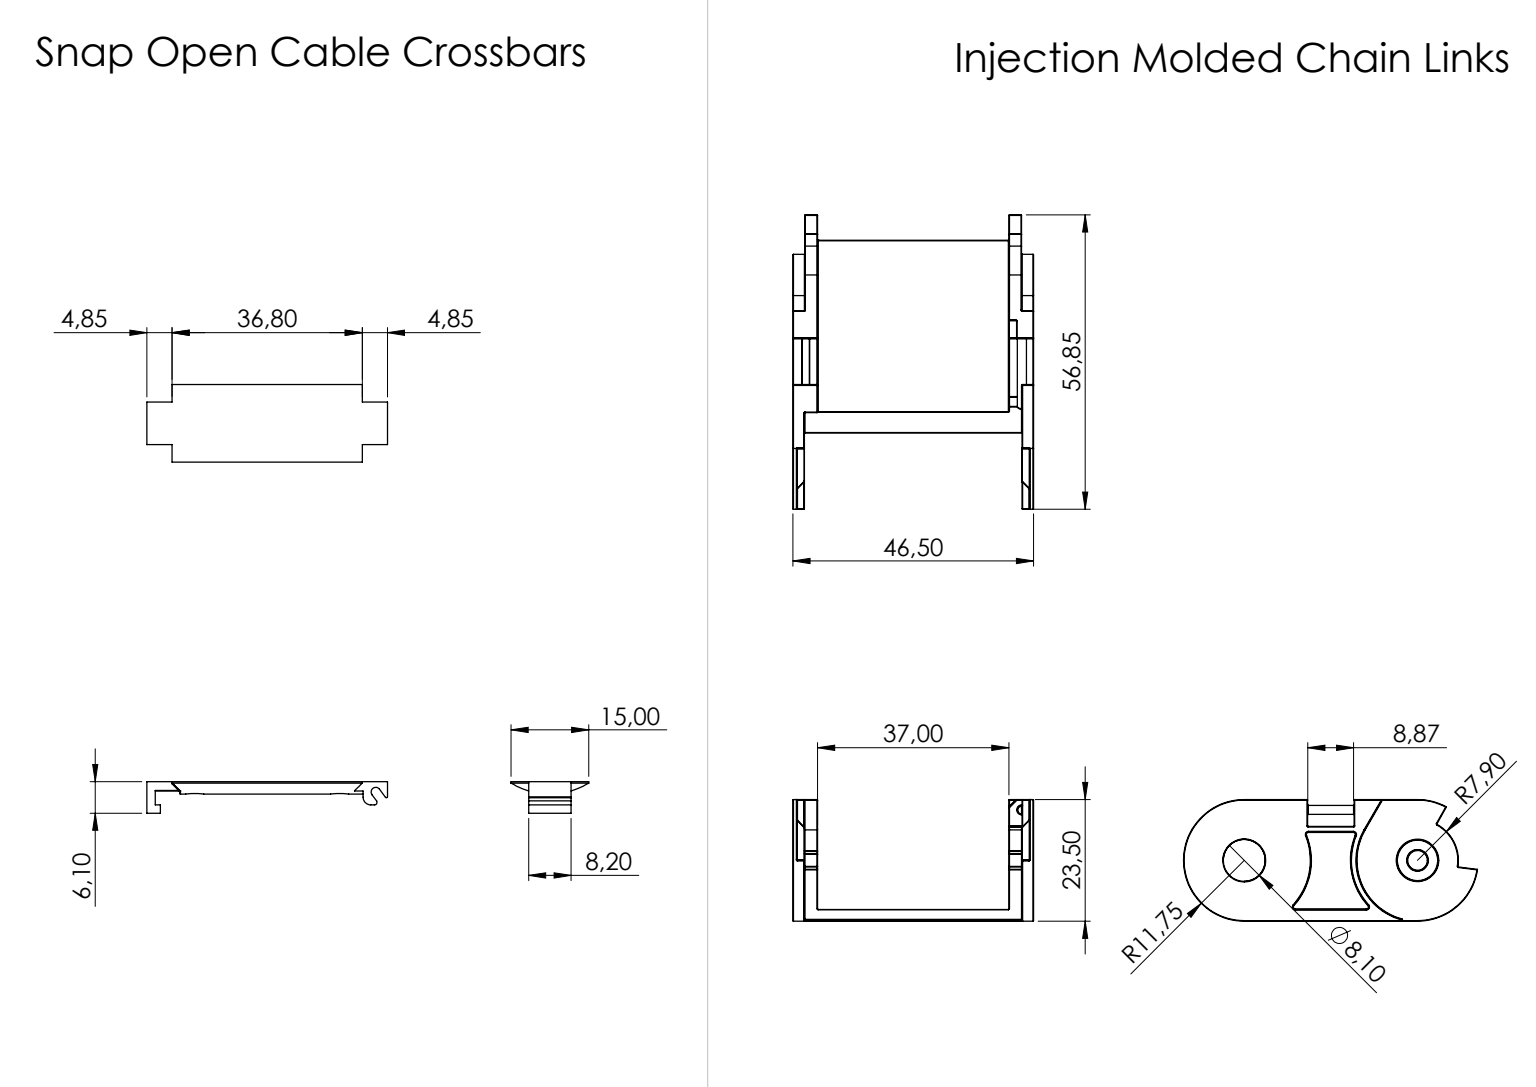
ISO-10303-21;
HEADER;
FILE_DESCRIPTION (('STEP AP214'),
    '1' );
FILE_NAME ('Injection Molded Chain Links.step',
    '2026-10-08T22:59:04',
    ( '' ),
    ( '' ),
    'SwSTEP 2.0',
    'SolidWorks 2020',
    '' );
FILE_SCHEMA (( 'AUTOMOTIVE_DESIGN' ));
ENDSEC;

DATA;
#14=ORIENTED_EDGE ( 'NONE', *, *, #107088, .T. ) ;
#39=LINE ( 'NONE', #62597, #48246 ) ;
#42=CARTESIAN_POINT ( 'NONE',  ( -20.94999999999999929, 0.000000000000000000, -7.900000000000000355 ) ) ;
#67=CARTESIAN_POINT ( 'NONE',  ( -23.15000000000000213, 0.000000000000000000, -4.149999999999999467 ) ) ;
#104=VECTOR ( 'NONE', #151138, 1000.000000000000000 ) ;
#105=ORIENTED_EDGE ( 'NONE', *, *, #252643, .T. ) ;
#109=VERTEX_POINT ( 'NONE', #88531 ) ;
#166=DIRECTION ( 'NONE',  ( -2.952720810173289112E-16, 1.000000000000000000, 0.000000000000000000 ) ) ;
#216=FACE_OUTER_BOUND ( 'NONE', #240838, .T. ) ;
#242=DIRECTION ( 'NONE',  ( 0.000000000000000000, 0.1568667991644863147, -0.9876197685951252359 ) ) ;
#257=CARTESIAN_POINT ( 'NONE',  ( -21.05000000000000071, 0.000000000000000000, -33.50000000000000000 ) ) ;
#265=DIRECTION ( 'NONE',  ( 1.000000000000000000, 1.836970198721029934E-16, 0.000000000000000000 ) ) ;
#269=TOROIDAL_SURFACE ( 'NONE', #212681, 0.2000000000000000111, 0.1000000000000000056 ) ;
#310=CARTESIAN_POINT ( 'NONE',  ( -18.50000000000000000, 9.350000000000001421, -21.35000000000000142 ) ) ;
#321=ORIENTED_EDGE ( 'NONE', *, *, #151126, .F. ) ;
#334=ORIENTED_EDGE ( 'NONE', *, *, #211457, .T. ) ;
#336=CARTESIAN_POINT ( 'NONE',  ( -20.94999027547553894, 10.29326151434211489, -38.95928225104149334 ) ) ;
#345=ORIENTED_EDGE ( 'NONE', *, *, #216352, .F. ) ;
#347=DIRECTION ( 'NONE',  ( 0.000000000000000000, -1.000000000000000000, 0.000000000000000000 ) ) ;
#349=CIRCLE ( 'NONE', #121198, 0.1000000000000000472 ) ;
#354=CIRCLE ( 'NONE', #158793, 0.09999999999999939493 ) ;
#359=AXIS2_PLACEMENT_3D ( 'NONE', #100272, #179854, #1176 ) ;
#378=FACE_OUTER_BOUND ( 'NONE', #36021, .T. ) ;
#380=ORIENTED_EDGE ( 'NONE', *, *, #23400, .F. ) ;
#389=EDGE_LOOP ( 'NONE', ( #34523, #210444, #11516, #231770, #22823, #35860, #120111, #57918, #85074, #11479, #66670, #27843 ) ) ;
#407=VECTOR ( 'NONE', #248788, 1000.000000000000000 ) ;
#409=AXIS2_PLACEMENT_3D ( 'NONE', #159903, #62072, #196433 ) ;
#440=CARTESIAN_POINT ( 'NONE',  ( -23.15000000000000213, 11.75000000000000355, -26.65839931010294350 ) ) ;
#454=DIRECTION ( 'NONE',  ( 0.000000000000000000, 0.000000000000000000, -1.000000000000000000 ) ) ;
#456=SPHERICAL_SURFACE ( 'NONE', #94402, 0.1000000000000000056 ) ;
#465=ORIENTED_EDGE ( 'NONE', *, *, #48822, .T. ) ;
#565=EDGE_CURVE ( 'NONE', #186188, #257228, #38296, .T. ) ;
#572=DIRECTION ( 'NONE',  ( 0.000000000000000000, -1.000000000000000000, 0.000000000000000000 ) ) ;
#581=LINE ( 'NONE', #39765, #75360 ) ;
#585=DIRECTION ( 'NONE',  ( 0.000000000000000000, 0.000000000000000000, -1.000000000000000000 ) ) ;
#587=ORIENTED_EDGE ( 'NONE', *, *, #178313, .F. ) ;
#626=ORIENTED_EDGE ( 'NONE', *, *, #237164, .T. ) ;
#649=DIRECTION ( 'NONE',  ( 0.000000000000000000, -0.6728971962616965286, 0.7397360091702632756 ) ) ;
#664=AXIS2_PLACEMENT_3D ( 'NONE', #248100, #70784, #68187 ) ;
#669=AXIS2_PLACEMENT_3D ( 'NONE', #62579, #85950, #142101 ) ;
#683=ORIENTED_EDGE ( 'NONE', *, *, #92102, .F. ) ;
#694=TOROIDAL_SURFACE ( 'NONE', #134002, 0.2000000000000000111, 0.1000000000000000056 ) ;
#747=CYLINDRICAL_SURFACE ( 'NONE', #257067, 0.5000000000000004441 ) ;
#757=EDGE_CURVE ( 'NONE', #213598, #47066, #138218, .T. ) ;
#764=CIRCLE ( 'NONE', #146531, 0.09999999999999949207 ) ;
#776=ADVANCED_FACE ( 'NONE', ( #218436 ), #241868, .T. ) ;
#836=ORIENTED_EDGE ( 'NONE', *, *, #101044, .T. ) ;
#847=TOROIDAL_SURFACE ( 'NONE', #100785, 4.099999999999999645, 0.1000000000000000056 ) ;
#873=CARTESIAN_POINT ( 'NONE',  ( -18.59999999999999787, 7.021664781900089913, -37.13356540189729316 ) ) ;
#878=DIRECTION ( 'NONE',  ( 0.000000000000000000, 0.000000000000000000, -1.000000000000000000 ) ) ;
#910=DIRECTION ( 'NONE',  ( 0.000000000000000000, 0.000000000000000000, -1.000000000000000000 ) ) ;
#939=CARTESIAN_POINT ( 'NONE',  ( 21.05000000000000071, -0.08559286336224566916, 6.413662734869540749 ) ) ;
#953=CARTESIAN_POINT ( 'NONE',  ( 22.40000000000010516, -9.465541304798784944E-13, 11.75043289245892808 ) ) ;
#960=CARTESIAN_POINT ( 'NONE',  ( -20.85000000000000142, 7.021664781900089913, -37.33356540189728889 ) ) ;
#977=ADVANCED_FACE ( 'NONE', ( #13240 ), #152767, .T. ) ;
#1009=EDGE_CURVE ( 'NONE', #228001, #178016, #16977, .T. ) ;
#1021=AXIS2_PLACEMENT_3D ( 'NONE', #24358, #201685, #107719 ) ;
#1027=DIRECTION ( 'NONE',  ( 0.000000000000000000, 0.9654727137038715545, 0.2605042016806676242 ) ) ;
#1041=ORIENTED_EDGE ( 'NONE', *, *, #205494, .F. ) ;
#1047=ORIENTED_EDGE ( 'NONE', *, *, #175147, .T. ) ;
#1094=FACE_OUTER_BOUND ( 'NONE', #108621, .T. ) ;
#1123=ORIENTED_EDGE ( 'NONE', *, *, #146803, .T. ) ;
#1147=CARTESIAN_POINT ( 'NONE',  ( 20.96937028524355640, 10.62446937162667737, -7.491426101169610163 ) ) ;
#1157=CARTESIAN_POINT ( 'NONE',  ( 23.14999999999999858, 0.000000000000000000, -33.50000000000000000 ) ) ;
#1160=CARTESIAN_POINT ( 'NONE',  ( 20.94999999999999929, 0.000000000000000000, -12.87500000000000000 ) ) ;
#1175=CARTESIAN_POINT ( 'NONE',  ( -23.25000000000000000, -11.75000000000000000, 3.469446951953614189E-15 ) ) ;
#1176=DIRECTION ( 'NONE',  ( -3.265361837132813093E-16, 1.000000000000000000, 0.000000000000000000 ) ) ;
#1186=CARTESIAN_POINT ( 'NONE',  ( -23.15000000000000213, 0.000000000000000000, 0.000000000000000000 ) ) ;
#1240=DIRECTION ( 'NONE',  ( 1.000000000000000000, 0.000000000000000000, 0.000000000000000000 ) ) ;
#1291=DIRECTION ( 'NONE',  ( 0.000000000000000000, 0.000000000000000000, -1.000000000000000000 ) ) ;
#1349=ADVANCED_FACE ( 'NONE', ( #250241 ), #148585, .T. ) ;
#1357=DIRECTION ( 'NONE',  ( 1.000000000000000000, -7.304098846218135653E-16, -2.111765289898286048E-31 ) ) ;
#1367=ORIENTED_EDGE ( 'NONE', *, *, #19245, .F. ) ;
#1370=DIRECTION ( 'NONE',  ( -1.000000000000000000, 7.304098846218135653E-16, 0.000000000000000000 ) ) ;
#1386=ORIENTED_EDGE ( 'NONE', *, *, #239545, .T. ) ;
#1410=ORIENTED_EDGE ( 'NONE', *, *, #124135, .T. ) ;
#1416=EDGE_CURVE ( 'NONE', #106998, #147671, #205037, .T. ) ;
#1470=DIRECTION ( 'NONE',  ( 0.000000000000000000, 0.000000000000000000, -1.000000000000000000 ) ) ;
#1477=EDGE_CURVE ( 'NONE', #5738, #125216, #26199, .T. ) ;
#1493=DIRECTION ( 'NONE',  ( -1.000000000000000000, 7.304098846218134667E-16, 2.111765289898285610E-31 ) ) ;
#1514=AXIS2_PLACEMENT_3D ( 'NONE', #216703, #117607, #38090 ) ;
#1562=EDGE_LOOP ( 'NONE', ( #208368, #145962, #52787, #187592 ) ) ;
#1576=ORIENTED_EDGE ( 'NONE', *, *, #142962, .T. ) ;
#1578=CIRCLE ( 'NONE', #80675, 0.1999999999999987899 ) ;
#1619=CARTESIAN_POINT ( 'NONE',  ( 23.14999999999999858, 11.65000000000000746, -26.48519422934606027 ) ) ;
#1674=VERTEX_POINT ( 'NONE', #171707 ) ;
#1764=AXIS2_PLACEMENT_3D ( 'NONE', #228855, #129746, #163748 ) ;
#1770=DIRECTION ( 'NONE',  ( 0.000000000000000000, 0.000000000000000000, -1.000000000000000000 ) ) ;
#1789=CARTESIAN_POINT ( 'NONE',  ( -18.51697539158856998, 10.31565961586830227, -39.03641941191784070 ) ) ;
#1800=DIRECTION ( 'NONE',  ( 1.000000000000000000, 0.000000000000000000, 0.000000000000000000 ) ) ;
#1812=DIRECTION ( 'NONE',  ( 0.000000000000000000, -0.9654727137038715545, 0.2605042016806676242 ) ) ;
#1823=CARTESIAN_POINT ( 'NONE',  ( 21.05000000000000071, 11.60000000000000675, -26.57179676972450011 ) ) ;
#1903=AXIS2_PLACEMENT_3D ( 'NONE', #254078, #75484, #96279 ) ;
#1923=ORIENTED_EDGE ( 'NONE', *, *, #127687, .F. ) ;
#1932=CARTESIAN_POINT ( 'NONE',  ( 18.50000972452444969, 10.29326151434227121, -38.95928225104144360 ) ) ;
#1934=CARTESIAN_POINT ( 'NONE',  ( 18.59999999999999787, -1.835859311443637010, -45.00443916879852679 ) ) ;
#1941=DIRECTION ( 'NONE',  ( -1.000000000000000000, -2.952720810173289112E-16, 0.000000000000000000 ) ) ;
#1958=DIRECTION ( 'NONE',  ( -3.469446951953614189E-14, 0.000000000000000000, 1.000000000000000000 ) ) ;
#2001=CYLINDRICAL_SURFACE ( 'NONE', #44834, 0.1000000000000000611 ) ;
#2013=AXIS2_PLACEMENT_3D ( 'NONE', #234226, #54301, #34786 ) ;
#2053=ORIENTED_EDGE ( 'NONE', *, *, #23400, .T. ) ;
#2055=AXIS2_PLACEMENT_3D ( 'NONE', #151383, #191803, #135636 ) ;
#2079=LINE ( 'NONE', #161180, #97613 ) ;
#2106=ORIENTED_EDGE ( 'NONE', *, *, #177693, .F. ) ;
#2112=CIRCLE ( 'NONE', #185298, 0.09999999999999892308 ) ;
#2119=ORIENTED_EDGE ( 'NONE', *, *, #28206, .T. ) ;
#2143=AXIS2_PLACEMENT_3D ( 'NONE', #50735, #208578, #170767 ) ;
#2157=DIRECTION ( 'NONE',  ( 0.000000000000000000, -0.4930308989875248349, -0.8700118002898312719 ) ) ;
#2178=AXIS2_PLACEMENT_3D ( 'NONE', #78745, #134856, #20087 ) ;
#2185=CIRCLE ( 'NONE', #147950, 0.5000000000000022204 ) ;
#2200=ORIENTED_EDGE ( 'NONE', *, *, #62626, .F. ) ;
#2208=DIRECTION ( 'NONE',  ( -1.000000000000000000, 0.000000000000000000, 0.000000000000000000 ) ) ;
#2227=CARTESIAN_POINT ( 'NONE',  ( 21.05000000000000071, -11.64999999999999147, -30.50000000000000000 ) ) ;
#2270=FACE_OUTER_BOUND ( 'NONE', #139592, .T. ) ;
#2308=ADVANCED_FACE ( 'NONE', ( #245479 ), #47239, .T. ) ;
#2323=FACE_OUTER_BOUND ( 'NONE', #221063, .T. ) ;
#2327=DIRECTION ( 'NONE',  ( 0.000000000000000000, 0.2605042016806672911, -0.9654727137038716656 ) ) ;
#2356=CARTESIAN_POINT ( 'NONE',  ( 18.59999999999999076, 11.75000000000000355, -8.099999999999999645 ) ) ;
#2373=ORIENTED_EDGE ( 'NONE', *, *, #116759, .T. ) ;
#2401=AXIS2_PLACEMENT_3D ( 'NONE', #20596, #4830, #81791 ) ;
#2406=ORIENTED_EDGE ( 'NONE', *, *, #176143, .F. ) ;
#2425=AXIS2_PLACEMENT_3D ( 'NONE', #153513, #135160, #16531 ) ;
#2438=CARTESIAN_POINT ( 'NONE',  ( 20.41140022480491467, 10.41043084240188854, -7.615001303634437058 ) ) ;
#2449=DIRECTION ( 'NONE',  ( 0.000000000000000000, -1.000000000000000000, 0.000000000000000000 ) ) ;
#2462=VECTOR ( 'NONE', #109339, 999.9999999999998863 ) ;
#2464=CIRCLE ( 'NONE', #48263, 0.1000000000000006578 ) ;
#2468=DIRECTION ( 'NONE',  ( 1.000000000000000000, 0.000000000000000000, -0.000000000000000000 ) ) ;
#2471=CARTESIAN_POINT ( 'NONE',  ( 23.14999999999999858, 5.599999999999996980, -21.09473398108690390 ) ) ;
#2481=CARTESIAN_POINT ( 'NONE',  ( -23.25000000000000000, 6.933893972126341509, -37.28564583437357527 ) ) ;
#2507=CARTESIAN_POINT ( 'NONE',  ( -20.85000000000000142, -1.835859311443637010, -45.00443916879852679 ) ) ;
#2524=CARTESIAN_POINT ( 'NONE',  ( 22.00356870141732912, 7.254242362486300166, -3.773983934443023074E-12 ) ) ;
#2532=AXIS2_PLACEMENT_3D ( 'NONE', #196465, #218584, #174399 ) ;
#2536=CARTESIAN_POINT ( 'NONE',  ( -18.59999999999999787, 9.350000000000001421, -21.25000000000000000 ) ) ;
#2539=ADVANCED_FACE ( 'NONE', ( #24724 ), #47377, .T. ) ;
#2543=DIRECTION ( 'NONE',  ( -1.000000000000000000, -0.000000000000000000, -0.000000000000000000 ) ) ;
#2622=CARTESIAN_POINT ( 'NONE',  ( -18.59999999999999787, -1.164121893241208960, -41.41484808557160591 ) ) ;
#2656=ORIENTED_EDGE ( 'NONE', *, *, #25519, .F. ) ;
#2661=LINE ( 'NONE', #164332, #59484 ) ;
#2686=AXIS2_PLACEMENT_3D ( 'NONE', #214499, #68931, #227984 ) ;
#2687=CARTESIAN_POINT ( 'NONE',  ( -20.85000000000000142, -1.835859311443637010, -45.00443916879852679 ) ) ;
#2688=CIRCLE ( 'NONE', #231670, 0.1999999999999987899 ) ;
#2693=ORIENTED_EDGE ( 'NONE', *, *, #252232, .F. ) ;
#2720=ORIENTED_EDGE ( 'NONE', *, *, #35424, .T. ) ;
#2730=DIRECTION ( 'NONE',  ( -0.7071067811865475727, -0.7071067811865475727, 0.000000000000000000 ) ) ;
#2734=CIRCLE ( 'NONE', #31990, 11.75000000000000000 ) ;
#2746=DIRECTION ( 'NONE',  ( 0.000000000000000000, 0.1575844902526727098, 0.9875055080513754913 ) ) ;
#2776=CARTESIAN_POINT ( 'NONE',  ( -21.05000000000000071, 1.261786168565025568, -8.086498963545480478 ) ) ;
#2804=EDGE_CURVE ( 'NONE', #58858, #117566, #146462, .T. ) ;
#2815=AXIS2_PLACEMENT_3D ( 'NONE', #94429, #119149, #18750 ) ;
#2824=DIRECTION ( 'NONE',  ( 1.000000000000000000, 0.000000000000000000, -0.000000000000000000 ) ) ;
#2856=DIRECTION ( 'NONE',  ( 0.000000000000000000, 0.9908441862701596881, 0.1350103645451904977 ) ) ;
#2868=AXIS2_PLACEMENT_3D ( 'NONE', #237182, #175947, #32601 ) ;
#2894=EDGE_CURVE ( 'NONE', #117327, #96622, #2079, .T. ) ;
#2897=ORIENTED_EDGE ( 'NONE', *, *, #128023, .F. ) ;
#2900=AXIS2_PLACEMENT_3D ( 'NONE', #201147, #143739, #240291 ) ;
#2913=VECTOR ( 'NONE', #172553, 1000.000000000000000 ) ;
#2958=DIRECTION ( 'NONE',  ( 0.000000000000000000, -0.1298341882520022694, -0.9915357197604853789 ) ) ;
#2977=AXIS2_PLACEMENT_3D ( 'NONE', #253000, #74412, #122498 ) ;
#2980=CIRCLE ( 'NONE', #252784, 0.09999999999999949207 ) ;
#3000=ORIENTED_EDGE ( 'NONE', *, *, #195095, .F. ) ;
#3012=ORIENTED_EDGE ( 'NONE', *, *, #238285, .F. ) ;
#3023=EDGE_CURVE ( 'NONE', #205304, #197965, #251765, .T. ) ;
#3040=CARTESIAN_POINT ( 'NONE',  ( -22.39999999999999858, 7.790779598373403836, 0.09999999999999939493 ) ) ;
#3043=CARTESIAN_POINT ( 'NONE',  ( 23.14999999999998437, 0.000000000000000000, 0.000000000000000000 ) ) ;
#3044=VERTEX_POINT ( 'NONE', #124619 ) ;
#3045=( LENGTH_UNIT ( ) NAMED_UNIT ( * ) SI_UNIT ( .MILLI., .METRE. ) );
#3067=CARTESIAN_POINT ( 'NONE',  ( 23.15000000000000213, -11.48912529307605546, -30.39999999999999503 ) ) ;
#3079=ORIENTED_EDGE ( 'NONE', *, *, #16516, .T. ) ;
#3101=DIRECTION ( 'NONE',  ( 1.000000000000000000, 0.000000000000000000, 0.000000000000000000 ) ) ;
#3137=CARTESIAN_POINT ( 'NONE',  ( -21.05000000000000071, -11.65000000000000036, 3.469446951953614189E-15 ) ) ;
#3147=FACE_OUTER_BOUND ( 'NONE', #106294, .T. ) ;
#3157=AXIS2_PLACEMENT_3D ( 'NONE', #39913, #180686, #43735 ) ;
#3158=VERTEX_POINT ( 'NONE', #133592 ) ;
#3194=AXIS2_PLACEMENT_3D ( 'NONE', #216657, #253210, #96674 ) ;
#3211=AXIS2_PLACEMENT_3D ( 'NONE', #225352, #131399, #89696 ) ;
#3226=DIRECTION ( 'NONE',  ( 0.000000000000000000, 0.000000000000000000, -1.000000000000000000 ) ) ;
#3228=FACE_OUTER_BOUND ( 'NONE', #214729, .T. ) ;
#3249=DIRECTION ( 'NONE',  ( 0.000000000000000000, -0.4999999999999799605, 0.8660254037844502539 ) ) ;
#3275=AXIS2_PLACEMENT_3D ( 'NONE', #31311, #49554, #73002 ) ;
#3287=CARTESIAN_POINT ( 'NONE',  ( -23.25000000000000000, -11.75000000000000000, 11.75000000000000000 ) ) ;
#3290=CARTESIAN_POINT ( 'NONE',  ( -23.25000000000000000, 0.000000000000000000, 0.000000000000000000 ) ) ;
#3294=ORIENTED_EDGE ( 'NONE', *, *, #79730, .F. ) ;
#3301=FACE_OUTER_BOUND ( 'NONE', #12226, .T. ) ;
#3327=CARTESIAN_POINT ( 'NONE',  ( -23.25000000000000000, 4.250000000000000000, -12.15000000000000391 ) ) ;
#3345=EDGE_LOOP ( 'NONE', ( #239006, #182794, #63827, #133263 ) ) ;
#3364=FACE_OUTER_BOUND ( 'NONE', #36710, .T. ) ;
#3402=EDGE_CURVE ( 'NONE', #83068, #179010, #22840, .T. ) ;
#3423=ORIENTED_EDGE ( 'NONE', *, *, #134881, .T. ) ;
#3447=DIRECTION ( 'NONE',  ( -0.000000000000000000, -0.000000000000000000, -1.000000000000000000 ) ) ;
#3477=CYLINDRICAL_SURFACE ( 'NONE', #1021, 0.09999999999999939493 ) ;
#3478=CARTESIAN_POINT ( 'NONE',  ( 22.49999999999999645, 11.64976291803192154, 0.08880997638692984808 ) ) ;
#3488=ORIENTED_EDGE ( 'NONE', *, *, #212736, .T. ) ;
#3504=CARTESIAN_POINT ( 'NONE',  ( 18.44444291854881968, -9.490101180943229409, -40.12890396489097355 ) ) ;
#3514=EDGE_CURVE ( 'NONE', #51281, #78587, #255988, .T. ) ;
#3557=CARTESIAN_POINT ( 'NONE',  ( -20.94999999999999929, 0.000000000000000000, -29.50000000000000355 ) ) ;
#3561=AXIS2_PLACEMENT_3D ( 'NONE', #138729, #236573, #1812 ) ;
#3582=CARTESIAN_POINT ( 'NONE',  ( -21.05439746398122836, 11.74999999999999645, -6.989916487484737928 ) ) ;
#3591=FACE_OUTER_BOUND ( 'NONE', #215374, .T. ) ;
#3594=ORIENTED_EDGE ( 'NONE', *, *, #227408, .F. ) ;
#3602=DIRECTION ( 'NONE',  ( 0.000000000000000000, 0.9915357197604882655, -0.1298341882519791490 ) ) ;
#3628=AXIS2_PLACEMENT_3D ( 'NONE', #8302, #107375, #206488 ) ;
#3631=VERTEX_POINT ( 'NONE', #104098 ) ;
#3645=EDGE_CURVE ( 'NONE', #255042, #137088, #210458, .T. ) ;
#3650=DIRECTION ( 'NONE',  ( -3.469446951953605354E-14, 1.000000000000000000, 0.000000000000000000 ) ) ;
#3661=ORIENTED_EDGE ( 'NONE', *, *, #115872, .F. ) ;
#3664=( BOUNDED_SURFACE ( )  B_SPLINE_SURFACE ( 3, 2, ( 
 ( #19306, #57123, #238346 ),
 ( #222611, #68705, #205626 ),
 ( #204345, #146932, #4840 ),
 ( #225181, #84353, #3582 ),
 ( #43998, #23180, #166547 ),
 ( #148232, #63553, #246062 ) ),
 .UNSPECIFIED., .F., .F., .F. ) 
 B_SPLINE_SURFACE_WITH_KNOTS ( ( 4, 2, 4 ),
 ( 3, 3 ),
 ( 1.570796326794895448, 2.356194490192343505, 3.141592653589791784 ),
 ( 0.000000000000000000, 1.000000000000000000 ),
 .UNSPECIFIED. ) 
 GEOMETRIC_REPRESENTATION_ITEM ( )  RATIONAL_B_SPLINE_SURFACE ( (
 ( 1.000000000000000000, 0.7071067811865414665, 1.000000000000000000),
 ( 1.000000000000000000, 0.6611148371779385080, 1.000000000000000000),
 ( 1.000000000000000000, 0.6092287576695514240, 1.000000000000000000),
 ( 1.000000000000000000, 0.5278258667058023379, 1.000000000000000000),
 ( 1.000000000000000000, 0.4993418825334033362, 1.000000000000000000),
 ( 1.000000000000000000, 0.4999999999999952816, 1.000000000000000000) ) ) 
 REPRESENTATION_ITEM ( '' )  SURFACE ( )  );
#3687=CARTESIAN_POINT ( 'NONE',  ( -23.15000000000000213, 11.65000000000000036, -21.25000000000000000 ) ) ;
#3697=AXIS2_PLACEMENT_3D ( 'NONE', #243963, #192993, #251669 ) ;
#3704=ORIENTED_EDGE ( 'NONE', *, *, #145562, .F. ) ;
#3711=DIRECTION ( 'NONE',  ( 0.000000000000000000, 1.000000000000000000, 0.000000000000000000 ) ) ;
#3741=EDGE_CURVE ( 'NONE', #199662, #64464, #206355, .T. ) ;
#3789=EDGE_LOOP ( 'NONE', ( #234210, #119558, #13967, #16047 ) ) ;
#3815=DIRECTION ( 'NONE',  ( -1.000000000000000000, 0.000000000000000000, 0.000000000000000000 ) ) ;
#3824=CARTESIAN_POINT ( 'NONE',  ( 21.07094088545303734, 6.320167221916491052, 0.09889370255222132422 ) ) ;
#3829=DIRECTION ( 'NONE',  ( -0.000000000000000000, 0.8660254037844411501, 0.4999999999999956701 ) ) ;
#3830=DIRECTION ( 'NONE',  ( 1.000000000000000000, 0.000000000000000000, 0.000000000000000000 ) ) ;
#3841=CARTESIAN_POINT ( 'NONE',  ( -21.14999999999999858, 6.540656951701240729, 0.000000000000000000 ) ) ;
#3844=DIRECTION ( 'NONE',  ( 0.000000000000000000, 0.000000000000000000, -1.000000000000000000 ) ) ;
#3878=CARTESIAN_POINT ( 'NONE',  ( -22.39999999999999858, 11.65000000000000036, -3.469446951953614189E-15 ) ) ;
#3883=AXIS2_PLACEMENT_3D ( 'NONE', #159584, #1770, #138685 ) ;
#3889=DIRECTION ( 'NONE',  ( 2.710505431213777355E-16, -1.000000000000000000, 0.000000000000000000 ) ) ;
#3936=ORIENTED_EDGE ( 'NONE', *, *, #105558, .T. ) ;
#3959=ORIENTED_EDGE ( 'NONE', *, *, #89948, .T. ) ;
#3973=DIRECTION ( 'NONE',  ( 0.000000000000000000, 0.4999999999999799605, -0.8660254037844502539 ) ) ;
#3996=ORIENTED_EDGE ( 'NONE', *, *, #128666, .F. ) ;
#3999=EDGE_CURVE ( 'NONE', #43854, #174426, #199068, .T. ) ;
#4007=AXIS2_PLACEMENT_3D ( 'NONE', #88671, #45719, #148692 ) ;
#4052=CARTESIAN_POINT ( 'NONE',  ( 18.49999999999999645, -9.419209763409250868, -7.247769462758938630 ) ) ;
#4075=ORIENTED_EDGE ( 'NONE', *, *, #146740, .T. ) ;
#4081=TOROIDAL_SURFACE ( 'NONE', #249613, 11.65000000000000036, 0.1000000000000000056 ) ;
#4082=AXIS2_PLACEMENT_3D ( 'NONE', #103246, #4162, #197548 ) ;
#4094=CARTESIAN_POINT ( 'NONE',  ( -20.94999999999999929, 11.64999999999999680, -26.71613433702190576 ) ) ;
#4098=VERTEX_POINT ( 'NONE', #98635 ) ;
#4103=CARTESIAN_POINT ( 'NONE',  ( 21.12230431290518951, 0.005209851689007149664, 6.457566653293008052 ) ) ;
#4162=DIRECTION ( 'NONE',  ( 1.000000000000000000, -0.000000000000000000, -0.000000000000000000 ) ) ;
#4187=CARTESIAN_POINT ( 'NONE',  ( -22.39999999999999858, -0.09999999999999939493, 11.64957080754479968 ) ) ;
#4217=CARTESIAN_POINT ( 'NONE',  ( -23.25000000000000000, -0.1008583690987122083, 11.74956712348939192 ) ) ;
#4246=ORIENTED_EDGE ( 'NONE', *, *, #174461, .T. ) ;
#4280=ORIENTED_EDGE ( 'NONE', *, *, #147191, .T. ) ;
#4290=ORIENTED_EDGE ( 'NONE', *, *, #18183, .F. ) ;
#4298=ORIENTED_EDGE ( 'NONE', *, *, #160551, .T. ) ;
#4300=AXIS2_PLACEMENT_3D ( 'NONE', #149727, #72766, #250086 ) ;
#4309=DIRECTION ( 'NONE',  ( 1.000000000000000000, 0.000000000000000000, -0.000000000000000000 ) ) ;
#4323=AXIS2_PLACEMENT_3D ( 'NONE', #118176, #97282, #184241 ) ;
#4329=DIRECTION ( 'NONE',  ( 0.000000000000000000, -1.000000000000000000, 0.000000000000000000 ) ) ;
#4330=ORIENTED_EDGE ( 'NONE', *, *, #17648, .F. ) ;
#4353=DIRECTION ( 'NONE',  ( 1.301042606982683418E-14, -0.8660254037844330455, 0.5000000000000096589 ) ) ;
#4416=VERTEX_POINT ( 'NONE', #39711 ) ;
#4476=DIRECTION ( 'NONE',  ( 0.000000000000000000, 0.000000000000000000, -1.000000000000000000 ) ) ;
#4477=CARTESIAN_POINT ( 'NONE',  ( 18.49999999999999645, -1.835341550224411922, -11.55515129256297868 ) ) ;
#4481=ORIENTED_EDGE ( 'NONE', *, *, #28307, .F. ) ;
#4497=EDGE_CURVE ( 'NONE', #223333, #104459, #188153, .T. ) ;
#4508=VERTEX_POINT ( 'NONE', #25272 ) ;
#4546=CARTESIAN_POINT ( 'NONE',  ( 20.94999999999999929, 0.000000000000000000, 0.000000000000000000 ) ) ;
#4608=EDGE_CURVE ( 'NONE', #13885, #18401, #253276, .T. ) ;
#4613=ORIENTED_EDGE ( 'NONE', *, *, #172783, .T. ) ;
#4645=ORIENTED_EDGE ( 'NONE', *, *, #42670, .T. ) ;
#4660=DIRECTION ( 'NONE',  ( 0.000000000000000000, -0.000000000000000000, -1.000000000000000000 ) ) ;
#4732=DIRECTION ( 'NONE',  ( 0.000000000000000000, -1.000000000000000000, 0.000000000000000000 ) ) ;
#4734=VERTEX_POINT ( 'NONE', #142315 ) ;
#4766=CARTESIAN_POINT ( 'NONE',  ( -18.51555513499604899, -9.352657054504497580, -7.195169895697221207 ) ) ;
#4824=DIRECTION ( 'NONE',  ( 0.000000000000000000, -0.9893560106964500722, 0.1455152366551550613 ) ) ;
#4830=DIRECTION ( 'NONE',  ( -5.603264701231743991E-32, 1.897661533703520143E-16, -1.000000000000000000 ) ) ;
#4840=CARTESIAN_POINT ( 'NONE',  ( -21.12844524849339223, 11.74999999999999645, -6.904413470842653666 ) ) ;
#4849=ORIENTED_EDGE ( 'NONE', *, *, #241298, .T. ) ;
#4884=SPHERICAL_SURFACE ( 'NONE', #33767, 0.1000000000000000056 ) ;
#4890=ORIENTED_EDGE ( 'NONE', *, *, #102475, .T. ) ;
#4892=CARTESIAN_POINT ( 'NONE',  ( 21.03675099975491136, 8.875180032784809825, -12.32554213677804711 ) ) ;
#4898=ORIENTED_EDGE ( 'NONE', *, *, #92333, .T. ) ;
#4918=FACE_OUTER_BOUND ( 'NONE', #132654, .T. ) ;
#4954=VECTOR ( 'NONE', #64817, 1000.000000000000000 ) ;
#4965=DIRECTION ( 'NONE',  ( 0.000000000000000000, 1.000000000000000000, 0.000000000000000000 ) ) ;
#4976=DIRECTION ( 'NONE',  ( 0.000000000000000000, 1.000000000000000000, 2.891205793294679805E-16 ) ) ;
#4979=CIRCLE ( 'NONE', #17474, 0.09999999999999939493 ) ;
#4981=AXIS2_PLACEMENT_3D ( 'NONE', #178018, #257471, #78871 ) ;
#5005=CARTESIAN_POINT ( 'NONE',  ( -23.25000000000000000, -11.48912529307605546, -30.39999999999999858 ) ) ;
#5012=ORIENTED_EDGE ( 'NONE', *, *, #187956, .T. ) ;
#5054=CARTESIAN_POINT ( 'NONE',  ( -18.59999999999999787, 11.64999999999999680, -6.914805770653999595 ) ) ;
#5103=CIRCLE ( 'NONE', #63385, 0.09999999999999939493 ) ;
#5121=ORIENTED_EDGE ( 'NONE', *, *, #73238, .F. ) ;
#5136=EDGE_CURVE ( 'NONE', #32549, #242536, #181169, .T. ) ;
#5150=CARTESIAN_POINT ( 'NONE',  ( 19.97071067695831559, 11.72071067695831914, -24.67625343280356276 ) ) ;
#5182=CARTESIAN_POINT ( 'NONE',  ( 21.12642695952774119, 0.09890328318936439378, 6.375659922035173288 ) ) ;
#5189=DIRECTION ( 'NONE',  ( 0.7071359030027419834, 0.000000000000000000, 0.7070776581709371511 ) ) ;
#5190=ORIENTED_EDGE ( 'NONE', *, *, #234752, .F. ) ;
#5222=VERTEX_POINT ( 'NONE', #122475 ) ;
#5230=DIRECTION ( 'NONE',  ( 0.000000000000000000, 0.000000000000000000, -1.000000000000000000 ) ) ;
#5236=VERTEX_POINT ( 'NONE', #145862 ) ;
#5241=ORIENTED_EDGE ( 'NONE', *, *, #38418, .T. ) ;
#5267=EDGE_CURVE ( 'NONE', #51098, #120640, #224118, .T. ) ;
#5286=AXIS2_PLACEMENT_3D ( 'NONE', #39953, #119475, #99861 ) ;
#5287=ORIENTED_EDGE ( 'NONE', *, *, #238878, .F. ) ;
#5290=EDGE_LOOP ( 'NONE', ( #54995, #145368, #185205, #101216 ) ) ;
#5315=FACE_OUTER_BOUND ( 'NONE', #40208, .T. ) ;
#5318=FACE_OUTER_BOUND ( 'NONE', #251989, .T. ) ;
#5342=SPHERICAL_SURFACE ( 'NONE', #191634, 0.1000000000000000056 ) ;
#5388=EDGE_CURVE ( 'NONE', #251327, #24262, #144137, .T. ) ;
#5406=EDGE_CURVE ( 'NONE', #74587, #77399, #27693, .T. ) ;
#5413=DIRECTION ( 'NONE',  ( 1.000000000000000000, -0.000000000000000000, -0.000000000000000000 ) ) ;
#5431=ORIENTED_EDGE ( 'NONE', *, *, #201112, .T. ) ;
#5447=CARTESIAN_POINT ( 'NONE',  ( -21.05000000000000071, -1.835341550224411922, -11.65515129256297833 ) ) ;
#5453=CARTESIAN_POINT ( 'NONE',  ( -20.85882249326303040, 10.33248238082519066, -39.09484654391314962 ) ) ;
#5463=CARTESIAN_POINT ( 'NONE',  ( 23.15000000000000213, -9.000000000000001776, -9.893969122652443104 ) ) ;
#5469=FACE_OUTER_BOUND ( 'NONE', #199782, .T. ) ;
#5471=ORIENTED_EDGE ( 'NONE', *, *, #188128, .F. ) ;
#5473=DIRECTION ( 'NONE',  ( -1.000000000000000000, -3.265361837132813093E-16, 0.000000000000000000 ) ) ;
#5533=DIRECTION ( 'NONE',  ( -0.000000000000000000, -0.000000000000000000, 1.000000000000000000 ) ) ;
#5538=VECTOR ( 'NONE', #97161, 1000.000000000000000 ) ;
#5540=CIRCLE ( 'NONE', #38903, 11.75000000000000000 ) ;
#5562=FACE_OUTER_BOUND ( 'NONE', #232632, .T. ) ;
#5570=AXIS2_PLACEMENT_3D ( 'NONE', #82463, #165915, #62935 ) ;
#5575=ORIENTED_EDGE ( 'NONE', *, *, #252743, .F. ) ;
#5631=CARTESIAN_POINT ( 'NONE',  ( -18.59999999999999787, 10.33248238082518711, -39.09484654391314962 ) ) ;
#5639=DIRECTION ( 'NONE',  ( 1.000000000000000000, 0.000000000000000000, 0.000000000000000000 ) ) ;
#5650=LINE ( 'NONE', #245587, #121614 ) ;
#5661=DIRECTION ( 'NONE',  ( 0.000000000000000000, 1.000000000000000000, 0.000000000000000000 ) ) ;
#5708=CARTESIAN_POINT ( 'NONE',  ( -23.25000000000000000, -11.65000000000000036, -3.100000000000001865 ) ) ;
#5721=AXIS2_PLACEMENT_3D ( 'NONE', #82782, #162383, #142775 ) ;
#5738=VERTEX_POINT ( 'NONE', #13450 ) ;
#5770=LINE ( 'NONE', #162320, #105725 ) ;
#5774=AXIS2_PLACEMENT_3D ( 'NONE', #63187, #142723, #222246 ) ;
#5781=CARTESIAN_POINT ( 'NONE',  ( 18.57399277249656322, 10.33112638555854268, -39.09012289269746532 ) ) ;
#5788=DIRECTION ( 'NONE',  ( 1.000000000000000000, 0.000000000000000000, 0.000000000000000000 ) ) ;
#5799=DIRECTION ( 'NONE',  ( 0.000000000000000000, 0.000000000000000000, -1.000000000000000000 ) ) ;
#5813=AXIS2_PLACEMENT_3D ( 'NONE', #1619, #57740, #19931 ) ;
#5826=EDGE_CURVE ( 'NONE', #47156, #195886, #250319, .T. ) ;
#5828=EDGE_LOOP ( 'NONE', ( #85955, #132514, #152160, #122344 ) ) ;
#5832=ORIENTED_EDGE ( 'NONE', *, *, #223359, .T. ) ;
#5848=DIRECTION ( 'NONE',  ( 0.000000000000000000, 0.4999999999999966693, -0.8660254037844405950 ) ) ;
#5876=AXIS2_PLACEMENT_3D ( 'NONE', #111557, #192376, #224112 ) ;
#5878=CARTESIAN_POINT ( 'NONE',  ( 23.24999999999999645, 5.599999999999996980, -12.40526601891309788 ) ) ;
#5889=ADVANCED_FACE ( 'NONE', ( #135486 ), #195509, .F. ) ;
#5904=AXIS2_PLACEMENT_3D ( 'NONE', #105179, #107792, #11271 ) ;
#5935=DIRECTION ( 'NONE',  ( 0.000000000000000000, 0.000000000000000000, -1.000000000000000000 ) ) ;
#5950=LINE ( 'NONE', #201602, #14273 ) ;
#5992=ADVANCED_FACE ( 'NONE', ( #92517 ), #212494, .F. ) ;
#6018=DIRECTION ( 'NONE',  ( 0.000000000000000000, 0.000000000000000000, 1.000000000000000000 ) ) ;
#6029=CARTESIAN_POINT ( 'NONE',  ( 21.97500000000000497, 9.749999999999998224, -21.25000000000000000 ) ) ;
#6045=VECTOR ( 'NONE', #249518, 1000.000000000000000 ) ;
#6053=CIRCLE ( 'NONE', #143438, 0.1000000000000028644 ) ;
#6064=CARTESIAN_POINT ( 'NONE',  ( -23.15000000000000213, 4.250000000000000000, -12.25000000000000000 ) ) ;
#6065=DIRECTION ( 'NONE',  ( -0.000000000000000000, 0.000000000000000000, -1.000000000000000000 ) ) ;
#6066=CARTESIAN_POINT ( 'NONE',  ( -18.52186455168988388, -9.481018481442522017, -7.025016477914483914 ) ) ;
#6079=CARTESIAN_POINT ( 'NONE',  ( -23.25000000000000000, -0.09999999999999939493, 11.64957080754479968 ) ) ;
#6108=LINE ( 'NONE', #225148, #116295 ) ;
#6122=CARTESIAN_POINT ( 'NONE',  ( -18.59999999999999787, 1.835341550224411922, -11.55515129256298046 ) ) ;
#6152=DIRECTION ( 'NONE',  ( 1.000000000000000000, 0.000000000000000000, 0.000000000000000000 ) ) ;
#6159=AXIS2_PLACEMENT_3D ( 'NONE', #215329, #154127, #177535 ) ;
#6160=CARTESIAN_POINT ( 'NONE',  ( -18.59999999999999787, -1.835859311443637010, -45.00443916879852679 ) ) ;
#6165=DIRECTION ( 'NONE',  ( 0.000000000000000000, -0.8777080977375132376, 0.4791956752371582251 ) ) ;
#6193=VERTEX_POINT ( 'NONE', #46976 ) ;
#6203=EDGE_CURVE ( 'NONE', #72992, #129969, #28773, .T. ) ;
#6224=ORIENTED_EDGE ( 'NONE', *, *, #16437, .T. ) ;
#6252=CARTESIAN_POINT ( 'NONE',  ( -20.85000000000000142, 10.33248238082519421, -39.09484654391315672 ) ) ;
#6283=FACE_OUTER_BOUND ( 'NONE', #81257, .T. ) ;
#6293=VERTEX_POINT ( 'NONE', #109526 ) ;
#6311=ORIENTED_EDGE ( 'NONE', *, *, #49953, .T. ) ;
#6354=DIRECTION ( 'NONE',  ( 0.000000000000000000, 1.000000000000000000, -6.308085367188393199E-16 ) ) ;
#6362=CIRCLE ( 'NONE', #31358, 0.2000000000000000944 ) ;
#6365=AXIS2_PLACEMENT_3D ( 'NONE', #256007, #39624, #239076 ) ;
#6390=DIRECTION ( 'NONE',  ( 0.000000000000000000, 8.673617379883997607E-15, -1.000000000000000000 ) ) ;
#6393=CARTESIAN_POINT ( 'NONE',  ( -21.05000000000000071, -1.261786168565025568, -8.086498963545480478 ) ) ;
#6399=DIRECTION ( 'NONE',  ( 0.000000000000000000, 0.000000000000000000, -1.000000000000000000 ) ) ;
#6411=CIRCLE ( 'NONE', #102065, 0.09999999999999939493 ) ;
#6421=AXIS2_PLACEMENT_3D ( 'NONE', #127541, #85804, #106667 ) ;
#6457=EDGE_CURVE ( 'NONE', #130735, #141605, #65422, .T. ) ;
#6486=FACE_OUTER_BOUND ( 'NONE', #102106, .T. ) ;
#6514=ORIENTED_EDGE ( 'NONE', *, *, #140101, .F. ) ;
#6525=EDGE_CURVE ( 'NONE', #79894, #139796, #61115, .T. ) ;
#6534=ORIENTED_EDGE ( 'NONE', *, *, #60005, .T. ) ;
#6539=ORIENTED_EDGE ( 'NONE', *, *, #13153, .T. ) ;
#6543=ORIENTED_EDGE ( 'NONE', *, *, #198849, .F. ) ;
#6556=VERTEX_POINT ( 'NONE', #181089 ) ;
#6561=LINE ( 'NONE', #45690, #17779 ) ;
#6569=CARTESIAN_POINT ( 'NONE',  ( 18.59999999999999432, -9.480686695278969012, -40.44111516875785384 ) ) ;
#6629=CARTESIAN_POINT ( 'NONE',  ( -21.04999999999999361, 6.344723404090243157, 0.01471785652417695149 ) ) ;
#6720=DIRECTION ( 'NONE',  ( -0.000000000000000000, 1.265107689135680095E-16, -1.000000000000000000 ) ) ;
#6745=CYLINDRICAL_SURFACE ( 'NONE', #194013, 0.09999999999999939493 ) ;
#6747=CIRCLE ( 'NONE', #31727, 12.87499999999999822 ) ;
#6815=CYLINDRICAL_SURFACE ( 'NONE', #66673, 0.09999999999999939493 ) ;
#6828=ORIENTED_EDGE ( 'NONE', *, *, #188454, .F. ) ;
#6883=PLANE ( 'NONE',  #183581 ) ;
#6892=EDGE_CURVE ( 'NONE', #257228, #71514, #223393, .T. ) ;
#6903=CIRCLE ( 'NONE', #181879, 0.1000000000000028644 ) ;
#6931=DIRECTION ( 'NONE',  ( 0.000000000000000000, 0.000000000000000000, -1.000000000000000000 ) ) ;
#6936=DIRECTION ( 'NONE',  ( 5.421010862427554711E-16, -1.000000000000000000, -3.252606517456533024E-15 ) ) ;
#6961=AXIS2_PLACEMENT_3D ( 'NONE', #185196, #28741, #84773 ) ;
#6976=LINE ( 'NONE', #246865, #66631 ) ;
#6990=EDGE_LOOP ( 'NONE', ( #61919, #4645, #17869, #90204 ) ) ;
#7004=ORIENTED_EDGE ( 'NONE', *, *, #124061, .F. ) ;
#7041=CARTESIAN_POINT ( 'NONE',  ( 18.49999999999999645, 1.866714910057309273, -11.75267524628200633 ) ) ;
#7062=DIRECTION ( 'NONE',  ( 0.000000000000000000, -0.1350103645451904977, 0.9908441862701596881 ) ) ;
#7081=EDGE_LOOP ( 'NONE', ( #137334, #244755, #197345, #78990 ) ) ;
#7102=LINE ( 'NONE', #72239, #98639 ) ;
#7111=DIRECTION ( 'NONE',  ( -1.000000000000000000, 0.000000000000000000, 0.000000000000000000 ) ) ;
#7168=TOROIDAL_SURFACE ( 'NONE', #202997, 7.800000000000000711, 0.1000000000000000056 ) ;
#7213=EDGE_CURVE ( 'NONE', #17135, #257228, #18497, .T. ) ;
#7214=EDGE_CURVE ( 'NONE', #178016, #18401, #152930, .T. ) ;
#7232=VECTOR ( 'NONE', #136462, 1000.000000000000000 ) ;
#7238=CARTESIAN_POINT ( 'NONE',  ( 20.94999999999999574, 1.749999999999999778, -11.66951155790164485 ) ) ;
#7269=CARTESIAN_POINT ( 'NONE',  ( 18.59999999999999432, -1.162701749938009677, -8.099999999999999645 ) ) ;
#7277=CARTESIAN_POINT ( 'NONE',  ( 20.94999999999999574, 10.47338541491290442, -7.578654464248542943 ) ) ;
#7282=CARTESIAN_POINT ( 'NONE',  ( 18.59999999999999076, 10.49142135623730709, -24.85000000000000142 ) ) ;
#7287=AXIS2_PLACEMENT_3D ( 'NONE', #64117, #48391, #67962 ) ;
#7304=AXIS2_PLACEMENT_3D ( 'NONE', #225617, #226931, #207388 ) ;
#7345=CARTESIAN_POINT ( 'NONE',  ( 21.95218792049437795, 7.201507561246661915, 0.09902843979991737822 ) ) ;
#7346=VECTOR ( 'NONE', #50037, 1000.000000000000114 ) ;
#7364=CARTESIAN_POINT ( 'NONE',  ( 18.49505816908823874, -9.437872553211134274, -40.27765720167089114 ) ) ;
#7367=DIRECTION ( 'NONE',  ( -1.000000000000000000, -2.952720810173289112E-16, 0.000000000000000000 ) ) ;
#7376=CARTESIAN_POINT ( 'NONE',  ( 23.14999999999999503, 6.649999999999999467, -21.35000000000000142 ) ) ;
#7382=ADVANCED_FACE ( 'NONE', ( #5315 ), #21091, .F. ) ;
#7411=ADVANCED_FACE ( 'NONE', ( #142284 ), #104421, .T. ) ;
#7416=CARTESIAN_POINT ( 'NONE',  ( -23.25000000000000000, -11.65000000000000036, -30.39999999999999858 ) ) ;
#7470=AXIS2_PLACEMENT_3D ( 'NONE', #79898, #219424, #95634 ) ;
#7482=DIRECTION ( 'NONE',  ( 0.000000000000000000, 1.000000000000000000, -6.308085367188393199E-16 ) ) ;
#7504=CARTESIAN_POINT ( 'NONE',  ( -18.50000000000000000, 11.64999999999999680, -12.14999999999999680 ) ) ;
#7505=AXIS2_PLACEMENT_3D ( 'NONE', #237710, #254659, #136010 ) ;
#7512=AXIS2_PLACEMENT_3D ( 'NONE', #116901, #96038, #196427 ) ;
#7527=EDGE_CURVE ( 'NONE', #56398, #72182, #168325, .T. ) ;
#7559=FACE_OUTER_BOUND ( 'NONE', #55007, .T. ) ;
#7563=( BOUNDED_SURFACE ( )  B_SPLINE_SURFACE ( 3, 2, ( 
 ( #156830, #75978, #79799 ),
 ( #238908, #35600, #175129 ),
 ( #154281, #78530, #236331 ),
 ( #39454, #253319, #116398 ) ),
 .UNSPECIFIED., .F., .F., .F. ) 
 B_SPLINE_SURFACE_WITH_KNOTS ( ( 4, 4 ),
 ( 3, 3 ),
 ( 0.0006461284895273955529, 0.0007503702773985933402 ),
 ( 0.000000000000000000, 1.000000000000000000 ),
 .UNSPECIFIED. ) 
 GEOMETRIC_REPRESENTATION_ITEM ( )  RATIONAL_B_SPLINE_SURFACE ( (
 ( 1.000000000000000000, 0.7071067811865475727, 1.000000000000000000),
 ( 1.000000000000000000, 0.7076476444648740483, 1.000000000000000000),
 ( 1.000000000000000000, 0.7075727925191916956, 1.000000000000000000),
 ( 1.000000000000000000, 0.7071067811865475727, 1.000000000000000000) ) ) 
 REPRESENTATION_ITEM ( '' )  SURFACE ( )  );
#7572=ORIENTED_EDGE ( 'NONE', *, *, #250128, .T. ) ;
#7582=AXIS2_PLACEMENT_3D ( 'NONE', #140304, #159910, #239435 ) ;
#7592=ORIENTED_EDGE ( 'NONE', *, *, #218958, .T. ) ;
#7665=ADVANCED_FACE ( 'NONE', ( #196812 ), #134263, .F. ) ;
#7672=EDGE_CURVE ( 'NONE', #213598, #39469, #11444, .T. ) ;
#7673=CYLINDRICAL_SURFACE ( 'NONE', #113340, 0.09999999999999939493 ) ;
#7687=CIRCLE ( 'NONE', #3561, 0.09999999999999971412 ) ;
#7693=EDGE_CURVE ( 'NONE', #199162, #107823, #57184, .T. ) ;
#7720=ORIENTED_EDGE ( 'NONE', *, *, #122168, .F. ) ;
#7728=DIRECTION ( 'NONE',  ( -1.000000000000000000, 0.000000000000000000, 0.000000000000000000 ) ) ;
#7739=EDGE_LOOP ( 'NONE', ( #132540, #11041, #38240, #23278 ) ) ;
#7751=VERTEX_POINT ( 'NONE', #20777 ) ;
#7760=CARTESIAN_POINT ( 'NONE',  ( 19.99999999738043144, 11.75000000000000888, -24.68717194963242534 ) ) ;
#7791=CARTESIAN_POINT ( 'NONE',  ( -22.59999999999999787, 11.74956712348939192, 0.1008583690987083364 ) ) ;
#7812=ORIENTED_EDGE ( 'NONE', *, *, #204325, .F. ) ;
#7815=AXIS2_PLACEMENT_3D ( 'NONE', #163813, #118600, #45136 ) ;
#7847=LINE ( 'NONE', #245166, #50903 ) ;
#7862=EDGE_CURVE ( 'NONE', #39052, #77399, #198857, .T. ) ;
#7872=DIRECTION ( 'NONE',  ( -0.000000000000000000, 0.8660254037844383745, -0.5000000000000003331 ) ) ;
#7882=ORIENTED_EDGE ( 'NONE', *, *, #25314, .T. ) ;
#7889=LINE ( 'NONE', #87390, #55164 ) ;
#7891=ORIENTED_EDGE ( 'NONE', *, *, #126743, .F. ) ;
#7896=CARTESIAN_POINT ( 'NONE',  ( -18.59999999999999787, 10.33248238082518711, -39.09484654391314962 ) ) ;
#7899=ADVANCED_FACE ( 'NONE', ( #170591 ), #149002, .T. ) ;
#7922=CARTESIAN_POINT ( 'NONE',  ( -21.04999999999999716, 0.09843749999999835965, 6.299230910086880186 ) ) ;
#7965=PLANE ( 'NONE',  #23796 ) ;
#7994=DIRECTION ( 'NONE',  ( -0.000000000000000000, 1.000000000000000000, 0.000000000000000000 ) ) ;
#8004=FACE_OUTER_BOUND ( 'NONE', #18921, .T. ) ;
#8034=AXIS2_PLACEMENT_3D ( 'NONE', #73330, #15921, #253206 ) ;
#8077=AXIS2_PLACEMENT_3D ( 'NONE', #178306, #158746, #79159 ) ;
#8078=EDGE_CURVE ( 'NONE', #15934, #56536, #149189, .T. ) ;
#8113=CIRCLE ( 'NONE', #199669, 0.09999999999999939493 ) ;
#8122=EDGE_LOOP ( 'NONE', ( #26697, #87654, #40215, #11669, #85136, #55965 ) ) ;
#8185=ORIENTED_EDGE ( 'NONE', *, *, #57731, .F. ) ;
#8193=CIRCLE ( 'NONE', #29067, 0.1000000000000002554 ) ;
#8232=CARTESIAN_POINT ( 'NONE',  ( 23.14999999999999858, 3.899999999999999467, -33.50000000000000000 ) ) ;
#8240=DIRECTION ( 'NONE',  ( 1.000000000000000000, -0.000000000000000000, -0.000000000000000000 ) ) ;
#8282=EDGE_LOOP ( 'NONE', ( #25425, #85408, #157565, #183929 ) ) ;
#8296=ORIENTED_EDGE ( 'NONE', *, *, #10518, .T. ) ;
#8302=CARTESIAN_POINT ( 'NONE',  ( 20.94999999999999929, -1.835341550224413698, -11.55515129256298046 ) ) ;
#8315=CARTESIAN_POINT ( 'NONE',  ( 21.05000000000000071, 8.776282895292474961, -12.15000000000000036 ) ) ;
#8325=EDGE_CURVE ( 'NONE', #183282, #144164, #16102, .T. ) ;
#8376=ADVANCED_FACE ( 'NONE', ( #85513 ), #91965, .F. ) ;
#8380=ADVANCED_FACE ( 'NONE', ( #73719 ), #16309, .F. ) ;
#8442=AXIS2_PLACEMENT_3D ( 'NONE', #197977, #37653, #221376 ) ;
#8481=AXIS2_PLACEMENT_3D ( 'NONE', #64042, #24942, #240122 ) ;
#8494=DIRECTION ( 'NONE',  ( 2.952720810173288619E-16, -1.000000000000000000, 0.000000000000000000 ) ) ;
#8515=VERTEX_POINT ( 'NONE', #98340 ) ;
#8531=EDGE_CURVE ( 'NONE', #137088, #28425, #179236, .T. ) ;
#8542=ORIENTED_EDGE ( 'NONE', *, *, #151246, .T. ) ;
#8573=EDGE_LOOP ( 'NONE', ( #5190, #101742, #92941, #251946 ) ) ;
#8587=ORIENTED_EDGE ( 'NONE', *, *, #126989, .F. ) ;
#8604=DIRECTION ( 'NONE',  ( 1.000000000000000000, 0.000000000000000000, 0.000000000000000000 ) ) ;
#8607=DIRECTION ( 'NONE',  ( -1.000000000000000000, 0.000000000000000000, 0.000000000000000000 ) ) ;
#8619=CARTESIAN_POINT ( 'NONE',  ( -20.85000000000000497, 11.74999999999999645, -26.58085275404129888 ) ) ;
#8632=CARTESIAN_POINT ( 'NONE',  ( -20.64999999999999858, 1.999999999999998224, -13.22462192276210224 ) ) ;
#8637=CARTESIAN_POINT ( 'NONE',  ( 21.05000000000000071, 8.776282895292474961, -8.558628995140949769 ) ) ;
#8645=CARTESIAN_POINT ( 'NONE',  ( -20.94999999999999929, 0.000000000000000000, 0.000000000000000000 ) ) ;
#8661=VERTEX_POINT ( 'NONE', #30423 ) ;
#8679=FACE_OUTER_BOUND ( 'NONE', #136288, .T. ) ;
#8727=CARTESIAN_POINT ( 'NONE',  ( -23.15000000000000213, 0.000000000000000000, 0.000000000000000000 ) ) ;
#8742=CIRCLE ( 'NONE', #225386, 0.1000000000000028644 ) ;
#8758=ORIENTED_EDGE ( 'NONE', *, *, #32710, .F. ) ;
#8759=EDGE_CURVE ( 'NONE', #123338, #186188, #168688, .T. ) ;
#8791=ORIENTED_EDGE ( 'NONE', *, *, #149288, .F. ) ;
#8793=CARTESIAN_POINT ( 'NONE',  ( -20.54999999999999716, 4.250000000000000000, -12.35000000000000142 ) ) ;
#8801=EDGE_CURVE ( 'NONE', #20836, #98230, #186979, .T. ) ;
#8818=ORIENTED_EDGE ( 'NONE', *, *, #256549, .T. ) ;
#8871=DIRECTION ( 'NONE',  ( -1.000000000000000000, 0.000000000000000000, 0.000000000000000000 ) ) ;
#8902=DIRECTION ( 'NONE',  ( 0.000000000000000000, 0.000000000000000000, -1.000000000000000000 ) ) ;
#8918=FACE_OUTER_BOUND ( 'NONE', #3345, .T. ) ;
#8954=CARTESIAN_POINT ( 'NONE',  ( 18.59999999999999787, -1.362429037193307435, -41.38888124792119783 ) ) ;
#8969=CARTESIAN_POINT ( 'NONE',  ( -20.64999999999999858, 7.249999999999999112, -21.15000000000000213 ) ) ;
#8973=EDGE_CURVE ( 'NONE', #49158, #207350, #128691, .T. ) ;
#9010=ORIENTED_EDGE ( 'NONE', *, *, #171322, .T. ) ;
#9031=ORIENTED_EDGE ( 'NONE', *, *, #224221, .F. ) ;
#9034=CARTESIAN_POINT ( 'NONE',  ( 20.04142135623731136, 11.75000000000000711, -24.65000000000000213 ) ) ;
#9048=ORIENTED_EDGE ( 'NONE', *, *, #60855, .T. ) ;
#9071=DIRECTION ( 'NONE',  ( 0.000000000000000000, 0.000000000000000000, -1.000000000000000000 ) ) ;
#9092=EDGE_LOOP ( 'NONE', ( #197591, #215666, #188118, #202048 ) ) ;
#9140=LINE ( 'NONE', #168256, #125943 ) ;
#9144=DIRECTION ( 'NONE',  ( 0.000000000000000000, -1.000000000000000000, -2.891205793294679805E-16 ) ) ;
#9185=DIRECTION ( 'NONE',  ( 0.000000000000000000, 0.000000000000000000, 1.000000000000000000 ) ) ;
#9201=CARTESIAN_POINT ( 'NONE',  ( -21.05000000000000071, 6.413662734869507887, -0.08559286336229579573 ) ) ;
#9216=VERTEX_POINT ( 'NONE', #33686 ) ;
#9228=EDGE_CURVE ( 'NONE', #156671, #193752, #220459, .T. ) ;
#9240=VECTOR ( 'NONE', #231816, 1000.000000000000000 ) ;
#9269=CARTESIAN_POINT ( 'NONE',  ( -21.65000000000000213, 7.708578643762696636, -21.25000000000000000 ) ) ;
#9302=DIRECTION ( 'NONE',  ( -0.000000000000000000, 0.000000000000000000, -1.000000000000000000 ) ) ;
#9366=DIRECTION ( 'NONE',  ( -4.391705002472929091E-16, 1.000000000000000000, 0.000000000000000000 ) ) ;
#9403=ORIENTED_EDGE ( 'NONE', *, *, #123253, .F. ) ;
#9409=DIRECTION ( 'NONE',  ( -1.000000000000000000, -0.000000000000000000, -0.000000000000000000 ) ) ;
#9413=DIRECTION ( 'NONE',  ( -1.000000000000000000, -0.000000000000000000, -0.000000000000000000 ) ) ;
#9436=CARTESIAN_POINT ( 'NONE',  ( -20.94999999999999929, -1.835859311443635233, -45.00443916879852679 ) ) ;
#9460=DIRECTION ( 'NONE',  ( 1.000000000000000000, 3.265361837132813093E-16, -0.000000000000000000 ) ) ;
#9461=DIRECTION ( 'NONE',  ( 0.000000000000000000, 0.000000000000000000, -1.000000000000000000 ) ) ;
#9470=VECTOR ( 'NONE', #76242, 1000.000000000000000 ) ;
#9480=ORIENTED_EDGE ( 'NONE', *, *, #178888, .T. ) ;
#9517=ORIENTED_EDGE ( 'NONE', *, *, #150988, .F. ) ;
#9524=CARTESIAN_POINT ( 'NONE',  ( 21.05000000000000071, -0.09999999999999939493, 0.000000000000000000 ) ) ;
#9554=ORIENTED_EDGE ( 'NONE', *, *, #108228, .F. ) ;
#9599=EDGE_CURVE ( 'NONE', #207350, #138366, #73761, .T. ) ;
#9684=EDGE_CURVE ( 'NONE', #219800, #150376, #140106, .T. ) ;
#9704=EDGE_LOOP ( 'NONE', ( #36339, #163113 ) ) ;
#9717=AXIS2_PLACEMENT_3D ( 'NONE', #174387, #22996, #82899 ) ;
#9738=CYLINDRICAL_SURFACE ( 'NONE', #229721, 0.09999999999999939493 ) ;
#9745=FILL_AREA_STYLE ('',( #89275 ) ) ;
#9767=DIRECTION ( 'NONE',  ( 0.000000000000000000, 0.9998779222360096863, -0.01562500000001061998 ) ) ;
#9777=DIRECTION ( 'NONE',  ( 0.000000000000000000, 0.000000000000000000, -1.000000000000000000 ) ) ;
#9785=CARTESIAN_POINT ( 'NONE',  ( -22.50000000000000000, 0.09999999999999939493, 11.64957080754479968 ) ) ;
#9811=DIRECTION ( 'NONE',  ( 0.000000000000000000, 0.000000000000000000, -1.000000000000000000 ) ) ;
#9839=FACE_OUTER_BOUND ( 'NONE', #98438, .T. ) ;
#9912=AXIS2_PLACEMENT_3D ( 'NONE', #217765, #39182, #118713 ) ;
#9917=ADVANCED_FACE ( 'NONE', ( #33075 ), #91713, .F. ) ;
#9926=DIRECTION ( 'NONE',  ( 1.000000000000000000, 0.000000000000000000, 0.000000000000000000 ) ) ;
#9990=DIRECTION ( 'NONE',  ( -1.836970198721029934E-16, 1.000000000000000000, 0.000000000000000000 ) ) ;
#10026=ORIENTED_EDGE ( 'NONE', *, *, #125080, .T. ) ;
#10069=ORIENTED_EDGE ( 'NONE', *, *, #192635, .F. ) ;
#10088=VECTOR ( 'NONE', #50298, 1000.000000000000000 ) ;
#10136=ORIENTED_EDGE ( 'NONE', *, *, #19425, .T. ) ;
#10144=CARTESIAN_POINT ( 'NONE',  ( -23.25000000000000000, 6.982009704856444898, -37.19615211825629331 ) ) ;
#10145=CARTESIAN_POINT ( 'NONE',  ( -20.94999999999999929, 5.849999999999952571, -10.13249722427796762 ) ) ;
#10150=EDGE_LOOP ( 'NONE', ( #5241, #172101, #38586, #91828, #47018 ) ) ;
#10152=AXIS2_PLACEMENT_3D ( 'NONE', #209448, #110348, #90773 ) ;
#10166=CARTESIAN_POINT ( 'NONE',  ( 21.08832698747859169, 8.775364393417216746, -12.22871746646415225 ) ) ;
#10190=EDGE_CURVE ( 'NONE', #119379, #94181, #100601, .T. ) ;
#10210=AXIS2_PLACEMENT_3D ( 'NONE', #76803, #74279, #32592 ) ;
#10241=ORIENTED_EDGE ( 'NONE', *, *, #3645, .F. ) ;
#10249=FACE_OUTER_BOUND ( 'NONE', #57648, .T. ) ;
#10250=DIRECTION ( 'NONE',  ( 1.000000000000000000, 0.000000000000000000, 0.000000000000000000 ) ) ;
#10260=DIRECTION ( 'NONE',  ( -1.000000000000000000, -3.265361837132813093E-16, 0.000000000000000000 ) ) ;
#10266=FACE_OUTER_BOUND ( 'NONE', #57926, .T. ) ;
#10272=CIRCLE ( 'NONE', #35416, 0.09999999999999939493 ) ;
#10299=AXIS2_PLACEMENT_3D ( 'NONE', #68331, #151743, #172611 ) ;
#10315=ORIENTED_EDGE ( 'NONE', *, *, #249936, .T. ) ;
#10334=CARTESIAN_POINT ( 'NONE',  ( 18.40000000000000213, -9.500000000000000000, -40.42214984933045940 ) ) ;
#10335=CARTESIAN_POINT ( 'NONE',  ( 19.96984138294294908, 11.75000000000005862, -24.72457207120111988 ) ) ;
#10352=ORIENTED_EDGE ( 'NONE', *, *, #141677, .T. ) ;
#10399=ORIENTED_EDGE ( 'NONE', *, *, #32685, .F. ) ;
#10441=CIRCLE ( 'NONE', #39680, 0.09999999999999939493 ) ;
#10446=ADVANCED_FACE ( 'NONE', ( #93875 ), #114732, .F. ) ;
#10498=EDGE_CURVE ( 'NONE', #83068, #94181, #118599, .T. ) ;
#10511=CARTESIAN_POINT ( 'NONE',  ( -18.50000000000000000, -9.400000000000005684, -7.297259759663287326 ) ) ;
#10512=CYLINDRICAL_SURFACE ( 'NONE', #249566, 0.09999999999999939493 ) ;
#10518=EDGE_CURVE ( 'NONE', #235552, #246027, #79430, .T. ) ;
#10525=CYLINDRICAL_SURFACE ( 'NONE', #200423, 0.09999999999999939493 ) ;
#10553=EDGE_CURVE ( 'NONE', #71337, #28028, #71806, .T. ) ;
#10591=FACE_OUTER_BOUND ( 'NONE', #68698, .T. ) ;
#10595=DIRECTION ( 'NONE',  ( 1.000000000000000000, 0.000000000000000000, 0.000000000000000000 ) ) ;
#10608=ORIENTED_EDGE ( 'NONE', *, *, #98569, .F. ) ;
#10653=FACE_OUTER_BOUND ( 'NONE', #241380, .T. ) ;
#10673=AXIS2_PLACEMENT_3D ( 'NONE', #42148, #121689, #201201 ) ;
#10707=EDGE_CURVE ( 'NONE', #72992, #4098, #146587, .T. ) ;
#10723=ORIENTED_EDGE ( 'NONE', *, *, #192563, .F. ) ;
#10739=ORIENTED_EDGE ( 'NONE', *, *, #7213, .F. ) ;
#10751=VERTEX_POINT ( 'NONE', #153600 ) ;
#10764=EDGE_CURVE ( 'NONE', #162495, #94704, #171867, .T. ) ;
#10777=ORIENTED_EDGE ( 'NONE', *, *, #81403, .F. ) ;
#10818=VERTEX_POINT ( 'NONE', #213510 ) ;
#10868=CARTESIAN_POINT ( 'NONE',  ( -22.60000000000094289, 0.1008583690985001419, 11.74956712348940790 ) ) ;
#10870=ORIENTED_EDGE ( 'NONE', *, *, #196952, .T. ) ;
#10878=DIRECTION ( 'NONE',  ( -1.000000000000000000, 0.000000000000000000, 0.000000000000000000 ) ) ;
#10885=DIRECTION ( 'NONE',  ( 1.000000000000000000, 0.000000000000000000, 0.000000000000000000 ) ) ;
#10889=ORIENTED_EDGE ( 'NONE', *, *, #57731, .T. ) ;
#10955=AXIS2_PLACEMENT_3D ( 'NONE', #127020, #227396, #205252 ) ;
#10973=ORIENTED_EDGE ( 'NONE', *, *, #144379, .T. ) ;
#10988=CARTESIAN_POINT ( 'NONE',  ( 18.59999999999999432, -1.135018845910178431, -41.21697688343231647 ) ) ;
#10994=DIRECTION ( 'NONE',  ( 0.000000000000000000, 0.000000000000000000, 1.000000000000000000 ) ) ;
#11014=CARTESIAN_POINT ( 'NONE',  ( 20.95512820512820440, 8.876151316288115822, -12.15000000000000036 ) ) ;
#11032=ORIENTED_EDGE ( 'NONE', *, *, #62228, .T. ) ;
#11034=DIRECTION ( 'NONE',  ( 0.000000000000000000, 0.000000000000000000, -1.000000000000000000 ) ) ;
#11036=VERTEX_POINT ( 'NONE', #225044 ) ;
#11041=ORIENTED_EDGE ( 'NONE', *, *, #144141, .T. ) ;
#11048=FACE_OUTER_BOUND ( 'NONE', #175054, .T. ) ;
#11080=CARTESIAN_POINT ( 'NONE',  ( -22.39999999999999858, 0.09999999999999939493, 7.790779598373403836 ) ) ;
#11085=VERTEX_POINT ( 'NONE', #211936 ) ;
#11112=VERTEX_POINT ( 'NONE', #72433 ) ;
#11150=CARTESIAN_POINT ( 'NONE',  ( -21.29999999999995808, 0.000000000000000000, 0.000000000000000000 ) ) ;
#11162=CARTESIAN_POINT ( 'NONE',  ( 20.04142135623730070, 11.75000000000000355, 11.75000000000000000 ) ) ;
#11215=DIRECTION ( 'NONE',  ( -3.787827842127535236E-15, 0.7397360091702777085, 0.6728971962616808744 ) ) ;
#11219=EDGE_CURVE ( 'NONE', #190309, #177816, #24983, .T. ) ;
#11271=DIRECTION ( 'NONE',  ( 0.000000000000000000, 0.000000000000000000, -1.000000000000000000 ) ) ;
#11284=EDGE_CURVE ( 'NONE', #180654, #214033, #38841, .T. ) ;
#11285=DIRECTION ( 'NONE',  ( 0.000000000000000000, 1.000000000000000000, 0.000000000000000000 ) ) ;
#11322=VERTEX_POINT ( 'NONE', #116669 ) ;
#11334=DIRECTION ( 'NONE',  ( -0.000000000000000000, 1.000000000000000000, 0.000000000000000000 ) ) ;
#11362=DIRECTION ( 'NONE',  ( 0.000000000000000000, 1.000000000000000000, -6.308085367188393199E-16 ) ) ;
#11407=ORIENTED_EDGE ( 'NONE', *, *, #195968, .T. ) ;
#11423=DIRECTION ( 'NONE',  ( 1.000000000000000000, 0.000000000000000000, 9.486769009248220990E-16 ) ) ;
#11444=CIRCLE ( 'NONE', #32303, 0.09999999999999939493 ) ;
#11450=ORIENTED_EDGE ( 'NONE', *, *, #66730, .T. ) ;
#11477=DIRECTION ( 'NONE',  ( 1.000000000000000000, 7.304098846218134667E-16, -0.000000000000000000 ) ) ;
#11479=ORIENTED_EDGE ( 'NONE', *, *, #131217, .T. ) ;
#11485=DIRECTION ( 'NONE',  ( 0.000000000000000000, 0.000000000000000000, -1.000000000000000000 ) ) ;
#11495=AXIS2_PLACEMENT_3D ( 'NONE', #244947, #66324, #145839 ) ;
#11516=ORIENTED_EDGE ( 'NONE', *, *, #90347, .F. ) ;
#11534=DIRECTION ( 'NONE',  ( 0.000000000000000000, 1.000000000000000000, 0.000000000000000000 ) ) ;
#11549=CARTESIAN_POINT ( 'NONE',  ( 21.05000000000000071, 11.65000000000000746, -12.15000000000000036 ) ) ;
#11554=ORIENTED_EDGE ( 'NONE', *, *, #147138, .F. ) ;
#11555=CYLINDRICAL_SURFACE ( 'NONE', #236126, 0.09999999999999939493 ) ;
#11560=EDGE_CURVE ( 'NONE', #221017, #128093, #49765, .T. ) ;
#11569=DIRECTION ( 'NONE',  ( -1.000000000000000000, 6.938893903907270030E-14, 0.000000000000000000 ) ) ;
#11586=CARTESIAN_POINT ( 'NONE',  ( 21.00000000000000000, 9.749999999999998224, -21.25000000000000000 ) ) ;
#11594=ORIENTED_EDGE ( 'NONE', *, *, #119400, .F. ) ;
#11603=DIRECTION ( 'NONE',  ( 0.000000000000000000, 1.000000000000000000, 0.000000000000000000 ) ) ;
#11613=CIRCLE ( 'NONE', #65760, 4.149999999999999467 ) ;
#11636=VERTEX_POINT ( 'NONE', #5054 ) ;
#11669=ORIENTED_EDGE ( 'NONE', *, *, #61107, .F. ) ;
#11683=ORIENTED_EDGE ( 'NONE', *, *, #128956, .F. ) ;
#11696=ORIENTED_EDGE ( 'NONE', *, *, #3514, .F. ) ;
#11697=ORIENTED_EDGE ( 'NONE', *, *, #33819, .T. ) ;
#11761=CARTESIAN_POINT ( 'NONE',  ( 20.94999999999999929, 0.000000000000000000, -37.50000000000000000 ) ) ;
#11776=CARTESIAN_POINT ( 'NONE',  ( 22.47110162079220785, 0.02879741280269312517, 11.64993593668433469 ) ) ;
#11788=CARTESIAN_POINT ( 'NONE',  ( -21.05000000000000071, 0.09779029130878996723, 6.257814610476121864 ) ) ;
#11803=CARTESIAN_POINT ( 'NONE',  ( -20.94999999999999929, -11.75000000000000000, -2.900000000000003464 ) ) ;
#11814=CARTESIAN_POINT ( 'NONE',  ( 20.04142135623730070, 11.65000000000000391, -21.35000000000000142 ) ) ;
#11830=DIRECTION ( 'NONE',  ( 1.000000000000000000, -0.000000000000000000, -0.000000000000000000 ) ) ;
#11849=DIRECTION ( 'NONE',  ( 0.000000000000000000, 0.9998779222360100194, 0.01562499999998606150 ) ) ;
#11854=FACE_OUTER_BOUND ( 'NONE', #136239, .T. ) ;
#11933=CARTESIAN_POINT ( 'NONE',  ( 21.14999999999998082, -11.75000000000000000, 3.469446951953614189E-15 ) ) ;
#11948=CARTESIAN_POINT ( 'NONE',  ( 20.94999999999999574, -1.249999999999999334, -8.000000000000000000 ) ) ;
#12009=ADVANCED_FACE ( 'NONE', ( #256465 ), #119611, .F. ) ;
#12023=ORIENTED_EDGE ( 'NONE', *, *, #245277, .F. ) ;
#12039=ORIENTED_EDGE ( 'NONE', *, *, #175617, .F. ) ;
#12048=AXIS2_PLACEMENT_3D ( 'NONE', #21430, #100888, #141347 ) ;
#12068=CARTESIAN_POINT ( 'NONE',  ( -20.54999999999999716, 2.499999999999998668, -20.27537807723789953 ) ) ;
#12100=DIRECTION ( 'NONE',  ( 0.000000000000000000, 0.2605042016806715099, 0.9654727137038706664 ) ) ;
#12142=DIRECTION ( 'NONE',  ( 0.000000000000000000, 0.000000000000000000, -1.000000000000000000 ) ) ;
#12159=ORIENTED_EDGE ( 'NONE', *, *, #131217, .F. ) ;
#12160=AXIS2_PLACEMENT_3D ( 'NONE', #97395, #182113, #239519 ) ;
#12226=EDGE_LOOP ( 'NONE', ( #62080, #241108, #191770, #165333, #241458, #101221, #189690, #151306, #3079, #147383, #79872 ) ) ;
#12228=CYLINDRICAL_SURFACE ( 'NONE', #171827, 0.1000000000000008105 ) ;
#12230=CARTESIAN_POINT ( 'NONE',  ( -23.15000000000000213, -11.65000000000000036, -30.39999999999999503 ) ) ;
#12316=FACE_OUTER_BOUND ( 'NONE', #80816, .T. ) ;
#12318=CARTESIAN_POINT ( 'NONE',  ( 20.12500000000000355, 10.24195072708267240, -7.860203727086118697 ) ) ;
#12324=EDGE_LOOP ( 'NONE', ( #69127, #202779, #176505, #35667, #176251 ) ) ;
#12340=DIRECTION ( 'NONE',  ( 1.000000000000000000, 0.000000000000000000, 0.000000000000000000 ) ) ;
#12346=DIRECTION ( 'NONE',  ( 1.000000000000000000, -0.000000000000000000, -0.000000000000000000 ) ) ;
#12383=LINE ( 'NONE', #189714, #74011 ) ;
#12452=CARTESIAN_POINT ( 'NONE',  ( -23.24999999999999645, -9.600000000000003197, -40.20018939122204671 ) ) ;
#12475=CIRCLE ( 'NONE', #199912, 0.09999999999999939493 ) ;
#12480=DIRECTION ( 'NONE',  ( 0.000000000000000000, 1.000000000000000000, -1.224646799147353207E-16 ) ) ;
#12566=EDGE_CURVE ( 'NONE', #26218, #137088, #201691, .T. ) ;
#12603=EDGE_CURVE ( 'NONE', #161501, #108803, #176206, .T. ) ;
#12604=DIRECTION ( 'NONE',  ( 0.000000000000000000, -1.000000000000000000, 0.000000000000000000 ) ) ;
#12662=AXIS2_PLACEMENT_3D ( 'NONE', #27321, #67685, #168122 ) ;
#12690=EDGE_CURVE ( 'NONE', #197777, #154965, #52573, .T. ) ;
#12727=ORIENTED_EDGE ( 'NONE', *, *, #40912, .T. ) ;
#12737=DIRECTION ( 'NONE',  ( 0.000000000000000000, 0.000000000000000000, 1.000000000000000000 ) ) ;
#12746=ORIENTED_EDGE ( 'NONE', *, *, #77368, .F. ) ;
#12754=VERTEX_POINT ( 'NONE', #253348 ) ;
#12778=FACE_OUTER_BOUND ( 'NONE', #233232, .T. ) ;
#12806=DIRECTION ( 'NONE',  ( 0.000000000000000000, 0.000000000000000000, -1.000000000000000000 ) ) ;
#12815=AXIS2_PLACEMENT_3D ( 'NONE', #196230, #52863, #15052 ) ;
#12830=CARTESIAN_POINT ( 'NONE',  ( -23.25000000000000000, 0.000000000000000000, 0.000000000000000000 ) ) ;
#12836=DIRECTION ( 'NONE',  ( 7.589415207398576792E-15, -1.000000000000000000, -0.000000000000000000 ) ) ;
#12839=CARTESIAN_POINT ( 'NONE',  ( 23.25000000000000000, -11.48912529307605546, -30.39999999999999503 ) ) ;
#12846=CARTESIAN_POINT ( 'NONE',  ( 23.15000000000000213, -8.663551401869158397, -9.524101118067305194 ) ) ;
#12866=ORIENTED_EDGE ( 'NONE', *, *, #163109, .F. ) ;
#12867=DIRECTION ( 'NONE',  ( 0.7071067811865487940, 0.000000000000000000, -0.7071067811865463515 ) ) ;
#12896=CARTESIAN_POINT ( 'NONE',  ( 18.52165635395184751, -9.481150711282177568, -7.024837582862474505 ) ) ;
#12915=AXIS2_PLACEMENT_3D ( 'NONE', #226295, #168961, #64673 ) ;
#12978=DIRECTION ( 'NONE',  ( 0.000000000000000000, 0.000000000000000000, -1.000000000000000000 ) ) ;
#12979=ORIENTED_EDGE ( 'NONE', *, *, #31337, .T. ) ;
#13028=AXIS2_PLACEMENT_3D ( 'NONE', #86582, #166188, #67055 ) ;
#13050=ADVANCED_FACE ( 'NONE', ( #230939 ), #101291, .F. ) ;
#13055=VECTOR ( 'NONE', #77517, 1000.000000000000227 ) ;
#13062=CARTESIAN_POINT ( 'NONE',  ( 21.93642651522410603, 7.327166239325793029, -1.462266042833915125E-16 ) ) ;
#13074=EDGE_LOOP ( 'NONE', ( #91816, #201390, #55241, #223903 ) ) ;
#13099=FACE_OUTER_BOUND ( 'NONE', #180748, .T. ) ;
#13117=DIRECTION ( 'NONE',  ( 0.000000000000000000, 0.000000000000000000, 1.000000000000000000 ) ) ;
#13132=CIRCLE ( 'NONE', #204641, 0.1000000000000002554 ) ;
#13141=CARTESIAN_POINT ( 'NONE',  ( -18.59999999999999787, 9.150000000000002132, 11.75000000000000000 ) ) ;
#13153=EDGE_CURVE ( 'NONE', #71883, #191690, #122205, .T. ) ;
#13161=ORIENTED_EDGE ( 'NONE', *, *, #223629, .F. ) ;
#13163=AXIS2_PLACEMENT_3D ( 'NONE', #125874, #123328, #82867 ) ;
#13168=CARTESIAN_POINT ( 'NONE',  ( -20.94999999999999929, 0.000000000000000000, 0.000000000000000000 ) ) ;
#13180=ADVANCED_FACE ( 'NONE', ( #62226 ), #255429, .T. ) ;
#13181=ORIENTED_EDGE ( 'NONE', *, *, #247520, .T. ) ;
#13199=VERTEX_POINT ( 'NONE', #2227 ) ;
#13237=EDGE_LOOP ( 'NONE', ( #236838, #214454, #160225, #164478, #113729 ) ) ;
#13240=FACE_OUTER_BOUND ( 'NONE', #158831, .T. ) ;
#13242=VERTEX_POINT ( 'NONE', #119645 ) ;
#13244=AXIS2_PLACEMENT_3D ( 'NONE', #82882, #209280, #188433 ) ;
#13253=CARTESIAN_POINT ( 'NONE',  ( 18.59999999999999076, -1.249999999999999334, -7.999999999999998224 ) ) ;
#13275=ORIENTED_EDGE ( 'NONE', *, *, #229800, .F. ) ;
#13282=ORIENTED_EDGE ( 'NONE', *, *, #247520, .F. ) ;
#13291=FACE_OUTER_BOUND ( 'NONE', #187765, .T. ) ;
#13320=ORIENTED_EDGE ( 'NONE', *, *, #227151, .T. ) ;
#13330=CARTESIAN_POINT ( 'NONE',  ( -20.54999999999999716, -9.000000000000003553, -9.893969122652444881 ) ) ;
#13345=CARTESIAN_POINT ( 'NONE',  ( -20.94999999999999929, 5.900000000000005684, -23.28090023534362629 ) ) ;
#13348=VECTOR ( 'NONE', #18195, 1000.000000000000000 ) ;
#13352=TOROIDAL_SURFACE ( 'NONE', #50733, 11.65000000000000036, 0.1000000000000000056 ) ;
#13362=CARTESIAN_POINT ( 'NONE',  ( 20.94999999999999929, -11.29603075033528548, -3.047899159663867152 ) ) ;
#13378=DIRECTION ( 'NONE',  ( 1.000000000000000000, 0.000000000000000000, 0.000000000000000000 ) ) ;
#13393=ORIENTED_EDGE ( 'NONE', *, *, #158154, .T. ) ;
#13446=DIRECTION ( 'NONE',  ( -0.000000000000000000, 0.1350103645451626311, 0.9908441862701635738 ) ) ;
#13450=CARTESIAN_POINT ( 'NONE',  ( 21.05000000000000071, -9.000000000000000000, -24.10603087734755690 ) ) ;
#13455=FACE_OUTER_BOUND ( 'NONE', #120093, .T. ) ;
#13503=CARTESIAN_POINT ( 'NONE',  ( 21.05000000000000071, 11.60000000000000675, -26.57179676972450011 ) ) ;
#13510=DIRECTION ( 'NONE',  ( 1.000000000000000000, 2.952720810173289112E-16, -0.000000000000000000 ) ) ;
#13528=ORIENTED_EDGE ( 'NONE', *, *, #10498, .F. ) ;
#13537=LINE ( 'NONE', #252127, #189098 ) ;
#13560=AXIS2_PLACEMENT_3D ( 'NONE', #77363, #164630, #143761 ) ;
#13570=DIRECTION ( 'NONE',  ( 0.000000000000000000, 0.000000000000000000, -1.000000000000000000 ) ) ;
#13580=ADVANCED_FACE ( 'NONE', ( #95461 ), #156756, .F. ) ;
#13594=CARTESIAN_POINT ( 'NONE',  ( -18.59999999999999787, -1.362429037193310988, -41.38888124792119783 ) ) ;
#13661=CARTESIAN_POINT ( 'NONE',  ( -21.05000000000000071, 0.000000000000000000, 0.000000000000000000 ) ) ;
#13667=LINE ( 'NONE', #232733, #178783 ) ;
#13692=FACE_OUTER_BOUND ( 'NONE', #103862, .T. ) ;
#13703=DIRECTION ( 'NONE',  ( 0.000000000000000000, 0.000000000000000000, -1.000000000000000000 ) ) ;
#13729=DIRECTION ( 'NONE',  ( 0.000000000000000000, -1.000000000000000000, 0.000000000000000000 ) ) ;
#13732=AXIS2_PLACEMENT_3D ( 'NONE', #5708, #83937, #240496 ) ;
#13746=CARTESIAN_POINT ( 'NONE',  ( 21.09546886439535029, 8.878553113014918452, -12.23709385055535925 ) ) ;
#13769=CARTESIAN_POINT ( 'NONE',  ( 21.05000000000000071, 0.000000000000000000, -33.50000000000000000 ) ) ;
#13771=VECTOR ( 'NONE', #61471, 1000.000000000000000 ) ;
#13785=DIRECTION ( 'NONE',  ( 0.000000000000000000, 0.000000000000000000, 1.000000000000000000 ) ) ;
#13788=DIRECTION ( 'NONE',  ( 0.000000000000000000, 0.000000000000000000, -1.000000000000000000 ) ) ;
#13791=DIRECTION ( 'NONE',  ( 1.000000000000000000, 0.000000000000000000, 0.000000000000000000 ) ) ;
#13819=ADVANCED_FACE ( 'NONE', ( #138224 ), #79535, .T. ) ;
#13823=LINE ( 'NONE', #150766, #16940 ) ;
#13825=EDGE_CURVE ( 'NONE', #233908, #143318, #26725, .T. ) ;
#13852=CARTESIAN_POINT ( 'NONE',  ( 20.94999999999999929, 5.850000000000004086, -23.36750277572207679 ) ) ;
#13860=VERTEX_POINT ( 'NONE', #76983 ) ;
#13865=ORIENTED_EDGE ( 'NONE', *, *, #185215, .F. ) ;
#13883=CIRCLE ( 'NONE', #43111, 0.1000000000000008799 ) ;
#13884=CARTESIAN_POINT ( 'NONE',  ( 22.39999999999999503, -5.963111948670274387E-16, 7.790779598373379855 ) ) ;
#13885=VERTEX_POINT ( 'NONE', #20899 ) ;
#13917=CYLINDRICAL_SURFACE ( 'NONE', #2013, 0.09999999999999939493 ) ;
#13928=CARTESIAN_POINT ( 'NONE',  ( 18.59999999999999432, -1.162701749938011453, -8.099999999999999645 ) ) ;
#13949=ORIENTED_EDGE ( 'NONE', *, *, #164570, .F. ) ;
#13964=EDGE_LOOP ( 'NONE', ( #3704, #39307, #23126, #102271 ) ) ;
#13967=ORIENTED_EDGE ( 'NONE', *, *, #247179, .F. ) ;
#13977=CARTESIAN_POINT ( 'NONE',  ( -21.14999999999999858, 0.000000000000000000, 6.540656951701240729 ) ) ;
#14030=ORIENTED_EDGE ( 'NONE', *, *, #60971, .F. ) ;
#14031=DIRECTION ( 'NONE',  ( -0.000000000000000000, 0.9876197685951279004, -0.1568667991644694115 ) ) ;
#14037=EDGE_CURVE ( 'NONE', #230288, #101170, #160191, .T. ) ;
#14048=CARTESIAN_POINT ( 'NONE',  ( -21.44999999999999929, 7.249999999999999112, -21.15000000000000213 ) ) ;
#14110=DIRECTION ( 'NONE',  ( 1.000000000000000000, 0.000000000000000000, 0.000000000000000000 ) ) ;
#14130=CIRCLE ( 'NONE', #184781, 0.8750000000000007772 ) ;
#14140=B_SPLINE_CURVE_WITH_KNOTS ( 'NONE', 3,
 ( #107693, #206803, #106391, #28198, #249778, #89408, #189811, #131107, #49003, #67287, #228936, #187257, #248496, #69879, #146805, #128549, #85528, #208105, #230209 ),
 .UNSPECIFIED., .F., .F.,
 ( 4, 3, 3, 3, 3, 3, 4 ),
 ( 1.387778780781445676E-17, 2.646747978908994698E-05, 5.271166642128863382E-05, 9.008788829885137981E-05, 0.0001426648776561022008, 0.0001897378458659801945, 0.0001917382627806380965 ),
 .UNSPECIFIED. ) ;
#14148=AXIS2_PLACEMENT_3D ( 'NONE', #51423, #228825, #69759 ) ;
#14154=ORIENTED_EDGE ( 'NONE', *, *, #192563, .T. ) ;
#14166=EDGE_CURVE ( 'NONE', #49960, #235552, #97777, .T. ) ;
#14179=CARTESIAN_POINT ( 'NONE',  ( 18.51997666896852124, -9.392332131518996263, -7.143406187483815728 ) ) ;
#14189=AXIS2_PLACEMENT_3D ( 'NONE', #254385, #154080, #178772 ) ;
#14194=CARTESIAN_POINT ( 'NONE',  ( 18.37172112093847787, -9.570961652243262563, -40.31673445348319973 ) ) ;
#14217=CIRCLE ( 'NONE', #180594, 0.1999999999999999833 ) ;
#14241=CARTESIAN_POINT ( 'NONE',  ( -21.44999999999999929, 7.150000000000000355, -21.25000000000000000 ) ) ;
#14265=DIRECTION ( 'NONE',  ( 0.000000000000000000, 0.000000000000000000, 1.000000000000000000 ) ) ;
#14267=ORIENTED_EDGE ( 'NONE', *, *, #36215, .F. ) ;
#14269=AXIS2_PLACEMENT_3D ( 'NONE', #97839, #219088, #254354 ) ;
#14273=VECTOR ( 'NONE', #85469, 1000.000000000000000 ) ;
#14298=CARTESIAN_POINT ( 'NONE',  ( 18.49999999999999289, 10.49142135623730709, -24.85000000000000142 ) ) ;
#14302=CARTESIAN_POINT ( 'NONE',  ( -20.94999999999999929, -1.835341550224411922, -11.55515129256298046 ) ) ;
#14307=ORIENTED_EDGE ( 'NONE', *, *, #164273, .T. ) ;
#14348=ADVANCED_FACE ( 'NONE', ( #97493 ), #154964, .T. ) ;
#14360=EDGE_CURVE ( 'NONE', #252532, #212201, #147891, .T. ) ;
#14363=CIRCLE ( 'NONE', #231019, 11.70000000000000284 ) ;
#14375=EDGE_CURVE ( 'NONE', #202242, #180038, #239464, .T. ) ;
#14399=CARTESIAN_POINT ( 'NONE',  ( 18.49999999999998934, 10.25000000261906941, -24.68717194963243600 ) ) ;
#14436=CYLINDRICAL_SURFACE ( 'NONE', #64384, 0.1000000000000008105 ) ;
#14446=EDGE_CURVE ( 'NONE', #244526, #202111, #97963, .T. ) ;
#14447=EDGE_LOOP ( 'NONE', ( #73022, #247290, #42877 ) ) ;
#14459=FACE_OUTER_BOUND ( 'NONE', #191373, .T. ) ;
#14460=EDGE_CURVE ( 'NONE', #73708, #209135, #39580, .T. ) ;
#14476=ORIENTED_EDGE ( 'NONE', *, *, #157233, .T. ) ;
#14495=CARTESIAN_POINT ( 'NONE',  ( 18.49999999999998934, 19.85039924723355398, -2.280303057801358335 ) ) ;
#14522=CARTESIAN_POINT ( 'NONE',  ( -20.85000000000000142, 6.933893972126341509, -37.28564583437357527 ) ) ;
#14569=ORIENTED_EDGE ( 'NONE', *, *, #79494, .T. ) ;
#14592=AXIS2_PLACEMENT_3D ( 'NONE', #227111, #131877, #210144 ) ;
#14610=LINE ( 'NONE', #168578, #198406 ) ;
#14618=ORIENTED_EDGE ( 'NONE', *, *, #192808, .F. ) ;
#14627=LINE ( 'NONE', #253205, #231484 ) ;
#14631=CARTESIAN_POINT ( 'NONE',  ( 20.94999999999999929, -8.663551401869154844, -23.97589888193268948 ) ) ;
#14737=CIRCLE ( 'NONE', #156397, 0.09999999999999939493 ) ;
#14772=AXIS2_PLACEMENT_3D ( 'NONE', #246451, #147351, #207341 ) ;
#14792=VECTOR ( 'NONE', #155691, 1000.000000000000000 ) ;
#14804=EDGE_CURVE ( 'NONE', #14945, #8661, #119037, .T. ) ;
#14819=EDGE_CURVE ( 'NONE', #226285, #41654, #39932, .T. ) ;
#14841=DIRECTION ( 'NONE',  ( -1.000000000000000000, 0.000000000000000000, 0.000000000000000000 ) ) ;
#14848=CARTESIAN_POINT ( 'NONE',  ( -20.54999999999999716, -9.000000000000001776, -23.60603087734756045 ) ) ;
#14859=ORIENTED_EDGE ( 'NONE', *, *, #114447, .F. ) ;
#14945=VERTEX_POINT ( 'NONE', #174906 ) ;
#14979=DIRECTION ( 'NONE',  ( 0.000000000000000000, 1.000000000000000000, -6.938893903907270030E-14 ) ) ;
#14982=ADVANCED_FACE ( 'NONE', ( #143420 ), #98138, .T. ) ;
#14993=TOROIDAL_SURFACE ( 'NONE', #227363, 0.2000000000000000111, 0.1000000000000000056 ) ;
#15004=CARTESIAN_POINT ( 'NONE',  ( -22.59999999999999787, 0.1008583690987122083, 11.74956712348939192 ) ) ;
#15008=AXIS2_PLACEMENT_3D ( 'NONE', #151579, #169875, #251926 ) ;
#15012=CARTESIAN_POINT ( 'NONE',  ( -18.59999999999999787, 11.64999999999999680, -12.14999999999999858 ) ) ;
#15014=AXIS2_PLACEMENT_3D ( 'NONE', #250738, #73425, #74723 ) ;
#15052=DIRECTION ( 'NONE',  ( 0.000000000000000000, 0.000000000000000000, -1.000000000000000000 ) ) ;
#15065=DIRECTION ( 'NONE',  ( 0.000000000000000000, 0.8700118002898321601, -0.4930308989875230030 ) ) ;
#15079=DIRECTION ( 'NONE',  ( 0.000000000000000000, 0.000000000000000000, 1.000000000000000000 ) ) ;
#15082=EDGE_CURVE ( 'NONE', #4416, #62328, #189937, .T. ) ;
#15210=ORIENTED_EDGE ( 'NONE', *, *, #241183, .F. ) ;
#15211=CARTESIAN_POINT ( 'NONE',  ( 21.05000000000000071, 5.499999999999998224, -21.09473398108690390 ) ) ;
#15227=AXIS2_PLACEMENT_3D ( 'NONE', #11150, #153261, #16305 ) ;
#15233=TOROIDAL_SURFACE ( 'NONE', #106791, 11.90000000000000213, 0.1000000000000000056 ) ;
#15278=CARTESIAN_POINT ( 'NONE',  ( -21.05000000000000071, -11.48912529307605901, -2.900000000000001688 ) ) ;
#15326=DIRECTION ( 'NONE',  ( 0.000000000000000000, 0.000000000000000000, -1.000000000000000000 ) ) ;
#15332=ORIENTED_EDGE ( 'NONE', *, *, #135325, .T. ) ;
#15358=AXIS2_PLACEMENT_3D ( 'NONE', #38588, #163676, #244481 ) ;
#15383=DIRECTION ( 'NONE',  ( 2.952720810173289112E-16, -1.000000000000000000, 0.000000000000000000 ) ) ;
#15391=CARTESIAN_POINT ( 'NONE',  ( 19.75857864376268935, 11.75000000000000355, -24.85000000000000142 ) ) ;
#15412=DIRECTION ( 'NONE',  ( 0.000000000000000000, 0.000000000000000000, 1.000000000000000000 ) ) ;
#15428=ORIENTED_EDGE ( 'NONE', *, *, #57389, .T. ) ;
#15442=CARTESIAN_POINT ( 'NONE',  ( -21.05000000000000071, 6.257814610476114758, 0.09779029130879343668 ) ) ;
#15468=CARTESIAN_POINT ( 'NONE',  ( 18.41832399655377372, -9.682403266673746955, -40.15684362002786401 ) ) ;
#15510=EDGE_CURVE ( 'NONE', #250352, #112246, #231650, .T. ) ;
#15569=VECTOR ( 'NONE', #154916, 1000.000000000000000 ) ;
#15571=EDGE_LOOP ( 'NONE', ( #181339, #200859, #159091, #36117 ) ) ;
#15585=EDGE_CURVE ( 'NONE', #224010, #175406, #86028, .T. ) ;
#15601=CIRCLE ( 'NONE', #40554, 0.1999999999999987899 ) ;
#15609=EDGE_CURVE ( 'NONE', #238460, #83068, #177691, .T. ) ;
#15622=DIRECTION ( 'NONE',  ( 0.000000000000000000, -1.000000000000000000, 0.000000000000000000 ) ) ;
#15628=VERTEX_POINT ( 'NONE', #154692 ) ;
#15634=CARTESIAN_POINT ( 'NONE',  ( -20.54999999999999716, 1.999999999999998224, -20.27537807723789953 ) ) ;
#15640=CARTESIAN_POINT ( 'NONE',  ( 20.94999999999999574, 0.000000000000000000, 0.000000000000000000 ) ) ;
#15672=AXIS2_PLACEMENT_3D ( 'NONE', #222405, #244561, #5935 ) ;
#15674=DIRECTION ( 'NONE',  ( 0.000000000000000000, 0.000000000000000000, -1.000000000000000000 ) ) ;
#15721=CYLINDRICAL_SURFACE ( 'NONE', #24414, 0.09999999999999939493 ) ;
#15744=VECTOR ( 'NONE', #224850, 1000.000000000000000 ) ;
#15746=DIRECTION ( 'NONE',  ( 2.952720810173289112E-16, -1.000000000000000000, 0.000000000000000000 ) ) ;
#15785=CARTESIAN_POINT ( 'NONE',  ( -20.94999999999999929, 1.162701749938009677, -8.000000000000000000 ) ) ;
#15844=FACE_OUTER_BOUND ( 'NONE', #172963, .T. ) ;
#15866=VECTOR ( 'NONE', #27145, 1000.000000000000000 ) ;
#15883=ORIENTED_EDGE ( 'NONE', *, *, #130796, .T. ) ;
#15886=AXIS2_PLACEMENT_3D ( 'NONE', #94771, #92199, #34833 ) ;
#15921=DIRECTION ( 'NONE',  ( 0.000000000000000000, 1.897661533703519897E-16, -1.000000000000000000 ) ) ;
#15931=ADVANCED_FACE ( 'NONE', ( #29317, #107519, #151817 ), #51366, .F. ) ;
#15934=VERTEX_POINT ( 'NONE', #28023 ) ;
#15958=EDGE_CURVE ( 'NONE', #140958, #72309, #77859, .T. ) ;
#15964=FACE_OUTER_BOUND ( 'NONE', #93420, .T. ) ;
#15971=AXIS2_PLACEMENT_3D ( 'NONE', #249471, #89092, #248177 ) ;
#15975=VERTEX_POINT ( 'NONE', #30584 ) ;
#15979=ORIENTED_EDGE ( 'NONE', *, *, #116788, .F. ) ;
#16006=CIRCLE ( 'NONE', #124310, 0.09999999999999939493 ) ;
#16031=CARTESIAN_POINT ( 'NONE',  ( 21.05000000000000071, 4.850467289719617270, -12.03426740900167857 ) ) ;
#16047=ORIENTED_EDGE ( 'NONE', *, *, #151680, .F. ) ;
#16088=DIRECTION ( 'NONE',  ( 0.000000000000000000, 1.000000000000000000, 1.734723475976817507E-14 ) ) ;
#16093=CIRCLE ( 'NONE', #215944, 0.09999999999999939493 ) ;
#16101=CARTESIAN_POINT ( 'NONE',  ( 23.14999999999999503, 11.65000000000000746, 11.75000000000000000 ) ) ;
#16102=CIRCLE ( 'NONE', #199242, 0.09999999999999939493 ) ;
#16135=EDGE_CURVE ( 'NONE', #186188, #49960, #253447, .T. ) ;
#16181=CIRCLE ( 'NONE', #161929, 11.90000000000000391 ) ;
#16185=AXIS2_PLACEMENT_3D ( 'NONE', #29683, #184867, #84439 ) ;
#16196=CARTESIAN_POINT ( 'NONE',  ( -23.25000000000000000, 4.837354856632041113E-16, -29.60000000000000142 ) ) ;
#16210=DIRECTION ( 'NONE',  ( -0.000000000000000000, 0.9876197685951276783, 0.1568667991644721316 ) ) ;
#16212=AXIS2_PLACEMENT_3D ( 'NONE', #169919, #211573, #225952 ) ;
#16232=AXIS2_PLACEMENT_3D ( 'NONE', #23925, #203811, #120463 ) ;
#16264=AXIS2_PLACEMENT_3D ( 'NONE', #16689, #217414, #136598 ) ;
#16292=ADVANCED_FACE ( 'NONE', ( #90206 ), #245472, .T. ) ;
#16300=ORIENTED_EDGE ( 'NONE', *, *, #134881, .F. ) ;
#16305=DIRECTION ( 'NONE',  ( 0.000000000000000000, 0.000000000000000000, -1.000000000000000000 ) ) ;
#16309=CYLINDRICAL_SURFACE ( 'NONE', #203337, 0.5000000000000004441 ) ;
#16337=LINE ( 'NONE', #253620, #205137 ) ;
#16347=CYLINDRICAL_SURFACE ( 'NONE', #204949, 7.900000000000003908 ) ;
#16376=CARTESIAN_POINT ( 'NONE',  ( -20.94999999999999929, 7.021664781900089913, -37.33356540189728889 ) ) ;
#16415=CARTESIAN_POINT ( 'NONE',  ( 20.94999999999999929, -9.400000000000002132, -9.893969122652443104 ) ) ;
#16423=ORIENTED_EDGE ( 'NONE', *, *, #137323, .T. ) ;
#16437=EDGE_CURVE ( 'NONE', #75563, #62135, #102986, .T. ) ;
#16461=EDGE_CURVE ( 'NONE', #50256, #172993, #194617, .T. ) ;
#16467=ORIENTED_EDGE ( 'NONE', *, *, #130630, .F. ) ;
#16469=DIRECTION ( 'NONE',  ( 0.000000000000000000, 0.000000000000000000, -1.000000000000000000 ) ) ;
#16494=VERTEX_POINT ( 'NONE', #175886 ) ;
#16503=VERTEX_POINT ( 'NONE', #140575 ) ;
#16504=DIRECTION ( 'NONE',  ( 0.000000000000000000, -0.9908441862701596881, 0.1350103645451904977 ) ) ;
#16516=EDGE_CURVE ( 'NONE', #108350, #169542, #161460, .T. ) ;
#16522=EDGE_LOOP ( 'NONE', ( #223656, #245540, #197763, #150986 ) ) ;
#16525=VERTEX_POINT ( 'NONE', #67461 ) ;
#16529=CARTESIAN_POINT ( 'NONE',  ( 20.95443524775735256, 8.878554263872812768, -8.533722275600151619 ) ) ;
#16531=DIRECTION ( 'NONE',  ( 1.000000000000000000, 0.000000000000000000, 0.000000000000000000 ) ) ;
#16540=CARTESIAN_POINT ( 'NONE',  ( -23.15000000000000213, 4.349999999999999645, -12.25000000000000000 ) ) ;
#16568=CARTESIAN_POINT ( 'NONE',  ( 20.95263205890667635, 8.895740107894022586, -8.489508406941629559 ) ) ;
#16572=DIRECTION ( 'NONE',  ( 1.000000000000000000, 0.000000000000000000, 0.000000000000000000 ) ) ;
#16606=ORIENTED_EDGE ( 'NONE', *, *, #92327, .F. ) ;
#16630=CARTESIAN_POINT ( 'NONE',  ( 21.06089410995832623, 10.72529553212358699, -12.20238073104318488 ) ) ;
#16631=EDGE_LOOP ( 'NONE', ( #167766, #53895, #154128, #3294 ) ) ;
#16665=DIRECTION ( 'NONE',  ( -1.000000000000000000, -2.952720810173289112E-16, 0.000000000000000000 ) ) ;
#16670=ORIENTED_EDGE ( 'NONE', *, *, #48135, .F. ) ;
#16689=CARTESIAN_POINT ( 'NONE',  ( 18.59999999999999076, 11.65000000000000391, -24.85000000000000142 ) ) ;
#16715=DIRECTION ( 'NONE',  ( 2.840903330521631775E-16, -0.8700118002898321601, 0.4930308989875230585 ) ) ;
#16734=CARTESIAN_POINT ( 'NONE',  ( 18.48536876927980543, -9.463527249867304647, -7.048618265082689405 ) ) ;
#16751=VECTOR ( 'NONE', #73410, 1000.000000000000000 ) ;
#16790=VERTEX_POINT ( 'NONE', #15211 ) ;
#16797=DIRECTION ( 'NONE',  ( 1.000000000000000000, -0.000000000000000000, -0.000000000000000000 ) ) ;
#16804=AXIS2_PLACEMENT_3D ( 'NONE', #13928, #234235, #16504 ) ;
#16814=CARTESIAN_POINT ( 'NONE',  ( -21.05000000000000071, -11.48912529307605546, -30.50000000000000000 ) ) ;
#16845=CARTESIAN_POINT ( 'NONE',  ( -21.14999999999999858, 11.65000000000000036, -6.783865662978153743 ) ) ;
#16896=CARTESIAN_POINT ( 'NONE',  ( 22.47809213839789066, 0.03753706762852151990, 11.64997333478780206 ) ) ;
#16900=CARTESIAN_POINT ( 'NONE',  ( 20.97107704358301916, 8.875478152021283762, -8.558973229389252424 ) ) ;
#16909=LINE ( 'NONE', #1160, #116888 ) ;
#16915=ORIENTED_EDGE ( 'NONE', *, *, #129763, .T. ) ;
#16920=DIRECTION ( 'NONE',  ( 0.000000000000000000, 0.000000000000000000, -1.000000000000000000 ) ) ;
#16926=CARTESIAN_POINT ( 'NONE',  ( -22.50000000000000000, 0.09263750060947925635, 11.64969720704075051 ) ) ;
#16940=VECTOR ( 'NONE', #33426, 1000.000000000000000 ) ;
#16954=CARTESIAN_POINT ( 'NONE',  ( 18.52928932188133970, 10.27928932188134503, -24.65000000000000213 ) ) ;
#16971=AXIS2_PLACEMENT_3D ( 'NONE', #125223, #243870, #185191 ) ;
#16977=B_SPLINE_CURVE_WITH_KNOTS ( 'NONE', 3,
 ( #120058, #253101, #178758, #176172, #77038, #237410, #177466, #219109, #233568, #114892, #135723, #254373, #75775, #57465, #215275, #40532, #37945, #39233, #58737, #174923, #155336, #35393 ),
 .UNSPECIFIED., .F., .F.,
 ( 4, 3, 3, 3, 3, 3, 3, 4 ),
 ( 0.000000000000000000, 7.307836821079277406E-06, 4.161455748548289888E-05, 7.576591810647585821E-05, 0.0001098090429817541203, 0.0001438003617351132435, 0.0001777914035423700445, 0.0002117966137403027368 ),
 .UNSPECIFIED. ) ;
#16981=ORIENTED_EDGE ( 'NONE', *, *, #9228, .T. ) ;
#16996=ORIENTED_EDGE ( 'NONE', *, *, #206602, .F. ) ;
#17001=AXIS2_PLACEMENT_3D ( 'NONE', #130087, #28476, #225322 ) ;
#17047=CARTESIAN_POINT ( 'NONE',  ( 22.50000000000000000, 7.790779598373383408, 0.09999999999999939493 ) ) ;
#17055=CARTESIAN_POINT ( 'NONE',  ( 21.07928932188134397, 6.328516656393303741, 0.09889514565439641580 ) ) ;
#17057=VERTEX_POINT ( 'NONE', #44599 ) ;
#17093=AXIS2_PLACEMENT_3D ( 'NONE', #54150, #35905, #132423 ) ;
#17098=ADVANCED_FACE ( 'NONE', ( #163428 ), #104685, .T. ) ;
#17130=AXIS2_PLACEMENT_3D ( 'NONE', #241450, #204862, #223144 ) ;
#17135=VERTEX_POINT ( 'NONE', #21364 ) ;
#17140=CIRCLE ( 'NONE', #83709, 0.09999999999999939493 ) ;
#17157=ORIENTED_EDGE ( 'NONE', *, *, #185900, .F. ) ;
#17181=EDGE_CURVE ( 'NONE', #50256, #237441, #182503, .T. ) ;
#17185=CARTESIAN_POINT ( 'NONE',  ( 23.14999999999999858, 0.000000000000000000, 0.000000000000000000 ) ) ;
#17191=ADVANCED_FACE ( 'NONE', ( #181705 ), #160869, .F. ) ;
#17198=AXIS2_PLACEMENT_3D ( 'NONE', #165398, #250063, #186246 ) ;
#17227=DIRECTION ( 'NONE',  ( -0.000000000000000000, -0.000000000000000000, 1.000000000000000000 ) ) ;
#17228=LINE ( 'NONE', #231458, #68608 ) ;
#17257=DIRECTION ( 'NONE',  ( 0.000000000000000000, 0.000000000000000000, -1.000000000000000000 ) ) ;
#17274=AXIS2_PLACEMENT_3D ( 'NONE', #209488, #154685, #12604 ) ;
#17377=( BOUNDED_CURVE ( )  B_SPLINE_CURVE ( 3, ( #125808, #12318, #171408, #247033 ),
 .UNSPECIFIED., .F., .F. ) 
 B_SPLINE_CURVE_WITH_KNOTS ( ( 4, 4 ),
 ( 4.712388980384689674, 6.231880751915386263 ),
 .UNSPECIFIED. ) 
 CURVE ( )  GEOMETRIC_REPRESENTATION_ITEM ( )  RATIONAL_B_SPLINE_CURVE ( ( 1.000000000000000000, 0.8166740347213228279, 0.8166740347213228279, 1.000000000000000000 ) ) 
 REPRESENTATION_ITEM ( '' )  );
#17393=LINE ( 'NONE', #257230, #230458 ) ;
#17431=ORIENTED_EDGE ( 'NONE', *, *, #239855, .F. ) ;
#17444=ORIENTED_EDGE ( 'NONE', *, *, #29263, .F. ) ;
#17448=ORIENTED_EDGE ( 'NONE', *, *, #158154, .F. ) ;
#17450=VECTOR ( 'NONE', #105361, 1000.000000000000000 ) ;
#17474=AXIS2_PLACEMENT_3D ( 'NONE', #171346, #194733, #193441 ) ;
#17481=ORIENTED_EDGE ( 'NONE', *, *, #93584, .T. ) ;
#17483=FACE_OUTER_BOUND ( 'NONE', #76390, .T. ) ;
#17493=DIRECTION ( 'NONE',  ( -1.000000000000000000, 0.000000000000000000, 0.000000000000000000 ) ) ;
#17619=CYLINDRICAL_SURFACE ( 'NONE', #33361, 0.09999999999999939493 ) ;
#17628=ADVANCED_FACE ( 'NONE', ( #108290 ), #185251, .T. ) ;
#17642=DIRECTION ( 'NONE',  ( 1.000000000000000000, 0.000000000000000000, 0.000000000000000000 ) ) ;
#17644=EDGE_LOOP ( 'NONE', ( #66734, #183287, #222633, #77003 ) ) ;
#17648=EDGE_CURVE ( 'NONE', #143516, #9216, #48304, .T. ) ;
#17655=CARTESIAN_POINT ( 'NONE',  ( -20.64999999999999858, 4.349999999999999645, -21.15000000000000213 ) ) ;
#17698=EDGE_CURVE ( 'NONE', #117566, #174236, #190408, .T. ) ;
#17706=ORIENTED_EDGE ( 'NONE', *, *, #108607, .T. ) ;
#17747=EDGE_CURVE ( 'NONE', #255303, #191355, #237887, .T. ) ;
#17754=FACE_OUTER_BOUND ( 'NONE', #119532, .T. ) ;
#17773=DIRECTION ( 'NONE',  ( -1.000000000000000000, -0.000000000000000000, -0.000000000000000000 ) ) ;
#17779=VECTOR ( 'NONE', #250311, 1000.000000000000000 ) ;
#17797=DIRECTION ( 'NONE',  ( 0.000000000000000000, 0.000000000000000000, 1.000000000000000000 ) ) ;
#17806=EDGE_CURVE ( 'NONE', #1674, #172993, #165738, .T. ) ;
#17816=VERTEX_POINT ( 'NONE', #155147 ) ;
#17827=EDGE_LOOP ( 'NONE', ( #138959, #243093, #90552, #143264 ) ) ;
#17842=CARTESIAN_POINT ( 'NONE',  ( -18.59999999999999787, 0.000000000000000000, 0.000000000000000000 ) ) ;
#17846=VERTEX_POINT ( 'NONE', #157726 ) ;
#17869=ORIENTED_EDGE ( 'NONE', *, *, #36400, .F. ) ;
#17883=CARTESIAN_POINT ( 'NONE',  ( 20.97468175916167965, 10.62526516437102231, -12.25476143541283314 ) ) ;
#17895=CARTESIAN_POINT ( 'NONE',  ( -22.50000000000088463, 0.04536165658774753140, 11.65050883420956573 ) ) ;
#17945=CARTESIAN_POINT ( 'NONE',  ( 21.07928932188134397, 6.328516656393312623, 0.09889514565439468108 ) ) ;
#17946=DIRECTION ( 'NONE',  ( 1.000000000000000000, 2.952720810173289112E-16, -0.000000000000000000 ) ) ;
#17947=EDGE_CURVE ( 'NONE', #98230, #108404, #69871, .T. ) ;
#17951=CARTESIAN_POINT ( 'NONE',  ( -20.64999999999999858, 1.999999999999998224, -20.27537807723789953 ) ) ;
#17957=TOROIDAL_SURFACE ( 'NONE', #92983, 4.149999999999999467, 0.1000000000000000056 ) ;
#18094=CYLINDRICAL_SURFACE ( 'NONE', #187059, 0.1000000000000000056 ) ;
#18118=CARTESIAN_POINT ( 'NONE',  ( 18.49999999999999289, 10.20857864376269575, -24.65000000000000213 ) ) ;
#18138=DIRECTION ( 'NONE',  ( 0.000000000000000000, 0.000000000000000000, -1.000000000000000000 ) ) ;
#18139=CARTESIAN_POINT ( 'NONE',  ( 20.85000000000000142, 7.120270961697594103, -37.15956304183931991 ) ) ;
#18141=ORIENTED_EDGE ( 'NONE', *, *, #18501, .F. ) ;
#18150=CYLINDRICAL_SURFACE ( 'NONE', #90685, 0.1000000000000028644 ) ;
#18164=VECTOR ( 'NONE', #149982, 1000.000000000000000 ) ;
#18167=( BOUNDED_SURFACE ( )  B_SPLINE_SURFACE ( 3, 2, ( 
 ( #185028, #205869, #42958 ),
 ( #83327, #2524, #239880 ),
 ( #65078, #143327, #125068 ),
 ( #3824, #144600, #121250 ) ),
 .UNSPECIFIED., .F., .F., .F. ) 
 B_SPLINE_SURFACE_WITH_KNOTS ( ( 4, 4 ),
 ( 3, 3 ),
 ( 0.04058434257139475337, 0.04256401539001600925 ),
 ( 0.000000000000000000, 1.000000000000000000 ),
 .UNSPECIFIED. ) 
 GEOMETRIC_REPRESENTATION_ITEM ( )  RATIONAL_B_SPLINE_SURFACE ( (
 ( 1.000000000000000000, 0.7103081912008133436, 1.000000000000000000),
 ( 1.000000000000000000, 0.7104998333555530010, 1.000000000000000000),
 ( 1.000000000000000000, 0.7107238315755207703, 1.000000000000000000),
 ( 1.000000000000000000, 0.7110073749539380650, 1.000000000000000000) ) ) 
 REPRESENTATION_ITEM ( '' )  SURFACE ( )  );
#18174=ORIENTED_EDGE ( 'NONE', *, *, #251561, .T. ) ;
#18183=EDGE_CURVE ( 'NONE', #240042, #129336, #228269, .T. ) ;
#18195=DIRECTION ( 'NONE',  ( -0.000000000000000000, 1.000000000000000000, 2.891205793294679805E-16 ) ) ;
#18196=CARTESIAN_POINT ( 'NONE',  ( -21.05000000000000071, 0.09779029130879170195, 6.257814610476114758 ) ) ;
#18200=CARTESIAN_POINT ( 'NONE',  ( -18.50000000000000000, 1.866714910057309273, -11.75267524628200633 ) ) ;
#18228=CARTESIAN_POINT ( 'NONE',  ( 18.49999999999999289, 10.24999999999999822, -24.64999999999999503 ) ) ;
#18257=CARTESIAN_POINT ( 'NONE',  ( 23.14999999999999503, 11.65000000000000746, -21.35000000000000142 ) ) ;
#18266=CARTESIAN_POINT ( 'NONE',  ( -23.15000000000000213, 11.65000000000000036, 0.000000000000000000 ) ) ;
#18269=CARTESIAN_POINT ( 'NONE',  ( -21.93642651522410247, 7.327166239325803687, -1.462266042833962457E-16 ) ) ;
#18271=LINE ( 'NONE', #155250, #174817 ) ;
#18274=ORIENTED_EDGE ( 'NONE', *, *, #203063, .F. ) ;
#18289=AXIS2_PLACEMENT_3D ( 'NONE', #237146, #117199, #158914 ) ;
#18301=DIRECTION ( 'NONE',  ( 0.000000000000000000, 0.000000000000000000, -1.000000000000000000 ) ) ;
#18324=ORIENTED_EDGE ( 'NONE', *, *, #245581, .T. ) ;
#18366=DIRECTION ( 'NONE',  ( -1.000000000000000000, -8.673617379884087537E-15, 0.000000000000000000 ) ) ;
#18397=DIRECTION ( 'NONE',  ( -1.000000000000000000, 0.000000000000000000, 0.000000000000000000 ) ) ;
#18401=VERTEX_POINT ( 'NONE', #205461 ) ;
#18480=EDGE_CURVE ( 'NONE', #252532, #220385, #30720, .T. ) ;
#18497=LINE ( 'NONE', #197115, #194620 ) ;
#18501=EDGE_CURVE ( 'NONE', #158940, #29061, #7687, .T. ) ;
#18532=AXIS2_PLACEMENT_3D ( 'NONE', #214749, #16572, #21698 ) ;
#18557=ADVANCED_FACE ( 'NONE', ( #220867 ), #173191, .F. ) ;
#18568=CARTESIAN_POINT ( 'NONE',  ( -18.43707690579160641, -9.682403433476396870, -40.15684337741278398 ) ) ;
#18657=ADVANCED_FACE ( 'NONE', ( #201312 ), #244280, .F. ) ;
#18665=CARTESIAN_POINT ( 'NONE',  ( -21.14999999999999858, 0.000000000000000000, 0.000000000000000000 ) ) ;
#18667=AXIS2_PLACEMENT_3D ( 'NONE', #249573, #128340, #69655 ) ;
#18698=VERTEX_POINT ( 'NONE', #181758 ) ;
#18711=CARTESIAN_POINT ( 'NONE',  ( 23.24999999999999645, 2.100000000000002309, -33.50000000000000000 ) ) ;
#18726=ORIENTED_EDGE ( 'NONE', *, *, #245976, .F. ) ;
#18735=CIRCLE ( 'NONE', #152032, 0.1999999999999987899 ) ;
#18748=DIRECTION ( 'NONE',  ( 0.000000000000000000, -0.000000000000000000, 1.000000000000000000 ) ) ;
#18750=DIRECTION ( 'NONE',  ( 0.000000000000000000, 2.664535259100376486E-15, -1.000000000000000000 ) ) ;
#18759=AXIS2_PLACEMENT_3D ( 'NONE', #196444, #197733, #257641 ) ;
#18766=VERTEX_POINT ( 'NONE', #216402 ) ;
#18779=ORIENTED_EDGE ( 'NONE', *, *, #225541, .T. ) ;
#18784=CARTESIAN_POINT ( 'NONE',  ( 21.14261333020286671, 10.71569264925490650, -12.25000000000021316 ) ) ;
#18792=VECTOR ( 'NONE', #141538, 1000.000000000000000 ) ;
#18797=AXIS2_PLACEMENT_3D ( 'NONE', #251010, #72420, #254825 ) ;
#18838=ADVANCED_FACE ( 'NONE', ( #157773 ), #237265, .T. ) ;
#18844=EDGE_LOOP ( 'NONE', ( #60694, #136667, #223098, #9010 ) ) ;
#18854=LINE ( 'NONE', #176669, #13055 ) ;
#18871=DIRECTION ( 'NONE',  ( 1.000000000000000000, 0.000000000000000000, 0.000000000000000000 ) ) ;
#18872=DIRECTION ( 'NONE',  ( 1.000000000000000000, 0.000000000000000000, -0.000000000000000000 ) ) ;
#18921=EDGE_LOOP ( 'NONE', ( #212775, #154333, #199069, #61402 ) ) ;
#18937=EDGE_CURVE ( 'NONE', #112246, #233645, #112118, .T. ) ;
#19045=ORIENTED_EDGE ( 'NONE', *, *, #78182, .F. ) ;
#19048=ADVANCED_FACE ( 'NONE', ( #8918 ), #235279, .F. ) ;
#19103=EDGE_CURVE ( 'NONE', #102134, #217631, #145397, .T. ) ;
#19136=FACE_OUTER_BOUND ( 'NONE', #83859, .T. ) ;
#19173=EDGE_CURVE ( 'NONE', #164389, #79953, #95346, .T. ) ;
#19245=EDGE_CURVE ( 'NONE', #62135, #138031, #63428, .T. ) ;
#19256=EDGE_CURVE ( 'NONE', #210177, #144164, #42592, .T. ) ;
#19267=AXIS2_PLACEMENT_3D ( 'NONE', #237610, #202324, #121541 ) ;
#19273=CARTESIAN_POINT ( 'NONE',  ( 22.50000000000000000, 0.1008583690987118059, 11.74956712348939369 ) ) ;
#19282=CARTESIAN_POINT ( 'NONE',  ( -18.59999999999999787, 9.350000000000001421, -21.15000000000000213 ) ) ;
#19306=CARTESIAN_POINT ( 'NONE',  ( -21.05000000000000071, 11.64999999999999680, -6.783865662978152855 ) ) ;
#19312=CARTESIAN_POINT ( 'NONE',  ( -21.05000000000000071, 11.64999999999999680, -6.783865662978151967 ) ) ;
#19329=CARTESIAN_POINT ( 'NONE',  ( -23.25000000000000000, -9.000000000000001776, -23.60603087734756045 ) ) ;
#19355=ORIENTED_EDGE ( 'NONE', *, *, #236335, .F. ) ;
#19359=EDGE_CURVE ( 'NONE', #178493, #101170, #175316, .T. ) ;
#19372=CARTESIAN_POINT ( 'NONE',  ( -21.08198257630413508, 0.07264332378459012474, 6.336596734015067511 ) ) ;
#19413=DIRECTION ( 'NONE',  ( 0.000000000000000000, -0.000000000000000000, 1.000000000000000000 ) ) ;
#19425=EDGE_CURVE ( 'NONE', #193155, #61614, #29570, .T. ) ;
#19445=DIRECTION ( 'NONE',  ( 1.000000000000000000, 3.265361837132813093E-16, -0.000000000000000000 ) ) ;
#19451=EDGE_CURVE ( 'NONE', #97347, #184180, #208625, .T. ) ;
#19453=VERTEX_POINT ( 'NONE', #146809 ) ;
#19471=VECTOR ( 'NONE', #65075, 1000.000000000000000 ) ;
#19491=CARTESIAN_POINT ( 'NONE',  ( -21.05000000000000426, -0.02103547654011232379, 6.304455821947658301 ) ) ;
#19522=CIRCLE ( 'NONE', #161159, 0.09999999999999949207 ) ;
#19560=LINE ( 'NONE', #219022, #124397 ) ;
#19587=CARTESIAN_POINT ( 'NONE',  ( -20.94999999999999929, -1.164121893241208960, -41.21484808557161017 ) ) ;
#19601=ORIENTED_EDGE ( 'NONE', *, *, #221247, .T. ) ;
#19625=LINE ( 'NONE', #159155, #93448 ) ;
#19665=DIRECTION ( 'NONE',  ( 0.000000000000000000, 0.000000000000000000, -1.000000000000000000 ) ) ;
#19688=VERTEX_POINT ( 'NONE', #80082 ) ;
#19693=ORIENTED_EDGE ( 'NONE', *, *, #104664, .F. ) ;
#19699=DIRECTION ( 'NONE',  ( -0.000000000000000000, -0.000000000000000000, -1.000000000000000000 ) ) ;
#19733=VERTEX_POINT ( 'NONE', #8315 ) ;
#19774=AXIS2_PLACEMENT_3D ( 'NONE', #135705, #255617, #173622 ) ;
#19797=FACE_OUTER_BOUND ( 'NONE', #164616, .T. ) ;
#19816=ADVANCED_FACE ( 'NONE', ( #89112 ), #146235, .F. ) ;
#19817=ORIENTED_EDGE ( 'NONE', *, *, #6203, .F. ) ;
#19829=VECTOR ( 'NONE', #223999, 1000.000000000000000 ) ;
#19852=DIRECTION ( 'NONE',  ( 0.000000000000000000, 0.000000000000000000, -1.000000000000000000 ) ) ;
#19864=CARTESIAN_POINT ( 'NONE',  ( -21.05000000000000071, -11.75000000000000000, -30.39999999999999503 ) ) ;
#19906=AXIS2_PLACEMENT_3D ( 'NONE', #178875, #197101, #156737 ) ;
#19914=CARTESIAN_POINT ( 'NONE',  ( 18.60000000000000142, -9.321008403361283001, -7.235938249077890738 ) ) ;
#19926=ORIENTED_EDGE ( 'NONE', *, *, #203042, .F. ) ;
#19931=DIRECTION ( 'NONE',  ( -3.469446951953635015E-14, 1.000000000000000000, 0.000000000000000000 ) ) ;
#19935=VECTOR ( 'NONE', #249863, 1000.000000000000000 ) ;
#19944=EDGE_CURVE ( 'NONE', #180003, #51281, #108817, .T. ) ;
#19972=CARTESIAN_POINT ( 'NONE',  ( -21.14999999999999858, 0.000000000000000000, 0.000000000000000000 ) ) ;
#19981=AXIS2_PLACEMENT_3D ( 'NONE', #10145, #225312, #230476 ) ;
#19986=EDGE_CURVE ( 'NONE', #41654, #72182, #216956, .T. ) ;
#20087=DIRECTION ( 'NONE',  ( 0.000000000000000000, 0.000000000000000000, 1.000000000000000000 ) ) ;
#20093=CARTESIAN_POINT ( 'NONE',  ( -21.14999999999999858, 0.000000000000000000, 6.540656951701240729 ) ) ;
#20120=ORIENTED_EDGE ( 'NONE', *, *, #92904, .F. ) ;
#20123=CARTESIAN_POINT ( 'NONE',  ( -22.47007471830798409, 1.829591166069288732E-15, 7.720710651926479429 ) ) ;
#20133=ORIENTED_EDGE ( 'NONE', *, *, #241622, .T. ) ;
#20193=ADVANCED_FACE ( 'NONE', ( #244022 ), #157159, .T. ) ;
#20235=EDGE_CURVE ( 'NONE', #70460, #49525, #169661, .T. ) ;
#20237=SPHERICAL_SURFACE ( 'NONE', #205696, 0.1000000000000000056 ) ;
#20239=AXIS2_PLACEMENT_3D ( 'NONE', #203773, #9413, #225869 ) ;
#20264=AXIS2_PLACEMENT_3D ( 'NONE', #93225, #211916, #232762 ) ;
#20289=CIRCLE ( 'NONE', #149476, 0.09999999999999910349 ) ;
#20290=ADVANCED_FACE ( 'NONE', ( #71836 ), #92655, .F. ) ;
#20292=DIRECTION ( 'NONE',  ( 0.000000000000000000, 2.168404344971003346E-15, 1.000000000000000000 ) ) ;
#20312=AXIS2_PLACEMENT_3D ( 'NONE', #61417, #194533, #123974 ) ;
#20317=CIRCLE ( 'NONE', #41174, 0.09999999999999939493 ) ;
#20319=DIRECTION ( 'NONE',  ( 0.000000000000000000, -0.000000000000000000, -1.000000000000000000 ) ) ;
#20330=CARTESIAN_POINT ( 'NONE',  ( -23.15000000000000213, 0.000000000000000000, -31.50000000000000000 ) ) ;
#20344=ORIENTED_EDGE ( 'NONE', *, *, #171742, .T. ) ;
#20352=ORIENTED_EDGE ( 'NONE', *, *, #131304, .T. ) ;
#20384=CARTESIAN_POINT ( 'NONE',  ( 20.95512820512820440, 8.876151316288115822, -8.558628995140949769 ) ) ;
#20392=DIRECTION ( 'NONE',  ( -1.000000000000000000, 0.000000000000000000, 0.000000000000000000 ) ) ;
#20412=AXIS2_PLACEMENT_3D ( 'NONE', #95521, #265, #158115 ) ;
#20421=ORIENTED_EDGE ( 'NONE', *, *, #151334, .F. ) ;
#20422=CARTESIAN_POINT ( 'NONE',  ( -22.39999999999999858, 0.000000000000000000, 0.000000000000000000 ) ) ;
#20460=ADVANCED_FACE ( 'NONE', ( #158318 ), #193890, .F. ) ;
#20483=DIRECTION ( 'NONE',  ( -1.000000000000000000, -7.304098846218134667E-16, 0.000000000000000000 ) ) ;
#20485=ORIENTED_EDGE ( 'NONE', *, *, #15958, .F. ) ;
#20511=EDGE_CURVE ( 'NONE', #216880, #138911, #218228, .T. ) ;
#20543=EDGE_CURVE ( 'NONE', #104459, #169470, #124018, .T. ) ;
#20563=ORIENTED_EDGE ( 'NONE', *, *, #234296, .T. ) ;
#20565=VERTEX_POINT ( 'NONE', #257235 ) ;
#20578=VECTOR ( 'NONE', #31177, 1000.000000000000000 ) ;
#20594=AXIS2_PLACEMENT_3D ( 'NONE', #41591, #97659, #160258 ) ;
#20596=CARTESIAN_POINT ( 'NONE',  ( 23.15000000000000213, -9.599999999999999645, -23.60603087734755690 ) ) ;
#20612=CIRCLE ( 'NONE', #53347, 7.720710678118680725 ) ;
#20677=CARTESIAN_POINT ( 'NONE',  ( -18.59999999999999787, -1.162701749938009677, -8.099999999999999645 ) ) ;
#20703=ORIENTED_EDGE ( 'NONE', *, *, #131224, .T. ) ;
#20740=CARTESIAN_POINT ( 'NONE',  ( 18.59999999999997655, -1.164121893241208960, -41.41484808557160591 ) ) ;
#20756=CARTESIAN_POINT ( 'NONE',  ( 20.84451136049667852, 10.62014191480694159, -7.493924559529303586 ) ) ;
#20771=EDGE_CURVE ( 'NONE', #61614, #193155, #153455, .T. ) ;
#20777=CARTESIAN_POINT ( 'NONE',  ( 18.59999999999999787, 5.899999999999947065, -10.21909976465641456 ) ) ;
#20780=CARTESIAN_POINT ( 'NONE',  ( -20.64999999999999858, 4.349999999999999645, -21.15000000000000213 ) ) ;
#20790=CIRCLE ( 'NONE', #124817, 0.1999999999999996503 ) ;
#20804=ORIENTED_EDGE ( 'NONE', *, *, #205044, .F. ) ;
#20836=VERTEX_POINT ( 'NONE', #38914 ) ;
#20845=ADVANCED_FACE ( 'NONE', ( #140551 ), #139254, .T. ) ;
#20867=DIRECTION ( 'NONE',  ( 0.000000000000000000, 8.881784197001252323E-16, -1.000000000000000000 ) ) ;
#20880=CARTESIAN_POINT ( 'NONE',  ( -20.94999999999999929, -1.360870587192041681, -8.072997927090961312 ) ) ;
#20887=VERTEX_POINT ( 'NONE', #217516 ) ;
#20895=FACE_OUTER_BOUND ( 'NONE', #244866, .T. ) ;
#20899=CARTESIAN_POINT ( 'NONE',  ( 21.05000000000000071, 10.72371710470752149, -12.15000000000000036 ) ) ;
#20958=ORIENTED_EDGE ( 'NONE', *, *, #187590, .F. ) ;
#20971=PLANE ( 'NONE',  #14189 ) ;
#21044=CARTESIAN_POINT ( 'NONE',  ( -23.25000000000000000, 1.999999999999998224, -20.27537807723789953 ) ) ;
#21063=AXIS2_PLACEMENT_3D ( 'NONE', #161279, #115720, #158727 ) ;
#21066=AXIS2_PLACEMENT_3D ( 'NONE', #70792, #206419, #189436 ) ;
#21083=FACE_OUTER_BOUND ( 'NONE', #182762, .T. ) ;
#21091=PLANE ( 'NONE',  #36393 ) ;
#21092=DIRECTION ( 'NONE',  ( 0.000000000000000000, 1.000000000000000000, 0.000000000000000000 ) ) ;
#21114=AXIS2_PLACEMENT_3D ( 'NONE', #65274, #186520, #183942 ) ;
#21125=ADVANCED_FACE ( 'NONE', ( #36036 ), #179399, .F. ) ;
#21131=CARTESIAN_POINT ( 'NONE',  ( 21.05000000000000071, -11.48912529307605901, -3.100000000000000533 ) ) ;
#21152=PLANE ( 'NONE',  #90172 ) ;
#21160=CARTESIAN_POINT ( 'NONE',  ( 21.08489834409762054, 10.62232389473552097, -12.35000000000000320 ) ) ;
#21214=CARTESIAN_POINT ( 'NONE',  ( 18.60000000000000853, -9.364236010366765228, -7.180254400724614072 ) ) ;
#21240=DIRECTION ( 'NONE',  ( 0.000000000000000000, -1.000000000000000000, 0.000000000000000000 ) ) ;
#21318=ORIENTED_EDGE ( 'NONE', *, *, #11560, .T. ) ;
#21324=DIRECTION ( 'NONE',  ( 1.000000000000000000, -0.000000000000000000, -0.000000000000000000 ) ) ;
#21327=CARTESIAN_POINT ( 'NONE',  ( -20.94999999999999929, -11.48912529307605546, -30.39999999999999503 ) ) ;
#21342=ORIENTED_EDGE ( 'NONE', *, *, #183289, .T. ) ;
#21351=CIRCLE ( 'NONE', #42018, 0.09999999999999939493 ) ;
#21364=CARTESIAN_POINT ( 'NONE',  ( -20.94999999999999929, -11.65000000000000036, -3.000000000000002665 ) ) ;
#21430=CARTESIAN_POINT ( 'NONE',  ( -21.45000000000000284, 7.708578643762696636, -21.15000000000000213 ) ) ;
#21434=SPHERICAL_SURFACE ( 'NONE', #33658, 0.1000000000000000056 ) ;
#21440=ORIENTED_EDGE ( 'NONE', *, *, #31507, .F. ) ;
#21485=CARTESIAN_POINT ( 'NONE',  ( -21.05000000000000071, -1.851028230140860487, -11.65391326942249428 ) ) ;
#21535=DIRECTION ( 'NONE',  ( -1.000000000000000000, 9.012599976028471648E-15, 6.882867235861662930E-14 ) ) ;
#21552=DIRECTION ( 'NONE',  ( 1.000000000000000000, -0.000000000000000000, -0.000000000000000000 ) ) ;
#21605=LINE ( 'NONE', #209210, #217717 ) ;
#21611=ORIENTED_EDGE ( 'NONE', *, *, #44350, .F. ) ;
#21615=FACE_OUTER_BOUND ( 'NONE', #158364, .T. ) ;
#21643=CARTESIAN_POINT ( 'NONE',  ( -21.05000000000000071, 11.65000000000000036, -26.48519422934605316 ) ) ;
#21698=DIRECTION ( 'NONE',  ( 0.000000000000000000, 0.000000000000000000, -1.000000000000000000 ) ) ;
#21714=DIRECTION ( 'NONE',  ( 1.000000000000000000, -7.304098846218135653E-16, 0.000000000000000000 ) ) ;
#21717=VECTOR ( 'NONE', #179755, 1000.000000000000000 ) ;
#21758=EDGE_CURVE ( 'NONE', #68838, #253474, #157525, .T. ) ;
#21769=DIRECTION ( 'NONE',  ( 0.000000000000000000, -1.000000000000000000, 0.000000000000000000 ) ) ;
#21771=ORIENTED_EDGE ( 'NONE', *, *, #133585, .T. ) ;
#21776=ADVANCED_FACE ( 'NONE', ( #52389 ), #69422, .T. ) ;
#21798=ORIENTED_EDGE ( 'NONE', *, *, #49334, .T. ) ;
#21852=ORIENTED_EDGE ( 'NONE', *, *, #241196, .T. ) ;
#21888=EDGE_LOOP ( 'NONE', ( #90002, #45657, #51790, #117778 ) ) ;
#21912=DIRECTION ( 'NONE',  ( 0.000000000000000000, 1.000000000000000000, 0.000000000000000000 ) ) ;
#21925=EDGE_CURVE ( 'NONE', #144336, #187076, #170014, .T. ) ;
#21931=DIRECTION ( 'NONE',  ( 0.000000000000000000, 0.000000000000000000, 1.000000000000000000 ) ) ;
#21944=CARTESIAN_POINT ( 'NONE',  ( -21.08621493067320429, 0.05619483947604889812, 6.349294291171942106 ) ) ;
#22009=ADVANCED_FACE ( 'NONE', ( #252141 ), #214317, .F. ) ;
#22023=CARTESIAN_POINT ( 'NONE',  ( -20.54999999999999716, 1.999999999999998224, -20.67537807723790166 ) ) ;
#22057=VERTEX_POINT ( 'NONE', #89220 ) ;
#22064=EDGE_CURVE ( 'NONE', #158940, #106265, #230019, .T. ) ;
#22067=DIRECTION ( 'NONE',  ( 0.000000000000000000, 0.000000000000000000, 1.000000000000000000 ) ) ;
#22071=DIRECTION ( 'NONE',  ( -1.000000000000000000, -2.952720810173289112E-16, 0.000000000000000000 ) ) ;
#22087=EDGE_CURVE ( 'NONE', #199662, #219323, #149335, .T. ) ;
#22106=DIRECTION ( 'NONE',  ( 1.000000000000000000, -0.000000000000000000, 0.000000000000000000 ) ) ;
#22130=CIRCLE ( 'NONE', #72006, 0.09999999999999999167 ) ;
#22145=CARTESIAN_POINT ( 'NONE',  ( -21.05000000000000071, 0.000000000000000000, 0.000000000000000000 ) ) ;
#22223=ORIENTED_EDGE ( 'NONE', *, *, #112310, .F. ) ;
#22230=CARTESIAN_POINT ( 'NONE',  ( 21.78635804494511419, 0.09900506550768010949, 7.035661485153183570 ) ) ;
#22238=ORIENTED_EDGE ( 'NONE', *, *, #116565, .F. ) ;
#22267=ORIENTED_EDGE ( 'NONE', *, *, #233995, .F. ) ;
#22292=VECTOR ( 'NONE', #205082, 1000.000000000000000 ) ;
#22297=AXIS2_PLACEMENT_3D ( 'NONE', #211759, #112655, #189630 ) ;
#22302=ORIENTED_EDGE ( 'NONE', *, *, #214526, .T. ) ;
#22320=AXIS2_PLACEMENT_3D ( 'NONE', #122008, #179430, #257598 ) ;
#22344=VECTOR ( 'NONE', #252161, 1000.000000000000000 ) ;
#22345=CIRCLE ( 'NONE', #26428, 0.1000000000000016431 ) ;
#22380=CARTESIAN_POINT ( 'NONE',  ( -20.54999999999999716, 4.349999999999999645, -16.75000000000000000 ) ) ;
#22413=TOROIDAL_SURFACE ( 'NONE', #18289, 0.2000000000000000111, 0.1000000000000000056 ) ;
#22482=ORIENTED_EDGE ( 'NONE', *, *, #29671, .T. ) ;
#22502=ADVANCED_FACE ( 'NONE', ( #238584 ), #15721, .F. ) ;
#22517=DIRECTION ( 'NONE',  ( 0.000000000000000000, 0.000000000000000000, -1.000000000000000000 ) ) ;
#22539=ORIENTED_EDGE ( 'NONE', *, *, #108607, .F. ) ;
#22570=VECTOR ( 'NONE', #239752, 1000.000000000000000 ) ;
#22608=ORIENTED_EDGE ( 'NONE', *, *, #119729, .F. ) ;
#22632=AXIS2_PLACEMENT_3D ( 'NONE', #253243, #211570, #232433 ) ;
#22649=DIRECTION ( 'NONE',  ( 1.000000000000000000, 0.000000000000000000, 0.000000000000000000 ) ) ;
#22674=LINE ( 'NONE', #80014, #116616 ) ;
#22694=CARTESIAN_POINT ( 'NONE',  ( -20.99551997958405991, 11.75000000000017941, -26.65165913768950290 ) ) ;
#22768=DIRECTION ( 'NONE',  ( 0.000000000000000000, -1.000000000000000000, 0.000000000000000000 ) ) ;
#22786=DIRECTION ( 'NONE',  ( 0.000000000000000000, -1.000000000000000000, -0.000000000000000000 ) ) ;
#22823=ORIENTED_EDGE ( 'NONE', *, *, #224414, .F. ) ;
#22825=CIRCLE ( 'NONE', #147706, 12.87500000000000000 ) ;
#22830=CARTESIAN_POINT ( 'NONE',  ( 18.50000324121758055, 10.29307482167976318, -38.95864214669396119 ) ) ;
#22835=CARTESIAN_POINT ( 'NONE',  ( 20.85000000000000142, -1.851617760468904805, -45.10318971960366241 ) ) ;
#22839=DIRECTION ( 'NONE',  ( 0.000000000000000000, -1.000000000000000000, 0.000000000000000000 ) ) ;
#22840=CIRCLE ( 'NONE', #135230, 0.09999999999999939493 ) ;
#22857=CIRCLE ( 'NONE', #81072, 0.1000000000000007133 ) ;
#22875=ORIENTED_EDGE ( 'NONE', *, *, #163616, .F. ) ;
#22987=CARTESIAN_POINT ( 'NONE',  ( -20.54999999999999716, 1.940186915887853303, -12.82911921105332631 ) ) ;
#22996=DIRECTION ( 'NONE',  ( 0.000000000000000000, -0.9999631594459056361, -0.008583690987124413183 ) ) ;
#22999=EDGE_LOOP ( 'NONE', ( #29684, #57804, #81188, #28338 ) ) ;
#23006=AXIS2_PLACEMENT_3D ( 'NONE', #83055, #60957, #183488 ) ;
#23031=AXIS2_PLACEMENT_3D ( 'NONE', #203222, #181116, #77170 ) ;
#23044=AXIS2_PLACEMENT_3D ( 'NONE', #13594, #50127, #111403 ) ;
#23058=CARTESIAN_POINT ( 'NONE',  ( 23.24999999999999289, 11.75000000000000711, -12.15000000000000036 ) ) ;
#23078=DIRECTION ( 'NONE',  ( 0.000000000000000000, -1.000000000000000000, 0.000000000000000000 ) ) ;
#23099=LINE ( 'NONE', #63472, #160353 ) ;
#23122=EDGE_LOOP ( 'NONE', ( #157606, #222379, #62144, #94582 ) ) ;
#23126=ORIENTED_EDGE ( 'NONE', *, *, #104446, .T. ) ;
#23165=DIRECTION ( 'NONE',  ( 0.000000000000000000, 0.4999999999999929501, -0.8660254037844427044 ) ) ;
#23168=ORIENTED_EDGE ( 'NONE', *, *, #59914, .T. ) ;
#23180=CARTESIAN_POINT ( 'NONE',  ( -20.94684162621883061, 11.74999999999999467, -6.841644000359353939 ) ) ;
#23200=ORIENTED_EDGE ( 'NONE', *, *, #187309, .F. ) ;
#23203=SPHERICAL_SURFACE ( 'NONE', #236233, 0.1000000000000000056 ) ;
#23224=TOROIDAL_SURFACE ( 'NONE', #189796, 0.2000000000000000111, 0.1000000000000000056 ) ;
#23228=DIRECTION ( 'NONE',  ( 0.000000000000000000, 0.000000000000000000, -1.000000000000000000 ) ) ;
#23231=CARTESIAN_POINT ( 'NONE',  ( 20.95512820512820795, 8.876151316288117599, -12.20017285912874883 ) ) ;
#23245=VERTEX_POINT ( 'NONE', #54186 ) ;
#23263=ADVANCED_FACE ( 'NONE', ( #178017 ), #17619, .T. ) ;
#23278=ORIENTED_EDGE ( 'NONE', *, *, #166741, .T. ) ;
#23280=ORIENTED_EDGE ( 'NONE', *, *, #230827, .T. ) ;
#23324=ORIENTED_EDGE ( 'NONE', *, *, #111867, .F. ) ;
#23334=CARTESIAN_POINT ( 'NONE',  ( 21.14999999999999858, 11.65000000000000391, -0.1000000000000028644 ) ) ;
#23356=ORIENTED_EDGE ( 'NONE', *, *, #137013, .F. ) ;
#23368=EDGE_CURVE ( 'NONE', #214472, #109031, #208302, .T. ) ;
#23397=EDGE_LOOP ( 'NONE', ( #77009, #81858, #13393, #39493 ) ) ;
#23400=EDGE_CURVE ( 'NONE', #56194, #224530, #220759, .T. ) ;
#23469=EDGE_LOOP ( 'NONE', ( #138010, #2053, #122836, #34254 ) ) ;
#23478=DIRECTION ( 'NONE',  ( 0.000000000000000000, 1.000000000000000000, 0.000000000000000000 ) ) ;
#23489=CARTESIAN_POINT ( 'NONE',  ( 23.15000000000000213, -11.64999999999999147, -30.39999999999999503 ) ) ;
#23516=VECTOR ( 'NONE', #182828, 1000.000000000000000 ) ;
#23534=DIRECTION ( 'NONE',  ( -1.000000000000000000, -0.000000000000000000, 0.000000000000000000 ) ) ;
#23538=EDGE_CURVE ( 'NONE', #23245, #47350, #68333, .T. ) ;
#23546=ORIENTED_EDGE ( 'NONE', *, *, #230789, .F. ) ;
#23612=ORIENTED_EDGE ( 'NONE', *, *, #216250, .T. ) ;
#23617=CIRCLE ( 'NONE', #169368, 4.149999999999999467 ) ;
#23635=CARTESIAN_POINT ( 'NONE',  ( -23.15000000000000213, 11.65000000000000036, -26.48519422934605672 ) ) ;
#23658=DIRECTION ( 'NONE',  ( -1.000000000000000000, 0.000000000000000000, 0.000000000000000000 ) ) ;
#23682=ORIENTED_EDGE ( 'NONE', *, *, #118094, .T. ) ;
#23685=EDGE_CURVE ( 'NONE', #166580, #228001, #59964, .T. ) ;
#23695=CIRCLE ( 'NONE', #102931, 0.09999999999999999167 ) ;
#23701=VERTEX_POINT ( 'NONE', #198210 ) ;
#23714=CARTESIAN_POINT ( 'NONE',  ( -21.05000000000000071, 0.000000000000000000, -33.50000000000000000 ) ) ;
#23715=AXIS2_PLACEMENT_3D ( 'NONE', #199975, #184244, #164692 ) ;
#23796=AXIS2_PLACEMENT_3D ( 'NONE', #187888, #168358, #47056 ) ;
#23798=AXIS2_PLACEMENT_3D ( 'NONE', #61796, #1800, #145163 ) ;
#23819=AXIS2_PLACEMENT_3D ( 'NONE', #148198, #90777, #128653 ) ;
#23849=CARTESIAN_POINT ( 'NONE',  ( 22.50000000000000000, 0.09999999999999939493, 7.790779598373383408 ) ) ;
#23874=AXIS2_PLACEMENT_3D ( 'NONE', #37333, #253774, #256287 ) ;
#23893=ORIENTED_EDGE ( 'NONE', *, *, #105148, .F. ) ;
#23894=AXIS2_PLACEMENT_3D ( 'NONE', #38045, #215363, #77138 ) ;
#23898=ORIENTED_EDGE ( 'NONE', *, *, #32116, .F. ) ;
#23920=CARTESIAN_POINT ( 'NONE',  ( -23.15000000000000213, 0.000000000000000000, -33.50000000000000000 ) ) ;
#23925=CARTESIAN_POINT ( 'NONE',  ( -20.64999999999999858, -9.400000000000002132, -23.60603087734756045 ) ) ;
#23928=DIRECTION ( 'NONE',  ( 1.000000000000000000, 3.265361837132813093E-16, -0.000000000000000000 ) ) ;
#23936=CARTESIAN_POINT ( 'NONE',  ( 21.14999999999999858, -0.09999999999999939493, 0.000000000000000000 ) ) ;
#23939=EDGE_LOOP ( 'NONE', ( #100458, #198427, #257947, #205974, #37849, #139673, #114242, #143402, #80822, #197168, #206052, #132137 ) ) ;
#23958=FACE_OUTER_BOUND ( 'NONE', #215628, .T. ) ;
#23968=CIRCLE ( 'NONE', #11495, 0.09999999999999939493 ) ;
#23973=CARTESIAN_POINT ( 'NONE',  ( 20.85000000000000142, -11.64999999999999147, -33.50000000000000000 ) ) ;
#23981=ORIENTED_EDGE ( 'NONE', *, *, #38248, .T. ) ;
#23992=EDGE_CURVE ( 'NONE', #122268, #113211, #212584, .T. ) ;
#24017=AXIS2_PLACEMENT_3D ( 'NONE', #37885, #79531, #117398 ) ;
#24031=DIRECTION ( 'NONE',  ( 0.000000000000000000, 0.000000000000000000, -1.000000000000000000 ) ) ;
#24032=CARTESIAN_POINT ( 'NONE',  ( -18.59999999999999787, -1.637172712970379918, -11.58215336547201701 ) ) ;
#24036=ORIENTED_EDGE ( 'NONE', *, *, #71783, .F. ) ;
#24041=EDGE_LOOP ( 'NONE', ( #76796, #232849, #228378, #112131 ) ) ;
#24081=DIRECTION ( 'NONE',  ( -1.000000000000000000, 0.000000000000000000, 0.000000000000000000 ) ) ;
#24110=AXIS2_PLACEMENT_3D ( 'NONE', #119226, #115356, #158379 ) ;
#24118=CARTESIAN_POINT ( 'NONE',  ( -23.25000000000000000, -1.851617760468904805, -45.10318971960366241 ) ) ;
#24140=AXIS2_PLACEMENT_3D ( 'NONE', #89735, #169331, #134003 ) ;
#24147=EDGE_LOOP ( 'NONE', ( #140484, #13528, #248617, #230484 ) ) ;
#24163=EDGE_CURVE ( 'NONE', #234900, #49525, #249260, .T. ) ;
#24200=CARTESIAN_POINT ( 'NONE',  ( 23.15000000000000213, -9.500000000000001776, -9.893969122652443104 ) ) ;
#24202=ADVANCED_FACE ( 'NONE', ( #173623 ), #216539, .T. ) ;
#24210=APPLICATION_CONTEXT ( 'automotive_design' ) ;
#24235=CIRCLE ( 'NONE', #36725, 0.1000000000000028644 ) ;
#24242=EDGE_LOOP ( 'NONE', ( #240204, #192585, #189296, #207550 ) ) ;
#24243=AXIS2_PLACEMENT_3D ( 'NONE', #36360, #254082, #96285 ) ;
#24262=VERTEX_POINT ( 'NONE', #14522 ) ;
#24291=VERTEX_POINT ( 'NONE', #58724 ) ;
#24314=CARTESIAN_POINT ( 'NONE',  ( 18.59999999999998721, 19.85039924723355398, -2.280303057801358335 ) ) ;
#24331=CARTESIAN_POINT ( 'NONE',  ( -20.64999999999999858, 7.150000000000000355, -21.15000000000000213 ) ) ;
#24358=CARTESIAN_POINT ( 'NONE',  ( -21.05000000000000071, 1.835341550224411922, -11.55515129256298046 ) ) ;
#24360=CARTESIAN_POINT ( 'NONE',  ( 22.49806830649814060, 11.64988965483908068, 0.07746431632550301871 ) ) ;
#24368=DIRECTION ( 'NONE',  ( 0.000000000000000000, 0.1350103645451876666, 0.9908441862701600211 ) ) ;
#24370=AXIS2_PLACEMENT_3D ( 'NONE', #152509, #251570, #110775 ) ;
#24382=CARTESIAN_POINT ( 'NONE',  ( -18.50000000000000355, -9.399999999999973710, -7.297259759663287326 ) ) ;
#24389=AXIS2_PLACEMENT_3D ( 'NONE', #130740, #171201, #125598 ) ;
#24393=VECTOR ( 'NONE', #35684, 1000.000000000000000 ) ;
#24411=VECTOR ( 'NONE', #9302, 1000.000000000000000 ) ;
#24412=ORIENTED_EDGE ( 'NONE', *, *, #10190, .F. ) ;
#24414=AXIS2_PLACEMENT_3D ( 'NONE', #179916, #114788, #217716 ) ;
#24415=CIRCLE ( 'NONE', #57703, 0.09999999999999892308 ) ;
#24429=CYLINDRICAL_SURFACE ( 'NONE', #208479, 0.09999999999999939493 ) ;
#24442=AXIS2_PLACEMENT_3D ( 'NONE', #98048, #118950, #19852 ) ;
#24450=AXIS2_PLACEMENT_3D ( 'NONE', #200536, #21912, #254081 ) ;
#24461=DIRECTION ( 'NONE',  ( -0.000000000000000000, -0.000000000000000000, -1.000000000000000000 ) ) ;
#24546=CARTESIAN_POINT ( 'NONE',  ( -22.00356870141645871, 7.254242362487164364, -2.206487650916222969E-12 ) ) ;
#24548=DIRECTION ( 'NONE',  ( 0.000000000000000000, 0.000000000000000000, -1.000000000000000000 ) ) ;
#24566=DIRECTION ( 'NONE',  ( -2.578261006436900068E-14, 0.1350103645451904977, -0.9908441862701597991 ) ) ;
#24569=CARTESIAN_POINT ( 'NONE',  ( -20.54999999999999716, -9.000000000000001776, -24.00603087734755903 ) ) ;
#24655=CIRCLE ( 'NONE', #16264, 0.09999999999999939493 ) ;
#24681=ORIENTED_EDGE ( 'NONE', *, *, #171742, .F. ) ;
#24689=CIRCLE ( 'NONE', #37322, 0.09999999999999939493 ) ;
#24707=CARTESIAN_POINT ( 'NONE',  ( -20.64999999999999858, 0.000000000000000000, 0.000000000000000000 ) ) ;
#24708=DIRECTION ( 'NONE',  ( -1.000000000000000000, -2.952720810173289112E-16, 0.000000000000000000 ) ) ;
#24719=CIRCLE ( 'NONE', #74606, 12.97499999999999964 ) ;
#24724=FACE_OUTER_BOUND ( 'NONE', #163104, .T. ) ;
#24742=ADVANCED_FACE ( 'NONE', ( #42727 ), #63832, .F. ) ;
#24753=ORIENTED_EDGE ( 'NONE', *, *, #123184, .T. ) ;
#24783=FACE_OUTER_BOUND ( 'NONE', #225504, .T. ) ;
#24799=AXIS2_PLACEMENT_3D ( 'NONE', #17842, #159961, #59515 ) ;
#24813=CARTESIAN_POINT ( 'NONE',  ( 21.07928932188134397, 0.09889514565439641580, 6.328516656393307294 ) ) ;
#24883=ORIENTED_EDGE ( 'NONE', *, *, #757, .F. ) ;
#24930=CARTESIAN_POINT ( 'NONE',  ( 18.46858270002952551, -9.474202674710566541, -7.102021934703857120 ) ) ;
#24942=DIRECTION ( 'NONE',  ( -1.000000000000000000, -0.000000000000000000, -0.000000000000000000 ) ) ;
#24957=EDGE_CURVE ( 'NONE', #197965, #86957, #196350, .T. ) ;
#24978=ORIENTED_EDGE ( 'NONE', *, *, #69913, .T. ) ;
#24981=DIRECTION ( 'NONE',  ( 0.000000000000000000, 0.000000000000000000, 1.000000000000000000 ) ) ;
#24982=VERTEX_POINT ( 'NONE', #192511 ) ;
#24983=LINE ( 'NONE', #124072, #171963 ) ;
#25062=CYLINDRICAL_SURFACE ( 'NONE', #88249, 0.09999999999999939493 ) ;
#25071=CARTESIAN_POINT ( 'NONE',  ( -20.89878130938411616, 10.32747123226657493, -39.07740328502492844 ) ) ;
#25102=CARTESIAN_POINT ( 'NONE',  ( -23.15000000000000213, -9.000000000000001776, -23.60603087734756045 ) ) ;
#25107=CARTESIAN_POINT ( 'NONE',  ( 21.07928932188134397, 0.09889514565439641580, 6.328516656393307294 ) ) ;
#25131=ORIENTED_EDGE ( 'NONE', *, *, #200286, .F. ) ;
#25134=ORIENTED_EDGE ( 'NONE', *, *, #156333, .T. ) ;
#25163=DIRECTION ( 'NONE',  ( 1.000000000000000000, 2.952720810173289112E-16, -0.000000000000000000 ) ) ;
#25182=VECTOR ( 'NONE', #211439, 1000.000000000000000 ) ;
#25183=EDGE_CURVE ( 'NONE', #152840, #37872, #188911, .T. ) ;
#25189=EDGE_CURVE ( 'NONE', #109469, #84065, #222304, .T. ) ;
#25232=ORIENTED_EDGE ( 'NONE', *, *, #81431, .T. ) ;
#25254=CARTESIAN_POINT ( 'NONE',  ( -20.94560253601877164, 11.74999999999999645, -26.51008351251536865 ) ) ;
#25272=CARTESIAN_POINT ( 'NONE',  ( -21.05000000000000071, 0.000000000000000000, -29.50000000000000355 ) ) ;
#25282=VECTOR ( 'NONE', #219946, 1000.000000000000000 ) ;
#25314=EDGE_CURVE ( 'NONE', #162626, #112086, #171399, .T. ) ;
#25319=DIRECTION ( 'NONE',  ( 0.000000000000000000, -0.1350103645451904977, -0.9908441862701596881 ) ) ;
#25328=ORIENTED_EDGE ( 'NONE', *, *, #91523, .F. ) ;
#25345=DIRECTION ( 'NONE',  ( -1.000000000000000000, -0.000000000000000000, 0.000000000000000000 ) ) ;
#25393=CARTESIAN_POINT ( 'NONE',  ( 18.52643265882457868, 10.31973158070287333, -39.05053347133544861 ) ) ;
#25395=DIRECTION ( 'NONE',  ( 0.000000000000000000, 1.000000000000000000, -6.308085367188393199E-16 ) ) ;
#25425=ORIENTED_EDGE ( 'NONE', *, *, #98448, .F. ) ;
#25433=EDGE_CURVE ( 'NONE', #10751, #49099, #180723, .T. ) ;
#25438=ORIENTED_EDGE ( 'NONE', *, *, #48135, .T. ) ;
#25447=CYLINDRICAL_SURFACE ( 'NONE', #111465, 0.09999999999999939493 ) ;
#25452=AXIS2_PLACEMENT_3D ( 'NONE', #35598, #133389, #212920 ) ;
#25466=EDGE_CURVE ( 'NONE', #43854, #226150, #209961, .T. ) ;
#25487=TOROIDAL_SURFACE ( 'NONE', #42240, 12.97499999999999609, 0.1000000000000000056 ) ;
#25489=DIRECTION ( 'NONE',  ( 3.469446951953635015E-14, -0.000000000000000000, 1.000000000000000000 ) ) ;
#25502=AXIS2_PLACEMENT_3D ( 'NONE', #103662, #85371, #124550 ) ;
#25519=EDGE_CURVE ( 'NONE', #208882, #202160, #184999, .T. ) ;
#25528=EDGE_LOOP ( 'NONE', ( #169349, #243508, #248005, #10608 ) ) ;
#25580=ORIENTED_EDGE ( 'NONE', *, *, #69326, .T. ) ;
#25635=EDGE_CURVE ( 'NONE', #3044, #188675, #97169, .T. ) ;
#25648=CIRCLE ( 'NONE', #34068, 0.09999999999999939493 ) ;
#25649=CARTESIAN_POINT ( 'NONE',  ( -18.49719636458550553, -9.446365359228076741, -7.071613869883250914 ) ) ;
#25656=AXIS2_PLACEMENT_3D ( 'NONE', #960, #75437, #137925 ) ;
#25716=DIRECTION ( 'NONE',  ( 1.000000000000000000, 0.000000000000000000, 0.000000000000000000 ) ) ;
#25742=CIRCLE ( 'NONE', #75811, 2.000000000000001776 ) ;
#25752=LINE ( 'NONE', #63586, #231645 ) ;
#25762=EDGE_CURVE ( 'NONE', #213598, #126780, #227317, .T. ) ;
#25765=FACE_OUTER_BOUND ( 'NONE', #59118, .T. ) ;
#25769=CONICAL_SURFACE ( 'NONE', #167273, 4.299999999999956302, 0.7853981633974466137 ) ;
#25790=CARTESIAN_POINT ( 'NONE',  ( 18.59999999999999432, 1.162701749938009677, -8.099999999999999645 ) ) ;
#25799=EDGE_CURVE ( 'NONE', #211613, #86491, #172005, .T. ) ;
#25808=AXIS2_PLACEMENT_3D ( 'NONE', #56004, #234675, #215110 ) ;
#25811=EDGE_CURVE ( 'NONE', #45832, #256245, #47043, .T. ) ;
#25832=EDGE_CURVE ( 'NONE', #202242, #204776, #84612, .T. ) ;
#25836=EDGE_LOOP ( 'NONE', ( #242179, #1367, #135468, #151353 ) ) ;
#25913=DIRECTION ( 'NONE',  ( 1.000000000000000000, -0.000000000000000000, -0.000000000000000000 ) ) ;
#25914=CARTESIAN_POINT ( 'NONE',  ( 18.49999999999999289, 10.49142135623730709, -24.85000000000000142 ) ) ;
#25980=FACE_OUTER_BOUND ( 'NONE', #6990, .T. ) ;
#25983=CARTESIAN_POINT ( 'NONE',  ( -20.94999999999999929, 1.736257131597397585, -11.56865232901749962 ) ) ;
#25988=ORIENTED_EDGE ( 'NONE', *, *, #66503, .T. ) ;
#26011=AXIS2_PLACEMENT_3D ( 'NONE', #97627, #177225, #52092 ) ;
#26023=AXIS2_PLACEMENT_3D ( 'NONE', #217788, #39204, #200823 ) ;
#26068=FACE_OUTER_BOUND ( 'NONE', #39914, .T. ) ;
#26074=CARTESIAN_POINT ( 'NONE',  ( -22.49544290803771318, 11.74987023785715934, 0.06531195925749262721 ) ) ;
#26105=CARTESIAN_POINT ( 'NONE',  ( -22.24259225415828567, 7.491937870565431368, 0.09906588345283832975 ) ) ;
#26117=CARTESIAN_POINT ( 'NONE',  ( 20.94999999999999929, 4.999999999999997335, -21.59473398108690390 ) ) ;
#26199=CIRCLE ( 'NONE', #151085, 0.5000000000000004441 ) ;
#26201=VECTOR ( 'NONE', #48231, 1000.000000000000000 ) ;
#26212=CARTESIAN_POINT ( 'NONE',  ( -23.25000000000000000, -1.249999999999999334, -41.30048075441507649 ) ) ;
#26218=VERTEX_POINT ( 'NONE', #236972 ) ;
#26248=DIRECTION ( 'NONE',  ( -0.000000000000000000, 1.000000000000000000, 2.891205793294679805E-16 ) ) ;
#26289=DIRECTION ( 'NONE',  ( -4.408576920032448588E-17, 0.1350103645451876944, -0.9908441862701601321 ) ) ;
#26342=DIRECTION ( 'NONE',  ( 0.000000000000000000, 1.000000000000000000, -0.000000000000000000 ) ) ;
#26348=CARTESIAN_POINT ( 'NONE',  ( -20.94999999999999929, 5.850000000000004086, -23.36750277572207324 ) ) ;
#26366=DIRECTION ( 'NONE',  ( 0.000000000000000000, 0.000000000000000000, -1.000000000000000000 ) ) ;
#26370=ORIENTED_EDGE ( 'NONE', *, *, #61506, .F. ) ;
#26386=CARTESIAN_POINT ( 'NONE',  ( 21.05000000000000071, 4.813084112149527805, -21.55848224347618114 ) ) ;
#26392=EDGE_CURVE ( 'NONE', #185736, #191967, #26407, .T. ) ;
#26396=ORIENTED_EDGE ( 'NONE', *, *, #101500, .T. ) ;
#26407=CIRCLE ( 'NONE', #172202, 12.97499999999999609 ) ;
#26414=ORIENTED_EDGE ( 'NONE', *, *, #219105, .T. ) ;
#26423=EDGE_CURVE ( 'NONE', #102134, #88943, #255077, .T. ) ;
#26428=AXIS2_PLACEMENT_3D ( 'NONE', #178156, #234239, #198974 ) ;
#26439=CYLINDRICAL_SURFACE ( 'NONE', #40505, 0.1000000000000001443 ) ;
#26477=DIRECTION ( 'NONE',  ( 1.000000000000000000, 0.000000000000000000, 0.000000000000000000 ) ) ;
#26486=AXIS2_PLACEMENT_3D ( 'NONE', #232443, #151627, #113744 ) ;
#26515=AXIS2_PLACEMENT_3D ( 'NONE', #63914, #243825, #205991 ) ;
#26533=VERTEX_POINT ( 'NONE', #248517 ) ;
#26535=CARTESIAN_POINT ( 'NONE',  ( -20.99780126800938262, 11.60538868787665301, -26.58735257170532762 ) ) ;
#26537=VERTEX_POINT ( 'NONE', #129842 ) ;
#26551=CARTESIAN_POINT ( 'NONE',  ( -20.54999999999999361, 11.64999999999999680, -21.35000000000000142 ) ) ;
#26558=FACE_OUTER_BOUND ( 'NONE', #166427, .T. ) ;
#26585=VECTOR ( 'NONE', #130005, 1000.000000000000000 ) ;
#26608=CYLINDRICAL_SURFACE ( 'NONE', #13732, 0.09999999999999939493 ) ;
#26648=CARTESIAN_POINT ( 'NONE',  ( 23.25000000000000000, -9.000000000000000000, -23.60603087734755690 ) ) ;
#26666=ORIENTED_EDGE ( 'NONE', *, *, #113984, .T. ) ;
#26678=ORIENTED_EDGE ( 'NONE', *, *, #2894, .T. ) ;
#26697=ORIENTED_EDGE ( 'NONE', *, *, #63806, .T. ) ;
#26700=ORIENTED_EDGE ( 'NONE', *, *, #256157, .F. ) ;
#26725=CIRCLE ( 'NONE', #230729, 0.09999999999999939493 ) ;
#26740=DIRECTION ( 'NONE',  ( -0.000000000000000000, 0.8660254037844502539, 0.4999999999999799605 ) ) ;
#26782=ORIENTED_EDGE ( 'NONE', *, *, #135045, .F. ) ;
#26794=DIRECTION ( 'NONE',  ( -1.000000000000000000, 0.000000000000000000, 0.000000000000000000 ) ) ;
#26807=ORIENTED_EDGE ( 'NONE', *, *, #10707, .F. ) ;
#26831=CARTESIAN_POINT ( 'NONE',  ( 21.05000000000000071, 4.898587196589410857E-16, -29.50000000000000355 ) ) ;
#26853=FACE_OUTER_BOUND ( 'NONE', #52820, .T. ) ;
#26857=DIRECTION ( 'NONE',  ( 0.000000000000000000, 0.000000000000000000, -1.000000000000000000 ) ) ;
#26866=DIRECTION ( 'NONE',  ( 7.304098846218134667E-16, -1.000000000000000000, 0.000000000000000000 ) ) ;
#26869=AXIS2_PLACEMENT_3D ( 'NONE', #135936, #36894, #116404 ) ;
#26901=ORIENTED_EDGE ( 'NONE', *, *, #8801, .F. ) ;
#26918=LINE ( 'NONE', #141688, #34008 ) ;
#26951=VERTEX_POINT ( 'NONE', #237647 ) ;
#26958=CARTESIAN_POINT ( 'NONE',  ( -21.14999999999999858, -0.09999999999999939493, 11.64957080754479968 ) ) ;
#26978=ORIENTED_EDGE ( 'NONE', *, *, #111463, .T. ) ;
#26991=CARTESIAN_POINT ( 'NONE',  ( -23.15000000000000213, -11.75000000000000000, 11.75000000000000000 ) ) ;
#26995=FACE_OUTER_BOUND ( 'NONE', #145307, .T. ) ;
#26996=DIRECTION ( 'NONE',  ( 1.000000000000000000, 0.000000000000000000, 0.000000000000000000 ) ) ;
#27021=ORIENTED_EDGE ( 'NONE', *, *, #237852, .F. ) ;
#27030=CARTESIAN_POINT ( 'NONE',  ( 20.85000000000000142, 11.75000000000000355, -33.50000000000000000 ) ) ;
#27080=FACE_OUTER_BOUND ( 'NONE', #14447, .T. ) ;
#27085=ADVANCED_FACE ( 'NONE', ( #35625 ), #194698, .F. ) ;
#27086=CARTESIAN_POINT ( 'NONE',  ( 21.05000000000000071, 0.000000000000000000, -0.09999999999999592548 ) ) ;
#27105=DIRECTION ( 'NONE',  ( 0.000000000000000000, -0.8777080977375132376, 0.4791956752371582251 ) ) ;
#27118=ORIENTED_EDGE ( 'NONE', *, *, #44275, .T. ) ;
#27145=DIRECTION ( 'NONE',  ( 1.000000000000000000, -0.000000000000000000, -0.000000000000000000 ) ) ;
#27149=ORIENTED_EDGE ( 'NONE', *, *, #140754, .F. ) ;
#27157=EDGE_CURVE ( 'NONE', #122573, #62691, #124127, .T. ) ;
#27159=LINE ( 'NONE', #204463, #245358 ) ;
#27162=CIRCLE ( 'NONE', #110505, 0.1000000000000000472 ) ;
#27178=ORIENTED_EDGE ( 'NONE', *, *, #78623, .T. ) ;
#27186=DIRECTION ( 'NONE',  ( 1.000000000000000000, 0.000000000000000000, 0.000000000000000000 ) ) ;
#27196=ORIENTED_EDGE ( 'NONE', *, *, #189097, .F. ) ;
#27204=VECTOR ( 'NONE', #239845, 1000.000000000000000 ) ;
#27253=DIRECTION ( 'NONE',  ( -1.000000000000000000, -0.000000000000000000, -0.000000000000000000 ) ) ;
#27263=CARTESIAN_POINT ( 'NONE',  ( -18.59999999999999787, -9.480686695278977894, -40.44111516875783963 ) ) ;
#27269=EDGE_LOOP ( 'NONE', ( #22267, #77698, #14267 ) ) ;
#27304=CARTESIAN_POINT ( 'NONE',  ( -18.59999999999999787, 9.150000000000002132, -12.34999999999999964 ) ) ;
#27314=ADVANCED_FACE ( 'NONE', ( #108407 ), #211358, .T. ) ;
#27321=CARTESIAN_POINT ( 'NONE',  ( -20.12071067811865888, 9.320710678118654613, -12.34999999999999964 ) ) ;
#27360=ADVANCED_FACE ( 'NONE', ( #10591 ), #214377, .F. ) ;
#27361=CARTESIAN_POINT ( 'NONE',  ( 20.01093837587850288, 11.75000000000000711, -24.75439743459708808 ) ) ;
#27381=FACE_OUTER_BOUND ( 'NONE', #33335, .T. ) ;
#27394=VECTOR ( 'NONE', #179131, 1000.000000000000000 ) ;
#27450=EDGE_LOOP ( 'NONE', ( #228195, #148069, #222139, #10069 ) ) ;
#27464=CARTESIAN_POINT ( 'NONE',  ( 23.15000000000000213, -11.64999999999999147, -30.39999999999999858 ) ) ;
#27469=ADVANCED_FACE ( 'NONE', ( #14459 ), #127318, .T. ) ;
#27486=DIRECTION ( 'NONE',  ( 0.000000000000000000, 0.9999631594459055250, 0.008583690987127922528 ) ) ;
#27518=CARTESIAN_POINT ( 'NONE',  ( -18.50000000000000000, -1.162701749938009677, -8.099999999999999645 ) ) ;
#27529=CARTESIAN_POINT ( 'NONE',  ( -21.05000000000000071, 6.299230910092280311, 0.09843750000031994962 ) ) ;
#27578=EDGE_CURVE ( 'NONE', #63488, #92976, #68637, .T. ) ;
#27580=ADVANCED_FACE ( 'NONE', ( #148159 ), #128607, .T. ) ;
#27594=CARTESIAN_POINT ( 'NONE',  ( -21.14999999999999858, -0.09999999999999939493, 6.249999999999998224 ) ) ;
#27603=CARTESIAN_POINT ( 'NONE',  ( 18.49999999999998934, 6.450000000000001066, -10.01702717044001822 ) ) ;
#27621=VECTOR ( 'NONE', #173281, 1000.000000000000000 ) ;
#27637=EDGE_CURVE ( 'NONE', #139796, #161077, #172916, .T. ) ;
#27666=CARTESIAN_POINT ( 'NONE',  ( -18.59999999999999787, -1.851617760468904805, -45.10318971960366241 ) ) ;
#27677=ORIENTED_EDGE ( 'NONE', *, *, #73671, .F. ) ;
#27693=CIRCLE ( 'NONE', #81766, 0.1000000000000012546 ) ;
#27697=CARTESIAN_POINT ( 'NONE',  ( -23.25000000000000000, 1.999999999999998224, -20.27537807723789953 ) ) ;
#27702=AXIS2_PLACEMENT_3D ( 'NONE', #223661, #26794, #65890 ) ;
#27718=ORIENTED_EDGE ( 'NONE', *, *, #88445, .T. ) ;
#27728=VERTEX_POINT ( 'NONE', #60605 ) ;
#27747=PLANE ( 'NONE',  #144684 ) ;
#27749=ORIENTED_EDGE ( 'NONE', *, *, #120353, .F. ) ;
#27765=VECTOR ( 'NONE', #3829, 999.9999999999998863 ) ;
#27796=ORIENTED_EDGE ( 'NONE', *, *, #14360, .T. ) ;
#27843=ORIENTED_EDGE ( 'NONE', *, *, #61571, .T. ) ;
#27868=EDGE_CURVE ( 'NONE', #156671, #241011, #27162, .T. ) ;
#27884=DIRECTION ( 'NONE',  ( 0.000000000000000000, 0.000000000000000000, -1.000000000000000000 ) ) ;
#27900=DIRECTION ( 'NONE',  ( 1.000000000000000000, 0.000000000000000000, 0.000000000000000000 ) ) ;
#27935=ORIENTED_EDGE ( 'NONE', *, *, #41117, .F. ) ;
#27943=DIRECTION ( 'NONE',  ( 0.000000000000000000, 1.000000000000000000, 0.000000000000000000 ) ) ;
#27946=DIRECTION ( 'NONE',  ( 0.000000000000000000, 0.000000000000000000, 1.000000000000000000 ) ) ;
#27955=AXIS2_PLACEMENT_3D ( 'NONE', #63987, #237491, #217897 ) ;
#27958=ADVANCED_FACE ( 'NONE', ( #150455 ), #243973, .F. ) ;
#27965=CARTESIAN_POINT ( 'NONE',  ( -21.14999999999999858, -11.75000000000000000, 3.469446951953614189E-15 ) ) ;
#27979=CARTESIAN_POINT ( 'NONE',  ( 18.55807992284871588, 10.32898536000685930, -39.08266832227643306 ) ) ;
#27982=ORIENTED_EDGE ( 'NONE', *, *, #187071, .T. ) ;
#28012=ORIENTED_EDGE ( 'NONE', *, *, #95875, .F. ) ;
#28020=VECTOR ( 'NONE', #109241, 1000.000000000000000 ) ;
#28023=CARTESIAN_POINT ( 'NONE',  ( 18.59999999999999076, 11.65000000000000391, -24.75000000000000000 ) ) ;
#28028=VERTEX_POINT ( 'NONE', #13503 ) ;
#28031=EDGE_LOOP ( 'NONE', ( #76784, #193384, #229541, #174619 ) ) ;
#28036=VECTOR ( 'NONE', #186522, 1000.000000000000000 ) ;
#28065=AXIS2_PLACEMENT_3D ( 'NONE', #139430, #136883, #80742 ) ;
#28072=DIRECTION ( 'NONE',  ( -3.265361837132813093E-16, 1.000000000000000000, 0.000000000000000000 ) ) ;
#28098=SPHERICAL_SURFACE ( 'NONE', #149748, 0.1000000000000000056 ) ;
#28127=ORIENTED_EDGE ( 'NONE', *, *, #71457, .T. ) ;
#28134=ORIENTED_EDGE ( 'NONE', *, *, #214888, .T. ) ;
#28165=AXIS2_PLACEMENT_3D ( 'NONE', #71621, #246393, #169464 ) ;
#28166=DIRECTION ( 'NONE',  ( 0.000000000000000000, 0.000000000000000000, -1.000000000000000000 ) ) ;
#28198=CARTESIAN_POINT ( 'NONE',  ( 20.87600722750343252, 10.33112638555853913, -39.09012289269746532 ) ) ;
#28201=VERTEX_POINT ( 'NONE', #182862 ) ;
#28206=EDGE_CURVE ( 'NONE', #174560, #231683, #111470, .T. ) ;
#28208=CARTESIAN_POINT ( 'NONE',  ( 21.09787244211743840, 8.775370707337266651, -12.23925338431755883 ) ) ;
#28209=DIRECTION ( 'NONE',  ( 0.7071067811865474617, 0.7071067811865474617, 2.044391222244499837E-16 ) ) ;
#28224=DIRECTION ( 'NONE',  ( 0.000000000000000000, 0.000000000000000000, -1.000000000000000000 ) ) ;
#28228=CARTESIAN_POINT ( 'NONE',  ( 22.14074124539698829, 7.390077851043746371, 0.09905289584407064862 ) ) ;
#28245=CARTESIAN_POINT ( 'NONE',  ( -18.49999999999997868, -9.321008403361298988, -7.235938249077866757 ) ) ;
#28249=CARTESIAN_POINT ( 'NONE',  ( -23.15000000000000213, 0.000000000000000000, -33.50000000000000000 ) ) ;
#28283=EDGE_CURVE ( 'NONE', #255303, #113692, #181457, .T. ) ;
#28297=DIRECTION ( 'NONE',  ( 1.000000000000000000, -0.000000000000000000, -0.000000000000000000 ) ) ;
#28307=EDGE_CURVE ( 'NONE', #158135, #124226, #116148, .T. ) ;
#28331=DIRECTION ( 'NONE',  ( 0.000000000000000000, 0.000000000000000000, 1.000000000000000000 ) ) ;
#28338=ORIENTED_EDGE ( 'NONE', *, *, #39739, .T. ) ;
#28362=CARTESIAN_POINT ( 'NONE',  ( -21.95218792049438861, 0.09902843979991576839, 7.201507561246681455 ) ) ;
#28393=ORIENTED_EDGE ( 'NONE', *, *, #147841, .F. ) ;
#28421=FACE_OUTER_BOUND ( 'NONE', #16522, .T. ) ;
#28425=VERTEX_POINT ( 'NONE', #211389 ) ;
#28427=CARTESIAN_POINT ( 'NONE',  ( -20.94999999999999929, -1.851028230140860487, -11.65391326942249250 ) ) ;
#28440=DIRECTION ( 'NONE',  ( 0.000000000000000000, -0.6728971962616783209, -0.7397360091702797069 ) ) ;
#28476=DIRECTION ( 'NONE',  ( 1.000000000000000000, -0.000000000000000000, -0.000000000000000000 ) ) ;
#28483=CARTESIAN_POINT ( 'NONE',  ( 21.05281448260627641, 8.776010158537628669, -12.17355791181142344 ) ) ;
#28499=CIRCLE ( 'NONE', #228372, 12.87499999999999822 ) ;
#28523=CIRCLE ( 'NONE', #240858, 0.09999999999999939493 ) ;
#28546=AXIS2_PLACEMENT_3D ( 'NONE', #182691, #166, #80983 ) ;
#28561=DIRECTION ( 'NONE',  ( -1.000000000000000000, 0.000000000000000000, 0.000000000000000000 ) ) ;
#28600=ORIENTED_EDGE ( 'NONE', *, *, #3999, .T. ) ;
#28610=EDGE_CURVE ( 'NONE', #29243, #170516, #44257, .T. ) ;
#28653=TOROIDAL_SURFACE ( 'NONE', #182742, 0.2000000000000000111, 0.1000000000000000056 ) ;
#28654=CARTESIAN_POINT ( 'NONE',  ( 19.75857864376269646, 11.65000000000000924, -24.75000000000000000 ) ) ;
#28679=CARTESIAN_POINT ( 'NONE',  ( -22.48660254037843487, 11.74999999999999822, 0.04999999999998229472 ) ) ;
#28713=ORIENTED_EDGE ( 'NONE', *, *, #193558, .T. ) ;
#28720=CIRCLE ( 'NONE', #174477, 0.2000000000000005107 ) ;
#28724=ORIENTED_EDGE ( 'NONE', *, *, #30569, .T. ) ;
#28741=DIRECTION ( 'NONE',  ( -1.000000000000000000, 0.000000000000000000, 0.000000000000000000 ) ) ;
#28773=LINE ( 'NONE', #106960, #28036 ) ;
#28801=EDGE_LOOP ( 'NONE', ( #68185, #4849, #115317, #90305 ) ) ;
#28864=CARTESIAN_POINT ( 'NONE',  ( -22.57320508075687115, 11.65000000000000036, -3.122502256758252770E-14 ) ) ;
#28874=ORIENTED_EDGE ( 'NONE', *, *, #6892, .F. ) ;
#28879=FACE_BOUND ( 'NONE', #230763, .T. ) ;
#28917=VECTOR ( 'NONE', #244871, 1000.000000000000227 ) ;
#28945=ADVANCED_FACE ( 'NONE', ( #104878 ), #204016, .T. ) ;
#28949=CARTESIAN_POINT ( 'NONE',  ( -20.85000000000000142, 0.000000000000000000, -41.40000000000000568 ) ) ;
#28961=ADVANCED_FACE ( 'NONE', ( #153085 ), #73534, .T. ) ;
#28977=ORIENTED_EDGE ( 'NONE', *, *, #49074, .F. ) ;
#28984=ORIENTED_EDGE ( 'NONE', *, *, #59562, .F. ) ;
#29061=VERTEX_POINT ( 'NONE', #188306 ) ;
#29062=DIRECTION ( 'NONE',  ( 0.000000000000000000, 0.8660254037844411501, 0.4999999999999956701 ) ) ;
#29067=AXIS2_PLACEMENT_3D ( 'NONE', #217655, #2468, #84538 ) ;
#29070=DIRECTION ( 'NONE',  ( 0.000000000000000000, 2.891205793294679805E-16, -1.000000000000000000 ) ) ;
#29089=EDGE_LOOP ( 'NONE', ( #133919, #132583, #96643, #11594, #54564 ) ) ;
#29137=EDGE_CURVE ( 'NONE', #235074, #162495, #223647, .T. ) ;
#29144=ADVANCED_FACE ( 'NONE', ( #257221 ), #175223, .T. ) ;
#29160=ORIENTED_EDGE ( 'NONE', *, *, #208296, .F. ) ;
#29167=AXIS2_PLACEMENT_3D ( 'NONE', #240282, #57761, #116475 ) ;
#29204=CARTESIAN_POINT ( 'NONE',  ( -23.25000000000000000, 5.082284216461512198E-16, 4.149999999999999467 ) ) ;
#29221=ORIENTED_EDGE ( 'NONE', *, *, #187309, .T. ) ;
#29222=FACE_OUTER_BOUND ( 'NONE', #187232, .T. ) ;
#29237=DIRECTION ( 'NONE',  ( 0.000000000000000000, -1.000000000000000000, 0.000000000000000000 ) ) ;
#29243=VERTEX_POINT ( 'NONE', #220716 ) ;
#29247=DIRECTION ( 'NONE',  ( 0.000000000000000000, 0.000000000000000000, -1.000000000000000000 ) ) ;
#29253=LINE ( 'NONE', #110023, #131230 ) ;
#29263=EDGE_CURVE ( 'NONE', #91559, #15975, #248610, .T. ) ;
#29265=ORIENTED_EDGE ( 'NONE', *, *, #208296, .T. ) ;
#29268=VECTOR ( 'NONE', #174856, 1000.000000000000000 ) ;
#29283=FACE_OUTER_BOUND ( 'NONE', #57984, .T. ) ;
#29317=FACE_BOUND ( 'NONE', #148798, .T. ) ;
#29329=EDGE_CURVE ( 'NONE', #113369, #159975, #168496, .T. ) ;
#29357=CARTESIAN_POINT ( 'NONE',  ( 23.15000000000000213, -9.500000000000000000, -23.60603087734755690 ) ) ;
#29388=CARTESIAN_POINT ( 'NONE',  ( 20.94999999999999929, 0.000000000000000000, -33.50000000000000000 ) ) ;
#29399=CARTESIAN_POINT ( 'NONE',  ( -21.05000000000000071, 1.261786168565025568, -8.086498963545480478 ) ) ;
#29418=CARTESIAN_POINT ( 'NONE',  ( 18.59999999999996945, 7.021664781900089913, -37.33356540189728889 ) ) ;
#29425=CARTESIAN_POINT ( 'NONE',  ( 18.39999999999999858, -9.682403433476396870, -40.15684337741279109 ) ) ;
#29445=CIRCLE ( 'NONE', #191939, 0.1000000000000028644 ) ;
#29452=CYLINDRICAL_SURFACE ( 'NONE', #20264, 0.09999999999999939493 ) ;
#29458=DIRECTION ( 'NONE',  ( 0.000000000000000000, 0.000000000000000000, -1.000000000000000000 ) ) ;
#29460=ORIENTED_EDGE ( 'NONE', *, *, #109787, .F. ) ;
#29471=CARTESIAN_POINT ( 'NONE',  ( 21.14999999999999858, 11.65000000000000746, -12.15000000000000036 ) ) ;
#29477=CARTESIAN_POINT ( 'NONE',  ( 21.14999999999999858, 0.000000000000000000, 6.540656951701244282 ) ) ;
#29485=ORIENTED_EDGE ( 'NONE', *, *, #35409, .F. ) ;
#29523=CARTESIAN_POINT ( 'NONE',  ( 21.05000000000000071, 10.60832956795391802, -7.591685013295530027 ) ) ;
#29527=CARTESIAN_POINT ( 'NONE',  ( -18.58693740092133240, -9.406432150253023039, -7.124816456501293693 ) ) ;
#29536=CARTESIAN_POINT ( 'NONE',  ( -21.05000000000000071, -1.162701749938009677, -8.099999999999999645 ) ) ;
#29565=UNCERTAINTY_MEASURE_WITH_UNIT (LENGTH_MEASURE( 1.000000000000000082E-05 ), #3045, 'distance_accuracy_value', 'NONE');
#29570=CIRCLE ( 'NONE', #100250, 4.099999999999999645 ) ;
#29576=DIRECTION ( 'NONE',  ( 1.000000000000000000, 0.000000000000000000, 0.000000000000000000 ) ) ;
#29639=VERTEX_POINT ( 'NONE', #176173 ) ;
#29643=DIRECTION ( 'NONE',  ( -0.000000000000000000, -2.891205793294679805E-16, 1.000000000000000000 ) ) ;
#29644=CARTESIAN_POINT ( 'NONE',  ( 23.15000000000000213, -9.000000000000000000, -24.10603087734755690 ) ) ;
#29671=EDGE_CURVE ( 'NONE', #241513, #160000, #180820, .T. ) ;
#29683=CARTESIAN_POINT ( 'NONE',  ( -21.05000000000000071, 1.835341550224411922, -11.55515129256298046 ) ) ;
#29684=ORIENTED_EDGE ( 'NONE', *, *, #5136, .T. ) ;
#29701=EDGE_CURVE ( 'NONE', #52139, #20565, #191344, .T. ) ;
#29711=ORIENTED_EDGE ( 'NONE', *, *, #26392, .T. ) ;
#29714=EDGE_CURVE ( 'NONE', #241513, #50852, #239077, .T. ) ;
#29716=ORIENTED_EDGE ( 'NONE', *, *, #197497, .T. ) ;
#29754=CARTESIAN_POINT ( 'NONE',  ( 20.94999999999999929, -11.64999999999999147, -30.59999999999999432 ) ) ;
#29756=CIRCLE ( 'NONE', #242092, 7.800000000000000711 ) ;
#29774=AXIS2_PLACEMENT_3D ( 'NONE', #73705, #254821, #54103 ) ;
#29792=LINE ( 'NONE', #191428, #62592 ) ;
#29801=CARTESIAN_POINT ( 'NONE',  ( 20.95512840106819752, 10.62384869377332031, -12.20247922079885328 ) ) ;
#29832=CARTESIAN_POINT ( 'NONE',  ( -20.64999999999999858, -9.400000000000002132, -23.60603087734756045 ) ) ;
#29843=DIRECTION ( 'NONE',  ( -4.448008912761043807E-16, 1.000000000000000000, -8.896017825522087613E-16 ) ) ;
#29858=ADVANCED_FACE ( 'NONE', ( #6486 ), #228125, .F. ) ;
#29878=EDGE_CURVE ( 'NONE', #49525, #115218, #115868, .T. ) ;
#29909=CARTESIAN_POINT ( 'NONE',  ( 19.81427058490548276, 11.66856398038106768, -24.75000000000000000 ) ) ;
#29929=DIRECTION ( 'NONE',  ( 0.000000000000000000, 1.000000000000000000, 0.000000000000000000 ) ) ;
#29940=AXIS2_PLACEMENT_3D ( 'NONE', #246525, #67897, #125312 ) ;
#29942=EDGE_CURVE ( 'NONE', #165206, #123641, #68572, .T. ) ;
#29981=FACE_OUTER_BOUND ( 'NONE', #81194, .T. ) ;
#30020=ORIENTED_EDGE ( 'NONE', *, *, #45576, .T. ) ;
#30046=CARTESIAN_POINT ( 'NONE',  ( -21.64999999999999858, 7.349999999999998757, -21.25000000000000000 ) ) ;
#30049=ORIENTED_EDGE ( 'NONE', *, *, #245581, .F. ) ;
#30078=CARTESIAN_POINT ( 'NONE',  ( 21.05000000000000071, 6.540656951701244282, -0.09999999999999939493 ) ) ;
#30092=CARTESIAN_POINT ( 'NONE',  ( -18.42554971533677843, -9.497159669437746032, -7.039826913548645315 ) ) ;
#30137=CARTESIAN_POINT ( 'NONE',  ( 20.12500000000000000, 9.749999999999998224, -21.25000000000000000 ) ) ;
#30140=AXIS2_PLACEMENT_3D ( 'NONE', #108266, #88664, #168279 ) ;
#30201=DIRECTION ( 'NONE',  ( 0.000000000000000000, 0.000000000000000000, -1.000000000000000000 ) ) ;
#30268=EDGE_CURVE ( 'NONE', #56467, #177411, #111702, .T. ) ;
#30289=DIRECTION ( 'NONE',  ( 0.000000000000000000, 0.1350103645451876666, 0.9908441862701600211 ) ) ;
#30349=CARTESIAN_POINT ( 'NONE',  ( 18.49999999999999645, -1.135018845910178431, -41.21697688343231647 ) ) ;
#30369=DIRECTION ( 'NONE',  ( 1.000000000000000000, 0.000000000000000000, 0.000000000000000000 ) ) ;
#30393=ORIENTED_EDGE ( 'NONE', *, *, #226142, .F. ) ;
#30394=EDGE_CURVE ( 'NONE', #106265, #161501, #89575, .T. ) ;
#30402=DIRECTION ( 'NONE',  ( 1.000000000000000000, -7.304098846218133681E-16, 0.000000000000000000 ) ) ;
#30423=CARTESIAN_POINT ( 'NONE',  ( 23.15000000000000213, -11.74999999999999112, -30.39999999999999858 ) ) ;
#30431=CIRCLE ( 'NONE', #242799, 0.09999999999999939493 ) ;
#30445=DIRECTION ( 'NONE',  ( 0.000000000000000000, 0.000000000000000000, -1.000000000000000000 ) ) ;
#30489=EDGE_LOOP ( 'NONE', ( #150807, #154247, #252827, #21798 ) ) ;
#30507=DIRECTION ( 'NONE',  ( 1.734723475976817507E-14, 0.000000000000000000, -1.000000000000000000 ) ) ;
#30520=LINE ( 'NONE', #110028, #37793 ) ;
#30569=EDGE_CURVE ( 'NONE', #102134, #32374, #74565, .T. ) ;
#30584=CARTESIAN_POINT ( 'NONE',  ( -20.94999999999999929, 5.021051876504146399E-16, -37.60000000000000142 ) ) ;
#30588=EDGE_LOOP ( 'NONE', ( #82019, #168822, #124367, #46540, #144795 ) ) ;
#30598=DIRECTION ( 'NONE',  ( 0.000000000000000000, 0.000000000000000000, 1.000000000000000000 ) ) ;
#30601=AXIS2_PLACEMENT_3D ( 'NONE', #122975, #21324, #39613 ) ;
#30602=DIRECTION ( 'NONE',  ( 0.000000000000000000, -0.8660254037844384856, 0.5000000000000002220 ) ) ;
#30641=CARTESIAN_POINT ( 'NONE',  ( -21.14999999999999858, -0.09999999999999939493, 6.540656951701240729 ) ) ;
#30663=CARTESIAN_POINT ( 'NONE',  ( -23.15000000000000213, 1.910280373831774847, -20.86863214480106166 ) ) ;
#30687=CARTESIAN_POINT ( 'NONE',  ( -18.59999999999999787, 9.350000000000001421, -21.35000000000000142 ) ) ;
#30720=LINE ( 'NONE', #35842, #228452 ) ;
#30790=LINE ( 'NONE', #110293, #188106 ) ;
#30824=EDGE_CURVE ( 'NONE', #141418, #77408, #185457, .T. ) ;
#30826=ORIENTED_EDGE ( 'NONE', *, *, #227717, .F. ) ;
#30835=CIRCLE ( 'NONE', #176578, 0.09999999999999997780 ) ;
#30838=CARTESIAN_POINT ( 'NONE',  ( 23.24999999999999645, 0.000000000000000000, -33.50000000000000000 ) ) ;
#30886=TOROIDAL_SURFACE ( 'NONE', #160058, 0.2000000000000000111, 0.1000000000000000056 ) ;
#30967=ORIENTED_EDGE ( 'NONE', *, *, #191753, .T. ) ;
#30987=ORIENTED_EDGE ( 'NONE', *, *, #139456, .T. ) ;
#30994=EDGE_LOOP ( 'NONE', ( #133895, #71460, #231115, #103685 ) ) ;
#31022=FACE_OUTER_BOUND ( 'NONE', #13964, .T. ) ;
#31044=CARTESIAN_POINT ( 'NONE',  ( 21.06600267594171783, 8.775166069199903163, -12.20426278237474094 ) ) ;
#31051=ORIENTED_EDGE ( 'NONE', *, *, #246762, .T. ) ;
#31066=ORIENTED_EDGE ( 'NONE', *, *, #2804, .F. ) ;
#31069=CIRCLE ( 'NONE', #176787, 11.75000000000000000 ) ;
#31072=VERTEX_POINT ( 'NONE', #63478 ) ;
#31088=EDGE_CURVE ( 'NONE', #32887, #72182, #90948, .T. ) ;
#31127=DIRECTION ( 'NONE',  ( 1.000000000000000000, -0.000000000000000000, -0.000000000000000000 ) ) ;
#31143=CARTESIAN_POINT ( 'NONE',  ( -18.33682934331515568, -9.511185591093616054, -40.40565476867323014 ) ) ;
#31177=DIRECTION ( 'NONE',  ( -1.000000000000000000, 0.000000000000000000, 0.000000000000000000 ) ) ;
#31199=DIRECTION ( 'NONE',  ( 0.000000000000000000, -0.1298341882520124002, -0.9915357197604841577 ) ) ;
#31205=ORIENTED_EDGE ( 'NONE', *, *, #121171, .T. ) ;
#31234=DIRECTION ( 'NONE',  ( 0.000000000000000000, 0.000000000000000000, 1.000000000000000000 ) ) ;
#31245=ORIENTED_EDGE ( 'NONE', *, *, #115905, .F. ) ;
#31261=CARTESIAN_POINT ( 'NONE',  ( -23.15000000000000213, -9.000000000000001776, -24.20603087734755832 ) ) ;
#31311=CARTESIAN_POINT ( 'NONE',  ( -18.50000000000000000, 0.000000000000000000, -33.50000000000000000 ) ) ;
#31318=AXIS2_PLACEMENT_3D ( 'NONE', #114280, #197659, #231681 ) ;
#31326=VERTEX_POINT ( 'NONE', #113523 ) ;
#31328=EDGE_CURVE ( 'NONE', #120640, #84969, #69134, .T. ) ;
#31337=EDGE_CURVE ( 'NONE', #214000, #105911, #52341, .T. ) ;
#31358=AXIS2_PLACEMENT_3D ( 'NONE', #179019, #197257, #56447 ) ;
#31378=CARTESIAN_POINT ( 'NONE',  ( -21.07954640115341860, 6.329287696024277210, 0.06600770713963553804 ) ) ;
#31380=EDGE_LOOP ( 'NONE', ( #80655, #43236, #168530, #247222 ) ) ;
#31401=LINE ( 'NONE', #230870, #114024 ) ;
#31409=ORIENTED_EDGE ( 'NONE', *, *, #168829, .T. ) ;
#31416=ADVANCED_FACE ( 'NONE', ( #198187 ), #219026, .T. ) ;
#31460=CARTESIAN_POINT ( 'NONE',  ( 23.14999999999999503, 11.65000000000000746, -26.48519422934606027 ) ) ;
#31470=CARTESIAN_POINT ( 'NONE',  ( 19.97071067811865674, 11.72071067811866385, -24.70857864376269575 ) ) ;
#31506=ORIENTED_EDGE ( 'NONE', *, *, #160971, .T. ) ;
#31507=EDGE_CURVE ( 'NONE', #256663, #97347, #110642, .T. ) ;
#31512=CARTESIAN_POINT ( 'NONE',  ( -21.05000000000000071, -1.162701749938009677, -8.000000000000000000 ) ) ;
#31534=DIRECTION ( 'NONE',  ( -1.000000000000000000, 0.000000000000000000, 0.000000000000000000 ) ) ;
#31582=CIRCLE ( 'NONE', #64854, 0.09999999999999939493 ) ;
#31598=VERTEX_POINT ( 'NONE', #170673 ) ;
#31620=CIRCLE ( 'NONE', #60792, 7.800000000000001599 ) ;
#31624=DIRECTION ( 'NONE',  ( 1.000000000000000000, 0.000000000000000000, 0.000000000000000000 ) ) ;
#31631=FACE_OUTER_BOUND ( 'NONE', #201524, .T. ) ;
#31644=ORIENTED_EDGE ( 'NONE', *, *, #125080, .F. ) ;
#31668=CARTESIAN_POINT ( 'NONE',  ( -23.15000000000000213, 0.000000000000000000, -33.50000000000000000 ) ) ;
#31673=CARTESIAN_POINT ( 'NONE',  ( -21.05000000000000071, 1.835341550224411922, -11.55515129256298046 ) ) ;
#31682=CARTESIAN_POINT ( 'NONE',  ( -23.25000000000000000, 0.000000000000000000, 0.000000000000000000 ) ) ;
#31707=CIRCLE ( 'NONE', #219104, 0.1000000000000028644 ) ;
#31719=AXIS2_PLACEMENT_3D ( 'NONE', #27464, #41871, #181383 ) ;
#31727=AXIS2_PLACEMENT_3D ( 'NONE', #72326, #129714, #207989 ) ;
#31746=ORIENTED_EDGE ( 'NONE', *, *, #14166, .F. ) ;
#31751=CARTESIAN_POINT ( 'NONE',  ( 20.94999999999999929, -1.835341550224413698, -11.55515129256298046 ) ) ;
#31757=CARTESIAN_POINT ( 'NONE',  ( 22.39999999999999503, 0.09999999999999939493, 6.249999999999998224 ) ) ;
#31765=VERTEX_POINT ( 'NONE', #93018 ) ;
#31770=VERTEX_POINT ( 'NONE', #250803 ) ;
#31781=EDGE_CURVE ( 'NONE', #132561, #144164, #81178, .T. ) ;
#31848=FACE_OUTER_BOUND ( 'NONE', #196067, .T. ) ;
#31858=FACE_OUTER_BOUND ( 'NONE', #248081, .T. ) ;
#31871=EDGE_LOOP ( 'NONE', ( #149010, #149127, #9480, #240412 ) ) ;
#31872=CARTESIAN_POINT ( 'NONE',  ( -23.25000000000000000, 11.75000000000000000, 11.75000000000000000 ) ) ;
#31912=DIRECTION ( 'NONE',  ( 1.000000000000000000, -0.000000000000000000, -0.000000000000000000 ) ) ;
#31920=DIRECTION ( 'NONE',  ( 0.000000000000000000, -0.1568667991644714932, 0.9876197685951274563 ) ) ;
#31923=VECTOR ( 'NONE', #171693, 1000.000000000000000 ) ;
#31924=DIRECTION ( 'NONE',  ( -1.000000000000000000, -2.952720810173289112E-16, 0.000000000000000000 ) ) ;
#31943=EDGE_CURVE ( 'NONE', #88270, #159975, #6362, .T. ) ;
#31990=AXIS2_PLACEMENT_3D ( 'NONE', #121344, #41792, #84700 ) ;
#32041=DIRECTION ( 'NONE',  ( 0.000000000000000000, 0.000000000000000000, -1.000000000000000000 ) ) ;
#32052=CARTESIAN_POINT ( 'NONE',  ( 21.12400222705966968, 8.778511907077053422, -12.25000000000000000 ) ) ;
#32077=AXIS2_PLACEMENT_3D ( 'NONE', #173732, #78416, #36776 ) ;
#32081=ORIENTED_EDGE ( 'NONE', *, *, #128666, .T. ) ;
#32116=EDGE_CURVE ( 'NONE', #122268, #62135, #244077, .T. ) ;
#32160=DIRECTION ( 'NONE',  ( 0.000000000000000000, 0.000000000000000000, 1.000000000000000000 ) ) ;
#32185=CARTESIAN_POINT ( 'NONE',  ( 21.05000000000000071, 0.000000000000000000, 0.000000000000000000 ) ) ;
#32192=CARTESIAN_POINT ( 'NONE',  ( -22.50000000000000000, 7.790779598373403836, 0.09999999999999939493 ) ) ;
#32211=ORIENTED_EDGE ( 'NONE', *, *, #53766, .T. ) ;
#32257=ORIENTED_EDGE ( 'NONE', *, *, #27578, .T. ) ;
#32303=AXIS2_PLACEMENT_3D ( 'NONE', #97693, #212556, #74350 ) ;
#32330=AXIS2_PLACEMENT_3D ( 'NONE', #26648, #142702, #85282 ) ;
#32343=CARTESIAN_POINT ( 'NONE',  ( 18.59999999999999076, 10.20857864376269575, -21.35000000000000142 ) ) ;
#32357=CARTESIAN_POINT ( 'NONE',  ( -22.39999999999999858, 0.000000000000000000, 11.64957080754479968 ) ) ;
#32369=EDGE_CURVE ( 'NONE', #75474, #196401, #135534, .T. ) ;
#32374=VERTEX_POINT ( 'NONE', #17047 ) ;
#32394=ORIENTED_EDGE ( 'NONE', *, *, #25635, .F. ) ;
#32396=CIRCLE ( 'NONE', #19906, 12.87499999999999822 ) ;
#32402=DIRECTION ( 'NONE',  ( -0.9880948137434723000, 0.1538461538461483591, -0.000000000000000000 ) ) ;
#32409=CARTESIAN_POINT ( 'NONE',  ( -23.15000000000000213, -11.48912529307605546, -30.39999999999999503 ) ) ;
#32421=CARTESIAN_POINT ( 'NONE',  ( -18.40000000000000213, -9.500000000000007105, -40.10018939122203818 ) ) ;
#32423=DIRECTION ( 'NONE',  ( -1.000000000000000000, 0.000000000000000000, 0.000000000000000000 ) ) ;
#32439=AXIS2_PLACEMENT_3D ( 'NONE', #93125, #132259, #154433 ) ;
#32462=EDGE_LOOP ( 'NONE', ( #44433, #48377, #118521, #70917 ) ) ;
#32468=CARTESIAN_POINT ( 'NONE',  ( 23.14999999999999858, 0.000000000000000000, -33.50000000000000000 ) ) ;
#32485=CARTESIAN_POINT ( 'NONE',  ( 18.44208962362730730, -9.552340496908351852, -40.34217305546407317 ) ) ;
#32490=DIRECTION ( 'NONE',  ( 0.000000000000000000, 0.000000000000000000, -1.000000000000000000 ) ) ;
#32536=ORIENTED_EDGE ( 'NONE', *, *, #221025, .T. ) ;
#32545=ORIENTED_EDGE ( 'NONE', *, *, #79324, .T. ) ;
#32549=VERTEX_POINT ( 'NONE', #142103 ) ;
#32554=VECTOR ( 'NONE', #72134, 1000.000000000000000 ) ;
#32592=DIRECTION ( 'NONE',  ( -1.000000000000000000, -1.836970198721029934E-16, 0.000000000000000000 ) ) ;
#32595=CARTESIAN_POINT ( 'NONE',  ( -18.59999999999999787, -9.499999999999998224, -12.15000000000000391 ) ) ;
#32596=ADVANCED_FACE ( 'NONE', ( #70308 ), #190230, .T. ) ;
#32601=DIRECTION ( 'NONE',  ( 1.000000000000000000, 0.000000000000000000, 0.000000000000000000 ) ) ;
#32640=DIRECTION ( 'NONE',  ( 0.000000000000000000, 0.8660254037844411501, 0.4999999999999956701 ) ) ;
#32660=EDGE_CURVE ( 'NONE', #167893, #69230, #102190, .T. ) ;
#32685=EDGE_CURVE ( 'NONE', #128006, #250275, #148397, .T. ) ;
#32693=CIRCLE ( 'NONE', #178417, 0.09999999999999939493 ) ;
#32710=EDGE_CURVE ( 'NONE', #26533, #41617, #76679, .T. ) ;
#32714=DIRECTION ( 'NONE',  ( -1.000000000000000000, 0.000000000000000000, 0.000000000000000000 ) ) ;
#32756=CARTESIAN_POINT ( 'NONE',  ( 21.00000000000000000, 9.749999999999998224, -12.25000000000000000 ) ) ;
#32767=VERTEX_POINT ( 'NONE', #72878 ) ;
#32788=ORIENTED_EDGE ( 'NONE', *, *, #143834, .F. ) ;
#32794=AXIS2_PLACEMENT_3D ( 'NONE', #155234, #258097, #234734 ) ;
#32841=EDGE_LOOP ( 'NONE', ( #13320, #71010, #35867, #99462 ) ) ;
#32887=VERTEX_POINT ( 'NONE', #122241 ) ;
#32946=DIRECTION ( 'NONE',  ( -3.265361837132813093E-16, 1.000000000000000000, 0.000000000000000000 ) ) ;
#32964=ORIENTED_EDGE ( 'NONE', *, *, #144379, .F. ) ;
#33002=LINE ( 'NONE', #9524, #121890 ) ;
#33027=CARTESIAN_POINT ( 'NONE',  ( 23.14999999999998437, 0.000000000000000000, 0.000000000000000000 ) ) ;
#33034=DIRECTION ( 'NONE',  ( 0.000000000000000000, 1.000000000000000000, 1.626303258728238113E-15 ) ) ;
#33057=ORIENTED_EDGE ( 'NONE', *, *, #192819, .F. ) ;
#33075=FACE_OUTER_BOUND ( 'NONE', #222777, .T. ) ;
#33119=AXIS2_PLACEMENT_3D ( 'NONE', #2471, #119898, #136858 ) ;
#33215=AXIS2_PLACEMENT_3D ( 'NONE', #55982, #135526, #215080 ) ;
#33225=PLANE ( 'NONE',  #57615 ) ;
#33238=ORIENTED_EDGE ( 'NONE', *, *, #230464, .F. ) ;
#33278=DIRECTION ( 'NONE',  ( 2.952720810173289112E-16, -1.000000000000000000, -0.000000000000000000 ) ) ;
#33292=VECTOR ( 'NONE', #71762, 1000.000000000000000 ) ;
#33335=EDGE_LOOP ( 'NONE', ( #163505, #131969, #96981, #150657 ) ) ;
#33350=CIRCLE ( 'NONE', #216648, 0.09999999999999939493 ) ;
#33361=AXIS2_PLACEMENT_3D ( 'NONE', #213258, #13788, #136269 ) ;
#33380=CARTESIAN_POINT ( 'NONE',  ( 21.05000000000000071, 10.72371681399907040, -7.594399235884193189 ) ) ;
#33424=CARTESIAN_POINT ( 'NONE',  ( -21.44999999999999929, 7.349999999999998757, -12.34999999999999964 ) ) ;
#33426=DIRECTION ( 'NONE',  ( 0.000000000000000000, 0.000000000000000000, -1.000000000000000000 ) ) ;
#33453=ORIENTED_EDGE ( 'NONE', *, *, #113681, .T. ) ;
#33485=EDGE_CURVE ( 'NONE', #138899, #169470, #7102, .T. ) ;
#33487=ORIENTED_EDGE ( 'NONE', *, *, #17806, .F. ) ;
#33502=CARTESIAN_POINT ( 'NONE',  ( -22.42357213249529124, 0.09908696400155765638, 7.672932386359936352 ) ) ;
#33536=VERTEX_POINT ( 'NONE', #209157 ) ;
#33598=CARTESIAN_POINT ( 'NONE',  ( 21.05000000000000071, 8.894723818377805458, -8.487084323149780118 ) ) ;
#33602=VERTEX_POINT ( 'NONE', #181301 ) ;
#33603=DIRECTION ( 'NONE',  ( -0.000000000000000000, -0.1298341882519737922, -0.9915357197604890427 ) ) ;
#33612=AXIS2_PLACEMENT_3D ( 'NONE', #71419, #248759, #12737 ) ;
#33624=CARTESIAN_POINT ( 'NONE',  ( 21.09706851349341861, 8.775842513473394391, -12.23556621639964703 ) ) ;
#33642=DIRECTION ( 'NONE',  ( -1.000000000000000000, 0.000000000000000000, 0.000000000000000000 ) ) ;
#33649=CARTESIAN_POINT ( 'NONE',  ( -23.15000000000000213, 5.900000000000005684, -23.28090023534362629 ) ) ;
#33658=AXIS2_PLACEMENT_3D ( 'NONE', #104756, #5661, #3101 ) ;
#33675=CARTESIAN_POINT ( 'NONE',  ( 23.14999999999999858, 4.898587196589414801E-16, -29.50000000000000355 ) ) ;
#33686=CARTESIAN_POINT ( 'NONE',  ( -22.50000000000000000, 0.09999999999999939493, 7.790779598373403836 ) ) ;
#33701=DIRECTION ( 'NONE',  ( 1.000000000000000000, -0.000000000000000000, -0.000000000000000000 ) ) ;
#33716=CIRCLE ( 'NONE', #233586, 0.09999999999999939493 ) ;
#33734=CIRCLE ( 'NONE', #50405, 7.800000000000001599 ) ;
#33737=AXIS2_PLACEMENT_3D ( 'NONE', #111863, #209672, #11485 ) ;
#33767=AXIS2_PLACEMENT_3D ( 'NONE', #103987, #66174, #242230 ) ;
#33789=AXIS2_PLACEMENT_3D ( 'NONE', #175674, #253898, #72742 ) ;
#33819=EDGE_CURVE ( 'NONE', #6556, #4734, #252981, .T. ) ;
#33824=ADVANCED_FACE ( 'NONE', ( #151154 ), #207283, .T. ) ;
#33847=CARTESIAN_POINT ( 'NONE',  ( -23.25000000000000000, -9.000000000000001776, -23.60603087734756045 ) ) ;
#33861=FACE_OUTER_BOUND ( 'NONE', #228291, .T. ) ;
#33862=ORIENTED_EDGE ( 'NONE', *, *, #83477, .T. ) ;
#33887=DIRECTION ( 'NONE',  ( -1.000000000000000000, 0.000000000000000000, 0.000000000000000000 ) ) ;
#33892=ORIENTED_EDGE ( 'NONE', *, *, #251385, .T. ) ;
#33921=DIRECTION ( 'NONE',  ( 1.000000000000000000, -0.000000000000000000, -0.000000000000000000 ) ) ;
#33930=VERTEX_POINT ( 'NONE', #37629 ) ;
#33935=CARTESIAN_POINT ( 'NONE',  ( 22.40736611211992368, 0.000000000000000000, 11.64957080754479968 ) ) ;
#33958=AXIS2_PLACEMENT_3D ( 'NONE', #162418, #106255, #101085 ) ;
#33959=DIRECTION ( 'NONE',  ( 3.265361837132813093E-16, -1.000000000000000000, -0.000000000000000000 ) ) ;
#33979=CARTESIAN_POINT ( 'NONE',  ( 21.14999999999999503, -0.1008583690987122083, 11.74956712348939192 ) ) ;
#33980=FACE_OUTER_BOUND ( 'NONE', #83384, .T. ) ;
#33986=ORIENTED_EDGE ( 'NONE', *, *, #82310, .F. ) ;
#33996=FACE_OUTER_BOUND ( 'NONE', #23469, .T. ) ;
#34001=CARTESIAN_POINT ( 'NONE',  ( 23.14999999999999147, 0.000000000000000000, 0.000000000000000000 ) ) ;
#34008=VECTOR ( 'NONE', #202948, 1000.000000000000114 ) ;
#34016=CARTESIAN_POINT ( 'NONE',  ( 20.94999999999999574, -1.360870587192041681, -8.072997927090961312 ) ) ;
#34017=ORIENTED_EDGE ( 'NONE', *, *, #153335, .T. ) ;
#34038=ORIENTED_EDGE ( 'NONE', *, *, #65832, .T. ) ;
#34040=ADVANCED_FACE ( 'NONE', ( #221353 ), #23203, .T. ) ;
#34041=CIRCLE ( 'NONE', #13163, 11.75000000000000000 ) ;
#34068=AXIS2_PLACEMENT_3D ( 'NONE', #96994, #98277, #17493 ) ;
#34102=CARTESIAN_POINT ( 'NONE',  ( -21.08479644141223019, 6.345038657731887355, 0.05855444256413715881 ) ) ;
#34143=CARTESIAN_POINT ( 'NONE',  ( 21.05000000000000071, -11.48912529307605546, -30.39999999999999503 ) ) ;
#34172=VERTEX_POINT ( 'NONE', #106538 ) ;
#34187=EDGE_CURVE ( 'NONE', #139796, #146959, #236585, .T. ) ;
#34215=CARTESIAN_POINT ( 'NONE',  ( -18.50000000000000000, 11.64999999999999680, -0.1000000000000028644 ) ) ;
#34225=AXIS2_PLACEMENT_3D ( 'NONE', #78389, #53700, #117528 ) ;
#34244=AXIS2_PLACEMENT_3D ( 'NONE', #120531, #57938, #80049 ) ;
#34254=ORIENTED_EDGE ( 'NONE', *, *, #171103, .T. ) ;
#34255=AXIS2_PLACEMENT_3D ( 'NONE', #108980, #128560, #210660 ) ;
#34259=DIRECTION ( 'NONE',  ( 1.000000000000000000, 2.952720810173289112E-16, -0.000000000000000000 ) ) ;
#34266=ADVANCED_FACE ( 'NONE', ( #175546, #210796 ), #36024, .F. ) ;
#34285=CARTESIAN_POINT ( 'NONE',  ( 18.49999999999999289, 11.75000000000000000, -24.85000000000000142 ) ) ;
#34291=B_SPLINE_CURVE_WITH_KNOTS ( 'NONE', 3,
 ( #209994, #170911, #30092, #50880, #206135, #130439, #52178, #147440, #249130, #10511 ),
 .UNSPECIFIED., .F., .F.,
 ( 4, 2, 2, 2, 4 ),
 ( 0.000000000000000000, 3.990160268012752048E-05, 7.980320536025504096E-05, 0.0001596064107205164245, 0.0003192128214410408721 ),
 .UNSPECIFIED. ) ;
#34299=FACE_OUTER_BOUND ( 'NONE', #216900, .T. ) ;
#34317=VERTEX_POINT ( 'NONE', #252471 ) ;
#34327=EDGE_CURVE ( 'NONE', #45832, #252532, #24235, .T. ) ;
#34336=CARTESIAN_POINT ( 'NONE',  ( 18.49999999999998934, 10.24999999999999822, -24.75000000000000000 ) ) ;
#34361=ADVANCED_FACE ( 'NONE', ( #235478 ), #206632, .F. ) ;
#34372=AXIS2_PLACEMENT_3D ( 'NONE', #31757, #205202, #10885 ) ;
#34380=EDGE_CURVE ( 'NONE', #3044, #129511, #94933, .T. ) ;
#34407=AXIS2_PLACEMENT_3D ( 'NONE', #108858, #168882, #28072 ) ;
#34414=EDGE_CURVE ( 'NONE', #33930, #92153, #49153, .T. ) ;
#34488=CARTESIAN_POINT ( 'NONE',  ( -18.50000000000000000, -9.500000000000005329, 11.75000000000000000 ) ) ;
#34493=ORIENTED_EDGE ( 'NONE', *, *, #60524, .F. ) ;
#34523=ORIENTED_EDGE ( 'NONE', *, *, #56466, .F. ) ;
#34546=ORIENTED_EDGE ( 'NONE', *, *, #90347, .T. ) ;
#34548=FACE_OUTER_BOUND ( 'NONE', #177826, .T. ) ;
#34554=AXIS2_PLACEMENT_3D ( 'NONE', #142567, #103434, #220830 ) ;
#34633=CARTESIAN_POINT ( 'NONE',  ( -22.39999999999999858, 11.75000000000000000, -3.469446951953614189E-15 ) ) ;
#34664=AXIS2_PLACEMENT_3D ( 'NONE', #256827, #118684, #15746 ) ;
#34685=DIRECTION ( 'NONE',  ( 0.000000000000000000, 0.1298341882520022694, 0.9915357197604852679 ) ) ;
#34723=EDGE_CURVE ( 'NONE', #93175, #109, #161151, .T. ) ;
#34755=CARTESIAN_POINT ( 'NONE',  ( 21.07094088545369104, 0.09889370255222153239, 6.320167221917142975 ) ) ;
#34786=DIRECTION ( 'NONE',  ( 1.000000000000000000, 0.000000000000000000, 0.000000000000000000 ) ) ;
#34829=ORIENTED_EDGE ( 'NONE', *, *, #24163, .F. ) ;
#34832=CARTESIAN_POINT ( 'NONE',  ( 21.05000000000000071, 11.75000000000000711, -26.48519422934605316 ) ) ;
#34833=DIRECTION ( 'NONE',  ( 0.000000000000000000, 0.9908441862701600211, 0.1350103645451876944 ) ) ;
#34853=VECTOR ( 'NONE', #194769, 1000.000000000000000 ) ;
#34862=CARTESIAN_POINT ( 'NONE',  ( 20.94999999999999929, 8.926614585087097709, -8.471683019223119615 ) ) ;
#34910=ORIENTED_EDGE ( 'NONE', *, *, #114602, .F. ) ;
#34918=DIRECTION ( 'NONE',  ( 0.000000000000000000, -2.005774019098195320E-13, 1.000000000000000000 ) ) ;
#34924=AXIS2_PLACEMENT_3D ( 'NONE', #7376, #204286, #166490 ) ;
#34954=CARTESIAN_POINT ( 'NONE',  ( 23.14999999999999858, 2.449293598294710852E-16, -31.50000000000000000 ) ) ;
#34967=AXIS2_PLACEMENT_3D ( 'NONE', #128148, #125564, #149006 ) ;
#34992=CARTESIAN_POINT ( 'NONE',  ( -18.47130263965434338, -9.471155585964025292, -40.18340476547687956 ) ) ;
#34998=EDGE_CURVE ( 'NONE', #20565, #145748, #207771, .T. ) ;
#35013=AXIS2_PLACEMENT_3D ( 'NONE', #133562, #18748, #35773 ) ;
#35030=EDGE_LOOP ( 'NONE', ( #83141, #62113, #103255, #195824 ) ) ;
#35038=CARTESIAN_POINT ( 'NONE',  ( 18.46947024752524769, -9.509297157156085589, -6.986689448697918081 ) ) ;
#35053=CARTESIAN_POINT ( 'NONE',  ( 18.44206774312970865, -9.491027357540085418, -40.12622750469819977 ) ) ;
#35077=DIRECTION ( 'NONE',  ( -0.000000000000000000, 0.1350103645451649625, -0.9908441862701631297 ) ) ;
#35083=CYLINDRICAL_SURFACE ( 'NONE', #172210, 0.09999999999999971412 ) ;
#35087=ORIENTED_EDGE ( 'NONE', *, *, #15082, .F. ) ;
#35093=ADVANCED_FACE ( 'NONE', ( #242933 ), #219512, .F. ) ;
#35184=EDGE_CURVE ( 'NONE', #210177, #47156, #57876, .T. ) ;
#35202=PLANE ( 'NONE',  #125691 ) ;
#35252=CARTESIAN_POINT ( 'NONE',  ( 18.49999999999999289, 10.20857864608310273, -24.70250686562995668 ) ) ;
#35266=EDGE_CURVE ( 'NONE', #199045, #164389, #20317, .T. ) ;
#35273=DIRECTION ( 'NONE',  ( -1.000000000000000000, -0.000000000000000000, -0.000000000000000000 ) ) ;
#35338=CARTESIAN_POINT ( 'NONE',  ( -23.25000000000000000, 0.000000000000000000, -33.50000000000000000 ) ) ;
#35366=LINE ( 'NONE', #212689, #184332 ) ;
#35385=ADVANCED_FACE ( 'NONE', ( #197081 ), #158017, .F. ) ;
#35393=CARTESIAN_POINT ( 'NONE',  ( 20.95512820512820440, 10.62384868371188062, -7.664913569087605794 ) ) ;
#35398=ADVANCED_FACE ( 'NONE', ( #173734 ), #212817, .F. ) ;
#35409=EDGE_CURVE ( 'NONE', #207337, #15628, #158095, .T. ) ;
#35416=AXIS2_PLACEMENT_3D ( 'NONE', #76315, #196280, #60609 ) ;
#35424=EDGE_CURVE ( 'NONE', #56815, #74339, #178755, .T. ) ;
#35462=AXIS2_PLACEMENT_3D ( 'NONE', #136586, #38799, #2208 ) ;
#35473=EDGE_LOOP ( 'NONE', ( #107809, #116251, #153518 ) ) ;
#35545=ORIENTED_EDGE ( 'NONE', *, *, #65882, .F. ) ;
#35557=DIRECTION ( 'NONE',  ( 1.000000000000000000, 0.000000000000000000, 0.000000000000000000 ) ) ;
#35571=EDGE_CURVE ( 'NONE', #197037, #118795, #153820, .T. ) ;
#35575=EDGE_CURVE ( 'NONE', #224018, #8661, #27159, .T. ) ;
#35585=DIRECTION ( 'NONE',  ( -0.000000000000000000, 0.01283462868039629209, -0.9999176327611372095 ) ) ;
#35592=CARTESIAN_POINT ( 'NONE',  ( -18.59999999999999787, -1.835859311443637010, -45.10443916879852821 ) ) ;
#35598=CARTESIAN_POINT ( 'NONE',  ( 21.05000000000000071, 0.000000000000000000, 0.000000000000000000 ) ) ;
#35600=CARTESIAN_POINT ( 'NONE',  ( 22.50014994444007499, 11.74971973189203744, 0.08308015671907631461 ) ) ;
#35620=CARTESIAN_POINT ( 'NONE',  ( -18.50000000000000000, -9.419084502813289461, -40.32990780702540690 ) ) ;
#35625=FACE_OUTER_BOUND ( 'NONE', #237316, .T. ) ;
#35631=EDGE_CURVE ( 'NONE', #88943, #120640, #228785, .T. ) ;
#35667=ORIENTED_EDGE ( 'NONE', *, *, #174143, .F. ) ;
#35675=EDGE_LOOP ( 'NONE', ( #173577, #103307, #112416, #16467 ) ) ;
#35684=DIRECTION ( 'NONE',  ( 1.000000000000000000, 1.836970198721029934E-16, -0.000000000000000000 ) ) ;
#35685=CARTESIAN_POINT ( 'NONE',  ( -23.25000000000000000, 0.000000000000000000, -33.50000000000000000 ) ) ;
#35723=DIRECTION ( 'NONE',  ( 1.000000000000000000, 0.000000000000000000, 0.000000000000000000 ) ) ;
#35773=DIRECTION ( 'NONE',  ( 1.000000000000000000, 0.000000000000000000, 0.000000000000000000 ) ) ;
#35814=CARTESIAN_POINT ( 'NONE',  ( 21.11701782572533048, 10.72160911600745692, -12.24503742951121055 ) ) ;
#35827=CARTESIAN_POINT ( 'NONE',  ( -23.15000000000000213, 11.65000000000000036, -26.48519422934604961 ) ) ;
#35836=VECTOR ( 'NONE', #222744, 1000.000000000000000 ) ;
#35842=CARTESIAN_POINT ( 'NONE',  ( 20.94999999999999929, 0.000000000000000000, -35.50000000000000711 ) ) ;
#35860=ORIENTED_EDGE ( 'NONE', *, *, #97773, .T. ) ;
#35867=ORIENTED_EDGE ( 'NONE', *, *, #21925, .F. ) ;
#35869=DIRECTION ( 'NONE',  ( 0.000000000000000000, 1.000000000000000000, 0.000000000000000000 ) ) ;
#35890=SPHERICAL_SURFACE ( 'NONE', #107827, 0.1000000000000000056 ) ;
#35897=CARTESIAN_POINT ( 'NONE',  ( 21.04999999999999716, 8.871279685995643760, -12.15000000000000036 ) ) ;
#35905=DIRECTION ( 'NONE',  ( 0.000000000000000000, 1.000000000000000000, 0.000000000000000000 ) ) ;
#35950=DIRECTION ( 'NONE',  ( -1.000000000000000000, -2.952720810173289112E-16, 0.000000000000000000 ) ) ;
#35965=FACE_OUTER_BOUND ( 'NONE', #95354, .T. ) ;
#35994=ORIENTED_EDGE ( 'NONE', *, *, #189081, .F. ) ;
#36018=CARTESIAN_POINT ( 'NONE',  ( -18.50000000000000000, 3.912899247233453615, -11.48182297301096888 ) ) ;
#36021=EDGE_LOOP ( 'NONE', ( #114652, #216989, #69435 ) ) ;
#36024=PLANE ( 'NONE',  #232349 ) ;
#36036=FACE_OUTER_BOUND ( 'NONE', #235665, .T. ) ;
#36037=LINE ( 'NONE', #75174, #92825 ) ;
#36044=PLANE ( 'NONE',  #31318 ) ;
#36073=DIRECTION ( 'NONE',  ( 0.000000000000000000, 1.776356839400250859E-15, -1.000000000000000000 ) ) ;
#36077=AXIS2_PLACEMENT_3D ( 'NONE', #20780, #199417, #122434 ) ;
#36103=CARTESIAN_POINT ( 'NONE',  ( -18.58671080940900211, -9.406932858826619892, -7.124154464904687956 ) ) ;
#36114=DIRECTION ( 'NONE',  ( -1.000000000000000000, 0.000000000000000000, -0.000000000000000000 ) ) ;
#36117=ORIENTED_EDGE ( 'NONE', *, *, #30394, .T. ) ;
#36138=EDGE_LOOP ( 'NONE', ( #107544, #233552, #222554, #137575 ) ) ;
#36140=CARTESIAN_POINT ( 'NONE',  ( 23.14999999999999858, 0.000000000000000000, 0.000000000000000000 ) ) ;
#36175=ORIENTED_EDGE ( 'NONE', *, *, #4497, .F. ) ;
#36215=EDGE_CURVE ( 'NONE', #26533, #199652, #86894, .T. ) ;
#36259=TOROIDAL_SURFACE ( 'NONE', #23798, 11.70000000000000462, 0.1000000000000000056 ) ;
#36281=CARTESIAN_POINT ( 'NONE',  ( 21.05000000000000071, -0.09999993530598326463, 6.478078221094742517 ) ) ;
#36293=DIRECTION ( 'NONE',  ( 0.000000000000000000, 0.000000000000000000, 1.000000000000000000 ) ) ;
#36296=ORIENTED_EDGE ( 'NONE', *, *, #257764, .F. ) ;
#36300=DIRECTION ( 'NONE',  ( 1.000000000000000000, -7.304098846218134667E-16, 4.607487905232622991E-31 ) ) ;
#36305=CARTESIAN_POINT ( 'NONE',  ( 20.94999999999999929, -9.400000000000000355, -23.60603087734755690 ) ) ;
#36316=CIRCLE ( 'NONE', #248680, 0.09999999999999999167 ) ;
#36339=ORIENTED_EDGE ( 'NONE', *, *, #25799, .T. ) ;
#36360=CARTESIAN_POINT ( 'NONE',  ( 20.94999999999999929, 0.000000000000000000, -33.50000000000000000 ) ) ;
#36374=DIRECTION ( 'NONE',  ( 1.000000000000000000, 0.000000000000000000, -0.000000000000000000 ) ) ;
#36380=CARTESIAN_POINT ( 'NONE',  ( -20.64999999999999858, 1.999999999999998224, -20.67537807723790166 ) ) ;
#36387=VERTEX_POINT ( 'NONE', #107317 ) ;
#36393=AXIS2_PLACEMENT_3D ( 'NONE', #26212, #105700, #62757 ) ;
#36400=EDGE_CURVE ( 'NONE', #178738, #13860, #116166, .T. ) ;
#36425=CARTESIAN_POINT ( 'NONE',  ( 21.05000000000000071, 8.876614585087098774, -8.385080478844676222 ) ) ;
#36479=CARTESIAN_POINT ( 'NONE',  ( 20.22516295850462598, 9.899364295449302631, -7.910065712091376433 ) ) ;
#36505=CARTESIAN_POINT ( 'NONE',  ( 20.85000000000000142, 0.000000000000000000, -41.40000000000000568 ) ) ;
#36534=AXIS2_PLACEMENT_3D ( 'NONE', #224920, #247054, #11034 ) ;
#36561=AXIS2_PLACEMENT_3D ( 'NONE', #172248, #152671, #53538 ) ;
#36591=ORIENTED_EDGE ( 'NONE', *, *, #119729, .T. ) ;
#36594=AXIS2_PLACEMENT_3D ( 'NONE', #227942, #210949, #111852 ) ;
#36597=VECTOR ( 'NONE', #146582, 1000.000000000000000 ) ;
#36604=LINE ( 'NONE', #70593, #180655 ) ;
#36628=CARTESIAN_POINT ( 'NONE',  ( -18.59999999999999787, 5.341242989991650703, 9.806650206488024324 ) ) ;
#36648=CIRCLE ( 'NONE', #86465, 11.65000000000000036 ) ;
#36663=CARTESIAN_POINT ( 'NONE',  ( 18.59999999999999787, 0.000000000000000000, 0.000000000000000000 ) ) ;
#36671=CARTESIAN_POINT ( 'NONE',  ( 19.97071067811864609, 11.72071067811865674, -24.65000000000000213 ) ) ;
#36688=AXIS2_PLACEMENT_3D ( 'NONE', #116691, #18872, #160977 ) ;
#36694=DIRECTION ( 'NONE',  ( -1.000000000000000000, 0.000000000000000000, 0.000000000000000000 ) ) ;
#36709=AXIS2_PLACEMENT_3D ( 'NONE', #165156, #189551, #66043 ) ;
#36710=EDGE_LOOP ( 'NONE', ( #83037, #61671, #35994, #22539 ) ) ;
#36722=ORIENTED_EDGE ( 'NONE', *, *, #194198, .T. ) ;
#36725=AXIS2_PLACEMENT_3D ( 'NONE', #115536, #215905, #111696 ) ;
#36744=ORIENTED_EDGE ( 'NONE', *, *, #25762, .T. ) ;
#36776=DIRECTION ( 'NONE',  ( 0.000000000000000000, 0.000000000000000000, 1.000000000000000000 ) ) ;
#36788=ORIENTED_EDGE ( 'NONE', *, *, #127046, .F. ) ;
#36819=CARTESIAN_POINT ( 'NONE',  ( -23.25000000000000000, 0.000000000000000000, -33.50000000000000000 ) ) ;
#36827=CIRCLE ( 'NONE', #99301, 0.6000000000000015321 ) ;
#36858=AXIS2_PLACEMENT_3D ( 'NONE', #239484, #41305, #120845 ) ;
#36862=TOROIDAL_SURFACE ( 'NONE', #24370, 11.65000000000000036, 0.1000000000000000056 ) ;
#36880=AXIS2_PLACEMENT_3D ( 'NONE', #250678, #108608, #146429 ) ;
#36894=DIRECTION ( 'NONE',  ( 1.000000000000000000, 0.000000000000000000, -0.000000000000000000 ) ) ;
#36909=ORIENTED_EDGE ( 'NONE', *, *, #234368, .F. ) ;
#36922=DIRECTION ( 'NONE',  ( 0.000000000000000000, 0.000000000000000000, 1.000000000000000000 ) ) ;
#36927=AXIS2_PLACEMENT_3D ( 'NONE', #42748, #122291, #44035 ) ;
#36963=CIRCLE ( 'NONE', #215959, 0.09999999999999939493 ) ;
#37010=VERTEX_POINT ( 'NONE', #235949 ) ;
#37029=ORIENTED_EDGE ( 'NONE', *, *, #78697, .T. ) ;
#37045=ADVANCED_FACE ( 'NONE', ( #58586 ), #4081, .T. ) ;
#37054=ADVANCED_FACE ( 'NONE', ( #100274 ), #203805, .T. ) ;
#37072=EDGE_CURVE ( 'NONE', #31770, #221017, #8193, .T. ) ;
#37079=AXIS2_PLACEMENT_3D ( 'NONE', #191698, #235906, #15622 ) ;
#37084=AXIS2_PLACEMENT_3D ( 'NONE', #66875, #108571, #51133 ) ;
#37095=CARTESIAN_POINT ( 'NONE',  ( -18.59999999999999787, 0.000000000000000000, -33.50000000000000000 ) ) ;
#37131=CARTESIAN_POINT ( 'NONE',  ( -21.53699400384793705, -1.597579023731851126E-12, 6.787711793239012081 ) ) ;
#37143=CARTESIAN_POINT ( 'NONE',  ( -18.59999999999999787, 7.070967871798842452, -37.24656422186831151 ) ) ;
#37144=FACE_OUTER_BOUND ( 'NONE', #221287, .T. ) ;
#37156=CARTESIAN_POINT ( 'NONE',  ( -18.59999999999999787, -1.162701749938009677, -8.099999999999999645 ) ) ;
#37163=DIRECTION ( 'NONE',  ( 0.000000000000000000, 0.000000000000000000, -1.000000000000000000 ) ) ;
#37174=CARTESIAN_POINT ( 'NONE',  ( 18.55857864376267941, 10.36715728752537835, -24.75000000000000355 ) ) ;
#37186=AXIS2_PLACEMENT_3D ( 'NONE', #1186, #78158, #238531 ) ;
#37192=VECTOR ( 'NONE', #159307, 1000.000000000000000 ) ;
#37207=EDGE_LOOP ( 'NONE', ( #103039, #162411, #142885, #237950 ) ) ;
#37260=FACE_OUTER_BOUND ( 'NONE', #27450, .T. ) ;
#37301=AXIS2_PLACEMENT_3D ( 'NONE', #137069, #39281, #3973 ) ;
#37311=CARTESIAN_POINT ( 'NONE',  ( 21.07016717457011623, -5.802175688691957323E-16, 6.320940838100908010 ) ) ;
#37322=AXIS2_PLACEMENT_3D ( 'NONE', #252730, #74144, #248909 ) ;
#37327=CARTESIAN_POINT ( 'NONE',  ( -18.59999999999999787, -1.249999999999999334, -8.000000000000000000 ) ) ;
#37333=CARTESIAN_POINT ( 'NONE',  ( -18.50000000000000000, 7.021664781900089913, -37.33356540189728889 ) ) ;
#37342=CARTESIAN_POINT ( 'NONE',  ( -23.15000000000000213, -11.65000000000000036, 3.469446951953614189E-15 ) ) ;
#37387=ORIENTED_EDGE ( 'NONE', *, *, #251071, .T. ) ;
#37424=VECTOR ( 'NONE', #234773, 1000.000000000000000 ) ;
#37427=EDGE_CURVE ( 'NONE', #106654, #66484, #33350, .T. ) ;
#37462=DIRECTION ( 'NONE',  ( 1.000000000000000000, 0.000000000000000000, 0.000000000000000000 ) ) ;
#37463=ORIENTED_EDGE ( 'NONE', *, *, #122168, .T. ) ;
#37468=CIRCLE ( 'NONE', #162360, 0.09999999999999939493 ) ;
#37495=EDGE_LOOP ( 'NONE', ( #254727, #28874, #162662, #163960 ) ) ;
#37534=AXIS2_PLACEMENT_3D ( 'NONE', #217381, #23078, #60882 ) ;
#37536=CARTESIAN_POINT ( 'NONE',  ( 21.05000000000000071, 6.540656951701244282, -9.351243737687475743E-16 ) ) ;
#37557=CARTESIAN_POINT ( 'NONE',  ( 21.13435531349779239, -1.328411718110899122E-15, 6.493721063592196252 ) ) ;
#37580=CARTESIAN_POINT ( 'NONE',  ( 18.50000000000000355, -9.421456145495524126, -7.241982084019278787 ) ) ;
#37612=LINE ( 'NONE', #175842, #94868 ) ;
#37629=CARTESIAN_POINT ( 'NONE',  ( 21.05000000000000071, 0.000000000000000000, 4.300000000000032685 ) ) ;
#37630=DIRECTION ( 'NONE',  ( -1.000000000000000000, -0.000000000000000000, -0.000000000000000000 ) ) ;
#37653=DIRECTION ( 'NONE',  ( 0.000000000000000000, -1.000000000000000000, 0.000000000000000000 ) ) ;
#37658=DIRECTION ( 'NONE',  ( 0.000000000000000000, -1.000000000000000000, 0.000000000000000000 ) ) ;
#37659=AXIS2_PLACEMENT_3D ( 'NONE', #92282, #109271, #229249 ) ;
#37757=CARTESIAN_POINT ( 'NONE',  ( 20.75572585718224872, 8.882316728398945926, -8.497258398706687643 ) ) ;
#37779=DIRECTION ( 'NONE',  ( -3.265361837132813093E-16, 1.000000000000000000, 0.000000000000000000 ) ) ;
#37793=VECTOR ( 'NONE', #150464, 1000.000000000000000 ) ;
#37807=ADVANCED_FACE ( 'NONE', ( #216733 ), #156800, .T. ) ;
#37811=CARTESIAN_POINT ( 'NONE',  ( 18.49999999999999289, 10.49142135623730709, -24.85000000000000142 ) ) ;
#37824=ORIENTED_EDGE ( 'NONE', *, *, #251905, .F. ) ;
#37829=DIRECTION ( 'NONE',  ( 0.000000000000000000, 0.000000000000000000, 1.000000000000000000 ) ) ;
#37835=ORIENTED_EDGE ( 'NONE', *, *, #41119, .F. ) ;
#37849=ORIENTED_EDGE ( 'NONE', *, *, #139456, .F. ) ;
#37872=VERTEX_POINT ( 'NONE', #220599 ) ;
#37885=CARTESIAN_POINT ( 'NONE',  ( -20.64999999999999858, 2.326828918379974323E-16, -31.59999999999999787 ) ) ;
#37889=ORIENTED_EDGE ( 'NONE', *, *, #185399, .F. ) ;
#37910=EDGE_LOOP ( 'NONE', ( #42618, #130167, #168519, #202299 ) ) ;
#37932=DIRECTION ( 'NONE',  ( -0.000000000000000000, -0.000000000000000000, 1.000000000000000000 ) ) ;
#37945=CARTESIAN_POINT ( 'NONE',  ( 20.95576188350343116, 10.60898054496340137, -7.611233722754299436 ) ) ;
#37960=EDGE_CURVE ( 'NONE', #251285, #155798, #137884, .T. ) ;
#37968=VECTOR ( 'NONE', #190575, 1000.000000000000000 ) ;
#37988=CYLINDRICAL_SURFACE ( 'NONE', #256239, 0.09999999999999939493 ) ;
#38045=CARTESIAN_POINT ( 'NONE',  ( -23.15000000000000213, 1.999999999999998224, -20.87537807723790095 ) ) ;
#38053=ORIENTED_EDGE ( 'NONE', *, *, #108515, .F. ) ;
#38058=EDGE_LOOP ( 'NONE', ( #207533, #222931, #134196, #164091 ) ) ;
#38069=VECTOR ( 'NONE', #56505, 1000.000000000000000 ) ;
#38090=DIRECTION ( 'NONE',  ( 0.000000000000000000, 0.000000000000000000, -1.000000000000000000 ) ) ;
#38093=ORIENTED_EDGE ( 'NONE', *, *, #119979, .F. ) ;
#38106=EDGE_CURVE ( 'NONE', #11036, #220463, #141998, .T. ) ;
#38116=CYLINDRICAL_SURFACE ( 'NONE', #156402, 0.09999999999999811817 ) ;
#38122=ADVANCED_FACE ( 'NONE', ( #165300 ), #161473, .T. ) ;
#38135=EDGE_CURVE ( 'NONE', #130475, #87594, #349, .T. ) ;
#38155=CIRCLE ( 'NONE', #67168, 0.09999999999999939493 ) ;
#38168=ORIENTED_EDGE ( 'NONE', *, *, #4497, .T. ) ;
#38171=CIRCLE ( 'NONE', #104741, 7.791421356237316687 ) ;
#38195=ORIENTED_EDGE ( 'NONE', *, *, #241298, .F. ) ;
#38240=ORIENTED_EDGE ( 'NONE', *, *, #62626, .T. ) ;
#38241=AXIS2_PLACEMENT_3D ( 'NONE', #29832, #225411, #10250 ) ;
#38243=EDGE_LOOP ( 'NONE', ( #93638, #93287, #198045, #122876 ) ) ;
#38248=EDGE_CURVE ( 'NONE', #4098, #135260, #170492, .T. ) ;
#38261=EDGE_CURVE ( 'NONE', #17816, #208385, #246061, .T. ) ;
#38296=CIRCLE ( 'NONE', #151309, 0.09999999999999939493 ) ;
#38328=CIRCLE ( 'NONE', #159156, 2.000000000000001776 ) ;
#38332=DIRECTION ( 'NONE',  ( 1.000000000000000000, 0.000000000000000000, 0.000000000000000000 ) ) ;
#38365=CARTESIAN_POINT ( 'NONE',  ( 21.09696443733127325, 10.72400988391847676, -12.23477752704822130 ) ) ;
#38380=VERTEX_POINT ( 'NONE', #233002 ) ;
#38393=CARTESIAN_POINT ( 'NONE',  ( -22.00356870068735660, -2.403239590344364268E-12, 7.254242361757839319 ) ) ;
#38397=EDGE_CURVE ( 'NONE', #137697, #10751, #14140, .T. ) ;
#38417=CARTESIAN_POINT ( 'NONE',  ( -20.94999999999999929, 11.69999999999999574, -26.74500185048138334 ) ) ;
#38418=EDGE_CURVE ( 'NONE', #26537, #176380, #184337, .T. ) ;
#38421=DIRECTION ( 'NONE',  ( 0.000000000000000000, 0.000000000000000000, -1.000000000000000000 ) ) ;
#38437=DIRECTION ( 'NONE',  ( -1.000000000000000000, -0.000000000000000000, -0.000000000000000000 ) ) ;
#38491=DIRECTION ( 'NONE',  ( -1.000000000000000000, 0.000000000000000000, 0.000000000000000000 ) ) ;
#38530=CARTESIAN_POINT ( 'NONE',  ( 23.15000000000000213, -8.596261682242985813, -24.04987248284971812 ) ) ;
#38563=DIRECTION ( 'NONE',  ( 0.000000000000000000, 1.000000000000000000, 0.000000000000000000 ) ) ;
#38586=ORIENTED_EDGE ( 'NONE', *, *, #194959, .T. ) ;
#38588=CARTESIAN_POINT ( 'NONE',  ( 18.59999999999998721, 6.846123162352588665, -37.23772626684986164 ) ) ;
#38595=ORIENTED_EDGE ( 'NONE', *, *, #29878, .T. ) ;
#38615=CARTESIAN_POINT ( 'NONE',  ( 20.94999999999999574, -11.64999999999999147, -3.000000000000002665 ) ) ;
#38655=EDGE_LOOP ( 'NONE', ( #65974, #17431, #161496, #151413 ) ) ;
#38660=VERTEX_POINT ( 'NONE', #63110 ) ;
#38675=AXIS2_PLACEMENT_3D ( 'NONE', #183241, #201504, #84075 ) ;
#38711=CARTESIAN_POINT ( 'NONE',  ( -22.39999999999999858, 11.65000000000000036, 0.09999999999999592548 ) ) ;
#38744=ORIENTED_EDGE ( 'NONE', *, *, #65496, .T. ) ;
#38770=EDGE_LOOP ( 'NONE', ( #251893, #249151, #167261 ) ) ;
#38799=DIRECTION ( 'NONE',  ( 0.000000000000000000, 0.000000000000000000, -1.000000000000000000 ) ) ;
#38816=CARTESIAN_POINT ( 'NONE',  ( -20.64999999999999858, 2.399999999999999467, -20.27537807723789953 ) ) ;
#38841=CIRCLE ( 'NONE', #142845, 0.09999999999999939493 ) ;
#38861=CARTESIAN_POINT ( 'NONE',  ( 18.54147908293617775, -9.463261657928100590, -7.048948896755796945 ) ) ;
#38874=ORIENTED_EDGE ( 'NONE', *, *, #202106, .F. ) ;
#38903=AXIS2_PLACEMENT_3D ( 'NONE', #88289, #171745, #54316 ) ;
#38910=EDGE_LOOP ( 'NONE', ( #160492, #53391, #79954, #37463 ) ) ;
#38914=CARTESIAN_POINT ( 'NONE',  ( 20.94999999999999929, -8.730841121495322099, -23.90192528101566438 ) ) ;
#38934=CIRCLE ( 'NONE', #118026, 11.65000000000000036 ) ;
#38943=CARTESIAN_POINT ( 'NONE',  ( -21.14250536705909411, -1.950243336657294609E-16, 6.518172176880757895 ) ) ;
#38975=FACE_OUTER_BOUND ( 'NONE', #23122, .T. ) ;
#38994=CIRCLE ( 'NONE', #150829, 0.09999999999999967248 ) ;
#38995=TOROIDAL_SURFACE ( 'NONE', #184708, 0.4000000000000003553, 0.1000000000000000056 ) ;
#39034=CARTESIAN_POINT ( 'NONE',  ( 20.53930447207976684, 8.977148687524273640, -8.442507141577925367 ) ) ;
#39037=CARTESIAN_POINT ( 'NONE',  ( 20.85000000000000142, 0.000000000000000000, -41.30000000000000426 ) ) ;
#39052=VERTEX_POINT ( 'NONE', #35592 ) ;
#39083=DIRECTION ( 'NONE',  ( 1.000000000000000000, -0.000000000000000000, -0.000000000000000000 ) ) ;
#39087=CARTESIAN_POINT ( 'NONE',  ( 21.05000000000000071, 0.000000000000000000, -33.50000000000000000 ) ) ;
#39103=DIRECTION ( 'NONE',  ( 0.000000000000000000, 0.000000000000000000, -1.000000000000000000 ) ) ;
#39113=EDGE_CURVE ( 'NONE', #104459, #210671, #141087, .T. ) ;
#39141=DIRECTION ( 'NONE',  ( -0.7071067811865389130, 0.000000000000000000, 0.7071067811865561215 ) ) ;
#39143=DIRECTION ( 'NONE',  ( 0.000000000000000000, 0.000000000000000000, 1.000000000000000000 ) ) ;
#39150=DIRECTION ( 'NONE',  ( -2.978066053179067751E-16, 1.000000000000000000, 0.000000000000000000 ) ) ;
#39182=DIRECTION ( 'NONE',  ( 1.000000000000000000, -0.000000000000000000, -0.000000000000000000 ) ) ;
#39188=AXIS2_PLACEMENT_3D ( 'NONE', #221671, #23534, #139567 ) ;
#39195=CARTESIAN_POINT ( 'NONE',  ( 21.08376601933332495, 6.341947271275658160, 0.06377601093000156984 ) ) ;
#39204=DIRECTION ( 'NONE',  ( -1.000000000000000000, 0.000000000000000000, 0.000000000000000000 ) ) ;
#39233=CARTESIAN_POINT ( 'NONE',  ( 20.95575313997065336, 10.61455330327483537, -7.621290701944819723 ) ) ;
#39240=ORIENTED_EDGE ( 'NONE', *, *, #113681, .F. ) ;
#39250=ORIENTED_EDGE ( 'NONE', *, *, #216352, .T. ) ;
#39275=DIRECTION ( 'NONE',  ( 1.000000000000000000, 0.000000000000000000, 0.000000000000000000 ) ) ;
#39281=DIRECTION ( 'NONE',  ( -4.336808689941752679E-15, 0.8660254037844482555, 0.4999999999999837907 ) ) ;
#39295=ORIENTED_EDGE ( 'NONE', *, *, #93888, .F. ) ;
#39307=ORIENTED_EDGE ( 'NONE', *, *, #81527, .T. ) ;
#39353=AXIS2_PLACEMENT_3D ( 'NONE', #175066, #149051, #169927 ) ;
#39386=DIRECTION ( 'NONE',  ( -1.000000000000000000, -0.000000000000000000, 0.000000000000000000 ) ) ;
#39423=ORIENTED_EDGE ( 'NONE', *, *, #120739, .T. ) ;
#39454=CARTESIAN_POINT ( 'NONE',  ( 22.57320508075688537, 11.75000000000000000, 4.930004492955712146E-16 ) ) ;
#39469=VERTEX_POINT ( 'NONE', #255530 ) ;
#39470=CARTESIAN_POINT ( 'NONE',  ( -18.42637059832564361, -9.496945461889701789, -40.10907730979983654 ) ) ;
#39480=( BOUNDED_SURFACE ( )  B_SPLINE_SURFACE ( 3, 2, ( 
 ( #71413, #115654, #34862 ),
 ( #209619, #33598, #16568 ),
 ( #110509, #250027, #170549 ),
 ( #96067, #132655, #213462 ) ),
 .UNSPECIFIED., .F., .F., .F. ) 
 B_SPLINE_SURFACE_WITH_KNOTS ( ( 4, 4 ),
 ( 3, 3 ),
 ( 0.0002700421466196735562, 0.0004789321604330922682 ),
 ( 0.000000000000000000, 1.000000000000000000 ),
 .UNSPECIFIED. ) 
 GEOMETRIC_REPRESENTATION_ITEM ( )  RATIONAL_B_SPLINE_SURFACE ( (
 ( 1.000000000000000000, 0.7071067811865475727, 1.000000000000000000),
 ( 1.000000000000000000, 0.7163411249511749679, 1.000000000000000000),
 ( 1.000000000000000000, 0.7221957104841917330, 1.000000000000000000),
 ( 1.000000000000000000, 0.7250110520819876836, 1.000000000000000000) ) ) 
 REPRESENTATION_ITEM ( '' )  SURFACE ( )  );
#39493=ORIENTED_EDGE ( 'NONE', *, *, #225795, .F. ) ;
#39517=CIRCLE ( 'NONE', #76884, 0.09999999999999939493 ) ;
#39522=EDGE_CURVE ( 'NONE', #171717, #122037, #187621, .T. ) ;
#39534=ORIENTED_EDGE ( 'NONE', *, *, #194647, .T. ) ;
#39559=DIRECTION ( 'NONE',  ( -0.000000000000000000, -0.9887567792719339499, -0.1495327102803676589 ) ) ;
#39560=VECTOR ( 'NONE', #155371, 1000.000000000000000 ) ;
#39580=CIRCLE ( 'NONE', #23006, 0.09999999999999939493 ) ;
#39585=EDGE_LOOP ( 'NONE', ( #134600, #175889, #38595, #196617 ) ) ;
#39603=CARTESIAN_POINT ( 'NONE',  ( 21.14999999999999858, -11.75000000000000000, -12.25000000000000000 ) ) ;
#39613=DIRECTION ( 'NONE',  ( 0.000000000000000000, -8.881784197001250746E-15, 1.000000000000000000 ) ) ;
#39624=DIRECTION ( 'NONE',  ( -0.000000000000000000, 1.000000000000000000, 0.000000000000000000 ) ) ;
#39647=ORIENTED_EDGE ( 'NONE', *, *, #38261, .F. ) ;
#39651=CARTESIAN_POINT ( 'NONE',  ( -23.25000000000000000, -1.149570369575693807, -41.31591248450196474 ) ) ;
#39659=CARTESIAN_POINT ( 'NONE',  ( 23.24999999999999289, 4.149999999999999467, 5.082284216461512198E-16 ) ) ;
#39665=CARTESIAN_POINT ( 'NONE',  ( -23.15000000000000213, 0.000000000000000000, 0.000000000000000000 ) ) ;
#39678=CARTESIAN_POINT ( 'NONE',  ( 22.47071067811865319, 7.720074744498043096, 0.09909245470260744093 ) ) ;
#39680=AXIS2_PLACEMENT_3D ( 'NONE', #146971, #205666, #209533 ) ;
#39704=CARTESIAN_POINT ( 'NONE',  ( -21.07016717457011268, -5.827586677109586333E-16, 6.320940838100898240 ) ) ;
#39707=FACE_OUTER_BOUND ( 'NONE', #65017, .T. ) ;
#39711=CARTESIAN_POINT ( 'NONE',  ( -21.65000000000000213, 7.708578643762696636, -12.25000000000000000 ) ) ;
#39716=ORIENTED_EDGE ( 'NONE', *, *, #56135, .T. ) ;
#39739=EDGE_CURVE ( 'NONE', #241011, #32549, #194046, .T. ) ;
#39757=CARTESIAN_POINT ( 'NONE',  ( 20.95512820512820440, 8.876151316288114046, -12.15000000000000036 ) ) ;
#39765=CARTESIAN_POINT ( 'NONE',  ( -21.05000000000000071, -1.162701749938009677, -8.000000000000000000 ) ) ;
#39769=DIRECTION ( 'NONE',  ( 1.000000000000000000, -0.000000000000000000, -0.000000000000000000 ) ) ;
#39799=ORIENTED_EDGE ( 'NONE', *, *, #221673, .F. ) ;
#39838=ORIENTED_EDGE ( 'NONE', *, *, #8078, .F. ) ;
#39913=CARTESIAN_POINT ( 'NONE',  ( -20.85000000000000142, -1.164121893241208960, -41.41484808557160591 ) ) ;
#39914=EDGE_LOOP ( 'NONE', ( #22482, #836, #169903, #224214 ) ) ;
#39916=ORIENTED_EDGE ( 'NONE', *, *, #245097, .T. ) ;
#39919=ORIENTED_EDGE ( 'NONE', *, *, #79651, .T. ) ;
#39924=ORIENTED_EDGE ( 'NONE', *, *, #246509, .T. ) ;
#39928=DIRECTION ( 'NONE',  ( -1.000000000000000000, -0.000000000000000000, 0.000000000000000000 ) ) ;
#39932=CIRCLE ( 'NONE', #223070, 0.1000000000000028644 ) ;
#39945=ORIENTED_EDGE ( 'NONE', *, *, #237608, .F. ) ;
#39953=CARTESIAN_POINT ( 'NONE',  ( -23.15000000000000213, 0.000000000000000000, 0.000000000000000000 ) ) ;
#39966=EDGE_CURVE ( 'NONE', #183080, #197777, #69609, .T. ) ;
#40016=ORIENTED_EDGE ( 'NONE', *, *, #141502, .F. ) ;
#40028=ORIENTED_EDGE ( 'NONE', *, *, #225541, .F. ) ;
#40032=ORIENTED_EDGE ( 'NONE', *, *, #56466, .T. ) ;
#40035=CARTESIAN_POINT ( 'NONE',  ( 20.04142135623730070, 11.65000000000000391, -21.25000000000000000 ) ) ;
#40039=ORIENTED_EDGE ( 'NONE', *, *, #134276, .F. ) ;
#40063=ADVANCED_FACE ( 'NONE', ( #73479 ), #90758, .T. ) ;
#40095=AXIS2_PLACEMENT_3D ( 'NONE', #76454, #156027, #97267 ) ;
#40097=ORIENTED_EDGE ( 'NONE', *, *, #248130, .T. ) ;
#40134=ORIENTED_EDGE ( 'NONE', *, *, #198580, .F. ) ;
#40166=FACE_OUTER_BOUND ( 'NONE', #12324, .T. ) ;
#40180=ADVANCED_FACE ( 'NONE', ( #122856 ), #61587, .F. ) ;
#40208=EDGE_LOOP ( 'NONE', ( #190545, #122737, #246358, #90850 ) ) ;
#40215=ORIENTED_EDGE ( 'NONE', *, *, #118094, .F. ) ;
#40234=CIRCLE ( 'NONE', #73554, 0.09999999999999982514 ) ;
#40242=ORIENTED_EDGE ( 'NONE', *, *, #29714, .T. ) ;
#40343=CARTESIAN_POINT ( 'NONE',  ( 20.87631937322882791, 10.47149503676486226, -7.579745874581184317 ) ) ;
#40372=EDGE_CURVE ( 'NONE', #251836, #97348, #136736, .T. ) ;
#40384=ORIENTED_EDGE ( 'NONE', *, *, #130602, .T. ) ;
#40387=LINE ( 'NONE', #2481, #131210 ) ;
#40403=DIRECTION ( 'NONE',  ( 1.000000000000000000, -0.000000000000000000, -0.000000000000000000 ) ) ;
#40475=DIRECTION ( 'NONE',  ( 1.000000000000000000, -0.000000000000000000, 0.000000000000000000 ) ) ;
#40483=VERTEX_POINT ( 'NONE', #174860 ) ;
#40505=AXIS2_PLACEMENT_3D ( 'NONE', #61704, #220776, #160827 ) ;
#40532=CARTESIAN_POINT ( 'NONE',  ( 20.95568717954149562, 10.60199405389181848, -7.602508368268654060 ) ) ;
#40554=AXIS2_PLACEMENT_3D ( 'NONE', #148419, #54434, #34918 ) ;
#40564=ORIENTED_EDGE ( 'NONE', *, *, #113275, .T. ) ;
#40588=ORIENTED_EDGE ( 'NONE', *, *, #97645, .F. ) ;
#40610=LINE ( 'NONE', #157995, #81855 ) ;
#40642=ORIENTED_EDGE ( 'NONE', *, *, #242926, .F. ) ;
#40650=CARTESIAN_POINT ( 'NONE',  ( -21.05000000000000071, 5.900000000000005684, -23.28090023534362629 ) ) ;
#40669=CARTESIAN_POINT ( 'NONE',  ( 23.15000000000000213, -9.500000000000000000, -23.60603087734755690 ) ) ;
#40672=DIRECTION ( 'NONE',  ( 0.000000000000000000, 0.000000000000000000, -1.000000000000000000 ) ) ;
#40685=VERTEX_POINT ( 'NONE', #84645 ) ;
#40747=CARTESIAN_POINT ( 'NONE',  ( -18.50000000000000000, 9.150000000000002132, -12.34999999999999964 ) ) ;
#40786=CIRCLE ( 'NONE', #136379, 0.1000000000000028644 ) ;
#40797=CARTESIAN_POINT ( 'NONE',  ( 21.14999999999999858, 11.65000000000000746, -12.25000000000000000 ) ) ;
#40817=VERTEX_POINT ( 'NONE', #147228 ) ;
#40864=EDGE_LOOP ( 'NONE', ( #214713, #130037, #198658, #182820 ) ) ;
#40885=DIRECTION ( 'NONE',  ( -0.000000000000000000, 0.1298341882520022694, 0.9915357197604853789 ) ) ;
#40905=EDGE_LOOP ( 'NONE', ( #45967, #234576, #42753, #50948, #174946 ) ) ;
#40912=EDGE_CURVE ( 'NONE', #158624, #120448, #65770, .T. ) ;
#40918=FACE_OUTER_BOUND ( 'NONE', #252249, .T. ) ;
#40932=TOROIDAL_SURFACE ( 'NONE', #190952, 3.899999999999999467, 0.1000000000000000056 ) ;
#40966=AXIS2_PLACEMENT_3D ( 'NONE', #181613, #159479, #81190 ) ;
#40971=CIRCLE ( 'NONE', #136600, 0.1000000000000002554 ) ;
#41002=CARTESIAN_POINT ( 'NONE',  ( 20.94999999999999574, 11.62071067811865888, -26.63158334765902424 ) ) ;
#41007=DIRECTION ( 'NONE',  ( 0.000000000000000000, 0.000000000000000000, -1.000000000000000000 ) ) ;
#41016=ADVANCED_FACE ( 'NONE', ( #197899 ), #82175, .T. ) ;
#41026=CARTESIAN_POINT ( 'NONE',  ( -20.85000000000000142, -11.65000000000000036, -33.50000000000000000 ) ) ;
#41027=CARTESIAN_POINT ( 'NONE',  ( -22.39999999999999858, -0.1008583690987139431, 11.74956712348939192 ) ) ;
#41048=AXIS2_PLACEMENT_3D ( 'NONE', #222686, #239712, #97590 ) ;
#41058=ORIENTED_EDGE ( 'NONE', *, *, #183956, .F. ) ;
#41065=LINE ( 'NONE', #201387, #112057 ) ;
#41074=DIRECTION ( 'NONE',  ( -1.000000000000000000, -0.000000000000000000, 0.000000000000000000 ) ) ;
#41076=ORIENTED_EDGE ( 'NONE', *, *, #105558, .F. ) ;
#41086=CIRCLE ( 'NONE', #74417, 0.09999999999999961697 ) ;
#41087=AXIS2_PLACEMENT_3D ( 'NONE', #23920, #4309, #44748 ) ;
#41096=ORIENTED_EDGE ( 'NONE', *, *, #229460, .F. ) ;
#41116=DIRECTION ( 'NONE',  ( -1.000000000000000000, -1.836970198721029934E-16, 0.000000000000000000 ) ) ;
#41117=EDGE_CURVE ( 'NONE', #192810, #75563, #6108, .T. ) ;
#41118=CYLINDRICAL_SURFACE ( 'NONE', #251243, 0.1000000000000000611 ) ;
#41119=EDGE_CURVE ( 'NONE', #19733, #56467, #233000, .T. ) ;
#41161=EDGE_CURVE ( 'NONE', #226600, #107823, #245471, .T. ) ;
#41174=AXIS2_PLACEMENT_3D ( 'NONE', #189394, #26477, #49872 ) ;
#41201=VECTOR ( 'NONE', #152741, 1000.000000000000000 ) ;
#41213=EDGE_CURVE ( 'NONE', #52039, #169096, #132495, .T. ) ;
#41290=VECTOR ( 'NONE', #231704, 1000.000000000000000 ) ;
#41305=DIRECTION ( 'NONE',  ( 0.000000000000000000, 1.000000000000000000, 0.000000000000000000 ) ) ;
#41339=ORIENTED_EDGE ( 'NONE', *, *, #202106, .T. ) ;
#41358=ORIENTED_EDGE ( 'NONE', *, *, #143252, .T. ) ;
#41421=CARTESIAN_POINT ( 'NONE',  ( 21.05000000000000071, -1.249999999999999334, -7.900000000000000355 ) ) ;
#41434=CARTESIAN_POINT ( 'NONE',  ( -18.59999999999999787, 7.021664781900089913, -37.23356540189728747 ) ) ;
#41500=EDGE_CURVE ( 'NONE', #161077, #18698, #174961, .T. ) ;
#41522=ORIENTED_EDGE ( 'NONE', *, *, #3023, .T. ) ;
#41537=VERTEX_POINT ( 'NONE', #89207 ) ;
#41540=ORIENTED_EDGE ( 'NONE', *, *, #238538, .F. ) ;
#41591=CARTESIAN_POINT ( 'NONE',  ( -23.25000000000000000, 0.000000000000000000, -33.50000000000000000 ) ) ;
#41606=CARTESIAN_POINT ( 'NONE',  ( -18.50000000000000000, 11.64999999999999680, -21.35000000000000142 ) ) ;
#41612=ORIENTED_EDGE ( 'NONE', *, *, #203463, .F. ) ;
#41617=VERTEX_POINT ( 'NONE', #194434 ) ;
#41635=FACE_OUTER_BOUND ( 'NONE', #25836, .T. ) ;
#41638=DIRECTION ( 'NONE',  ( 1.000000000000000000, -0.000000000000000000, -0.000000000000000000 ) ) ;
#41645=DIRECTION ( 'NONE',  ( 1.000000000000000000, 2.952720810173289112E-16, -0.000000000000000000 ) ) ;
#41654=VERTEX_POINT ( 'NONE', #44334 ) ;
#41673=CARTESIAN_POINT ( 'NONE',  ( 18.59999999999999787, -1.835859311443637010, -45.00443916879852679 ) ) ;
#41703=CARTESIAN_POINT ( 'NONE',  ( 22.39999999999999503, 11.65000000000000746, -0.1000000000000028644 ) ) ;
#41718=ADVANCED_FACE ( 'NONE', ( #220404 ), #83091, .F. ) ;
#41735=ORIENTED_EDGE ( 'NONE', *, *, #18937, .T. ) ;
#41764=AXIS2_PLACEMENT_3D ( 'NONE', #83273, #22067, #181140 ) ;
#41765=ORIENTED_EDGE ( 'NONE', *, *, #61307, .T. ) ;
#41779=CARTESIAN_POINT ( 'NONE',  ( 23.24999999999999645, -2.100000000000002309, -33.50000000000000000 ) ) ;
#41783=DIRECTION ( 'NONE',  ( 1.000000000000000000, 0.000000000000000000, 0.000000000000000000 ) ) ;
#41792=DIRECTION ( 'NONE',  ( 1.000000000000000000, 0.000000000000000000, 0.000000000000000000 ) ) ;
#41801=CARTESIAN_POINT ( 'NONE',  ( 21.17356465864818560, 0.09891124101387020751, 6.422803126241725558 ) ) ;
#41835=EDGE_CURVE ( 'NONE', #3044, #92153, #230676, .T. ) ;
#41836=CIRCLE ( 'NONE', #241718, 0.1000000000000001305 ) ;
#41866=ORIENTED_EDGE ( 'NONE', *, *, #143162, .T. ) ;
#41871=DIRECTION ( 'NONE',  ( -1.000000000000000000, -0.000000000000000000, -0.000000000000000000 ) ) ;
#41897=AXIS2_PLACEMENT_3D ( 'NONE', #131508, #114516, #55784 ) ;
#41903=DIRECTION ( 'NONE',  ( 0.7071067811865388020, -0.7071067811865561215, 0.000000000000000000 ) ) ;
#41936=DIRECTION ( 'NONE',  ( 0.000000000000000000, 0.000000000000000000, -1.000000000000000000 ) ) ;
#41952=ADVANCED_FACE ( 'NONE', ( #235565 ), #173092, .T. ) ;
#41955=EDGE_CURVE ( 'NONE', #243771, #249368, #79202, .T. ) ;
#41973=ORIENTED_EDGE ( 'NONE', *, *, #200462, .F. ) ;
#41990=DIRECTION ( 'NONE',  ( -1.000000000000000000, 0.000000000000000000, 0.000000000000000000 ) ) ;
#42018=AXIS2_PLACEMENT_3D ( 'NONE', #216431, #135604, #172229 ) ;
#42021=LINE ( 'NONE', #202356, #184339 ) ;
#42059=CARTESIAN_POINT ( 'NONE',  ( -20.89192007715127986, 10.32898536000685574, -39.08266832227643306 ) ) ;
#42113=CARTESIAN_POINT ( 'NONE',  ( 18.59999999999999076, 10.20857864376269575, -21.25000000000000000 ) ) ;
#42120=B_SPLINE_CURVE_WITH_KNOTS ( 'NONE', 3,
 ( #258018, #222778, #102825, #162847, #104108, #182402 ),
 .UNSPECIFIED., .F., .F.,
 ( 4, 2, 4 ),
 ( 0.000000000000000000, 0.0001895189928937387276, 0.0003790379857874774552 ),
 .UNSPECIFIED. ) ;
#42148=CARTESIAN_POINT ( 'NONE',  ( -23.15000000000000213, 0.000000000000000000, 0.000000000000000000 ) ) ;
#42190=EDGE_CURVE ( 'NONE', #167418, #138366, #224402, .T. ) ;
#42203=CARTESIAN_POINT ( 'NONE',  ( 21.05000000000000071, 1.835341550224413698, -11.55515129256298401 ) ) ;
#42206=ORIENTED_EDGE ( 'NONE', *, *, #56353, .T. ) ;
#42237=FACE_OUTER_BOUND ( 'NONE', #222951, .T. ) ;
#42240=AXIS2_PLACEMENT_3D ( 'NONE', #125751, #5788, #227426 ) ;
#42250=EDGE_LOOP ( 'NONE', ( #180563, #80778, #232506, #232971, #196091 ) ) ;
#42276=EDGE_CURVE ( 'NONE', #49960, #213315, #103750, .T. ) ;
#42321=AXIS2_PLACEMENT_3D ( 'NONE', #53215, #31127, #248853 ) ;
#42325=CARTESIAN_POINT ( 'NONE',  ( -20.07928932188135107, 9.220710678118654968, -12.34999999999999964 ) ) ;
#42327=ORIENTED_EDGE ( 'NONE', *, *, #139074, .F. ) ;
#42356=LINE ( 'NONE', #120628, #142378 ) ;
#42366=CARTESIAN_POINT ( 'NONE',  ( 18.59117750673696179, 10.33248238082519066, -39.09484654391314962 ) ) ;
#42372=CARTESIAN_POINT ( 'NONE',  ( -23.25000000000000000, -11.65000000000000036, -30.50000000000000000 ) ) ;
#42390=ADVANCED_FACE ( 'NONE', ( #211875 ), #55309, .T. ) ;
#42398=EDGE_LOOP ( 'NONE', ( #230348, #55523, #2406 ) ) ;
#42399=CARTESIAN_POINT ( 'NONE',  ( -20.64999999999999858, 2.449293598294710359E-16, -35.50000000000000711 ) ) ;
#42424=AXIS2_PLACEMENT_3D ( 'NONE', #221794, #223097, #163150 ) ;
#42433=DIRECTION ( 'NONE',  ( -1.836970198721029934E-16, 1.000000000000000000, 0.000000000000000000 ) ) ;
#42439=DIRECTION ( 'NONE',  ( -0.000000000000000000, 0.1350103645451876666, 0.9908441862701600211 ) ) ;
#42445=ORIENTED_EDGE ( 'NONE', *, *, #146427, .F. ) ;
#42446=DIRECTION ( 'NONE',  ( 1.000000000000000000, 0.000000000000000000, 0.000000000000000000 ) ) ;
#42458=AXIS2_PLACEMENT_3D ( 'NONE', #183051, #66936, #185605 ) ;
#42470=DIRECTION ( 'NONE',  ( 0.000000000000000000, 0.000000000000000000, -1.000000000000000000 ) ) ;
#42504=ORIENTED_EDGE ( 'NONE', *, *, #187590, .T. ) ;
#42520=ORIENTED_EDGE ( 'NONE', *, *, #145840, .T. ) ;
#42528=CARTESIAN_POINT ( 'NONE',  ( 20.94999999999999574, -11.48912529307605901, -2.900000000000003464 ) ) ;
#42592=LINE ( 'NONE', #23058, #229285 ) ;
#42599=DIRECTION ( 'NONE',  ( 0.000000000000000000, 1.734723475976817507E-14, -1.000000000000000000 ) ) ;
#42605=CARTESIAN_POINT ( 'NONE',  ( -22.45354308602459525, 2.198771867883399074E-07, 11.75043289045890127 ) ) ;
#42616=CARTESIAN_POINT ( 'NONE',  ( -20.54999999999999716, 0.000000000000000000, 0.000000000000000000 ) ) ;
#42618=ORIENTED_EDGE ( 'NONE', *, *, #88156, .F. ) ;
#42643=CARTESIAN_POINT ( 'NONE',  ( 18.50000000000000000, -9.399999999999998579, -40.38204184817267617 ) ) ;
#42661=ADVANCED_FACE ( 'NONE', ( #78128 ), #232983, .F. ) ;
#42670=EDGE_CURVE ( 'NONE', #161077, #13860, #83072, .T. ) ;
#42723=AXIS2_PLACEMENT_3D ( 'NONE', #89616, #58179, #137721 ) ;
#42727=FACE_OUTER_BOUND ( 'NONE', #159331, .T. ) ;
#42745=TOROIDAL_SURFACE ( 'NONE', #34407, 0.2000000000000000111, 0.1000000000000000056 ) ;
#42748=CARTESIAN_POINT ( 'NONE',  ( 18.57071067811864040, 10.17928932188134539, -21.35000000000000142 ) ) ;
#42753=ORIENTED_EDGE ( 'NONE', *, *, #239243, .F. ) ;
#42768=DIRECTION ( 'NONE',  ( 0.000000000000000000, 0.000000000000000000, -1.000000000000000000 ) ) ;
#42868=DIRECTION ( 'NONE',  ( 1.000000000000000000, 0.000000000000000000, 0.000000000000000000 ) ) ;
#42877=ORIENTED_EDGE ( 'NONE', *, *, #183711, .F. ) ;
#42910=DIRECTION ( 'NONE',  ( 0.000000000000000000, -1.000000000000000000, 0.000000000000000000 ) ) ;
#42915=DIRECTION ( 'NONE',  ( 0.000000000000000000, 0.000000000000000000, -1.000000000000000000 ) ) ;
#42933=DIRECTION ( 'NONE',  ( 0.000000000000000000, 0.000000000000000000, -1.000000000000000000 ) ) ;
#42958=CARTESIAN_POINT ( 'NONE',  ( 22.39999999999999858, 7.790779598373385184, -1.572093150103981429E-15 ) ) ;
#42972=CIRCLE ( 'NONE', #117963, 0.5000000000000004441 ) ;
#43064=ORIENTED_EDGE ( 'NONE', *, *, #173494, .F. ) ;
#43079=ORIENTED_EDGE ( 'NONE', *, *, #123212, .F. ) ;
#43088=ORIENTED_EDGE ( 'NONE', *, *, #37960, .F. ) ;
#43111=AXIS2_PLACEMENT_3D ( 'NONE', #225606, #144798, #27486 ) ;
#43123=AXIS2_PLACEMENT_3D ( 'NONE', #198168, #61229, #258096 ) ;
#43135=EDGE_LOOP ( 'NONE', ( #65108, #70658, #28600, #80933 ) ) ;
#43136=ORIENTED_EDGE ( 'NONE', *, *, #103639, .T. ) ;
#43185=EDGE_LOOP ( 'NONE', ( #256082, #191656, #99835, #63835 ) ) ;
#43199=DIRECTION ( 'NONE',  ( 1.000000000000000000, 0.000000000000000000, 0.000000000000000000 ) ) ;
#43234=DIRECTION ( 'NONE',  ( 0.000000000000000000, 1.000000000000000000, 0.000000000000000000 ) ) ;
#43236=ORIENTED_EDGE ( 'NONE', *, *, #231159, .T. ) ;
#43239=CARTESIAN_POINT ( 'NONE',  ( -18.59999999999999787, 0.000000000000000000, -33.50000000000000000 ) ) ;
#43254=ORIENTED_EDGE ( 'NONE', *, *, #41119, .T. ) ;
#43271=DIRECTION ( 'NONE',  ( -0.000000000000000000, 0.1350103645451876666, 0.9908441862701600211 ) ) ;
#43421=VERTEX_POINT ( 'NONE', #174109 ) ;
#43462=FACE_OUTER_BOUND ( 'NONE', #128236, .T. ) ;
#43472=DIRECTION ( 'NONE',  ( 0.000000000000000000, 0.000000000000000000, 1.000000000000000000 ) ) ;
#43503=CARTESIAN_POINT ( 'NONE',  ( -20.54999999999999716, 4.349999999999999645, -21.25000000000000000 ) ) ;
#43512=CARTESIAN_POINT ( 'NONE',  ( -18.50000000000000000, 10.29288807858820398, -38.95800201601218049 ) ) ;
#43513=DIRECTION ( 'NONE',  ( -0.000000000000000000, 0.000000000000000000, -1.000000000000000000 ) ) ;
#43525=CARTESIAN_POINT ( 'NONE',  ( -21.05000000000000071, 11.74999999999999645, -26.65839931010294706 ) ) ;
#43532=ADVANCED_FACE ( 'NONE', ( #180486 ), #21434, .T. ) ;
#43560=DIRECTION ( 'NONE',  ( -0.000000000000000000, 0.8660254037844383745, -0.5000000000000003331 ) ) ;
#43612=CIRCLE ( 'NONE', #210221, 0.5999999999999998668 ) ;
#43628=DIRECTION ( 'NONE',  ( -0.000000000000000000, 0.000000000000000000, -1.000000000000000000 ) ) ;
#43641=ADVANCED_FACE ( 'NONE', ( #222141 ), #269, .T. ) ;
#43646=DIRECTION ( 'NONE',  ( -0.000000000000000000, 0.1298341882520022694, 0.9915357197604853789 ) ) ;
#43648=AXIS2_PLACEMENT_3D ( 'NONE', #59651, #135355, #94948 ) ;
#43672=ORIENTED_EDGE ( 'NONE', *, *, #245097, .F. ) ;
#43680=DIRECTION ( 'NONE',  ( 1.000000000000000000, -0.000000000000000000, -0.000000000000000000 ) ) ;
#43727=EDGE_LOOP ( 'NONE', ( #179125, #122680, #218202, #132660 ) ) ;
#43735=DIRECTION ( 'NONE',  ( 0.000000000000000000, 0.000000000000000000, 1.000000000000000000 ) ) ;
#43803=DIRECTION ( 'NONE',  ( 1.000000000000000000, -0.000000000000000000, -0.000000000000000000 ) ) ;
#43814=EDGE_CURVE ( 'NONE', #191967, #116906, #83627, .T. ) ;
#43835=ORIENTED_EDGE ( 'NONE', *, *, #221673, .T. ) ;
#43842=DIRECTION ( 'NONE',  ( 1.000000000000000000, -0.000000000000000000, -0.000000000000000000 ) ) ;
#43846=CARTESIAN_POINT ( 'NONE',  ( -23.25000000000000000, -9.600000000000001421, -23.60603087734756045 ) ) ;
#43854=VERTEX_POINT ( 'NONE', #139741 ) ;
#43866=ORIENTED_EDGE ( 'NONE', *, *, #62086, .T. ) ;
#43921=CARTESIAN_POINT ( 'NONE',  ( -18.40000000000000213, -9.519327731092442235, -6.972976376559327782 ) ) ;
#43937=ORIENTED_EDGE ( 'NONE', *, *, #55379, .T. ) ;
#43957=CARTESIAN_POINT ( 'NONE',  ( -20.94999999999999929, 1.835341550224413698, -11.55515129256298046 ) ) ;
#43982=DIRECTION ( 'NONE',  ( 0.000000000000000000, -0.8660254037844412611, -0.4999999999999956701 ) ) ;
#43998=CARTESIAN_POINT ( 'NONE',  ( -20.97625342178427132, 11.60000000082050953, -6.928203229801833452 ) ) ;
#43999=EDGE_CURVE ( 'NONE', #113100, #52139, #123726, .T. ) ;
#44001=AXIS2_PLACEMENT_3D ( 'NONE', #102995, #182572, #85982 ) ;
#44002=DIRECTION ( 'NONE',  ( 1.000000000000000000, 0.000000000000000000, 0.000000000000000000 ) ) ;
#44031=CARTESIAN_POINT ( 'NONE',  ( 18.59999999999999432, 1.162701749938009677, -8.099999999999999645 ) ) ;
#44035=DIRECTION ( 'NONE',  ( 0.7071067811865388020, -0.7071067811865561215, 0.000000000000000000 ) ) ;
#44052=CARTESIAN_POINT ( 'NONE',  ( 21.05000000000000071, -9.400000000000002132, -9.893969122652443104 ) ) ;
#44075=DIRECTION ( 'NONE',  ( -1.000000000000000000, 0.000000000000000000, 0.000000000000000000 ) ) ;
#44087=CARTESIAN_POINT ( 'NONE',  ( -21.53699400380413564, 6.787711793193499155, -1.424708524881391155E-14 ) ) ;
#44105=EDGE_LOOP ( 'NONE', ( #154387, #146732, #3000, #213187, #3996 ) ) ;
#44138=EDGE_CURVE ( 'NONE', #169096, #160332, #13132, .T. ) ;
#44195=CARTESIAN_POINT ( 'NONE',  ( -18.59999999999999787, -1.866714910057309273, -11.75267524628200633 ) ) ;
#44201=VERTEX_POINT ( 'NONE', #175717 ) ;
#44212=AXIS2_PLACEMENT_3D ( 'NONE', #162809, #64962, #238473 ) ;
#44231=DIRECTION ( 'NONE',  ( 0.000000000000000000, 8.023096076392503095E-14, 1.000000000000000000 ) ) ;
#44251=DIRECTION ( 'NONE',  ( 0.000000000000000000, 0.000000000000000000, -1.000000000000000000 ) ) ;
#44257=CIRCLE ( 'NONE', #85904, 0.09999999999999954758 ) ;
#44275=EDGE_CURVE ( 'NONE', #207698, #13242, #100572, .T. ) ;
#44297=ORIENTED_EDGE ( 'NONE', *, *, #92333, .F. ) ;
#44319=VERTEX_POINT ( 'NONE', #145538 ) ;
#44327=DIRECTION ( 'NONE',  ( -0.000000000000000000, 0.000000000000000000, -1.000000000000000000 ) ) ;
#44329=DIRECTION ( 'NONE',  ( -1.000000000000000000, 0.000000000000000000, 0.000000000000000000 ) ) ;
#44334=CARTESIAN_POINT ( 'NONE',  ( 18.39999999999999858, -9.600000000000003197, -40.20018939122204671 ) ) ;
#44350=EDGE_CURVE ( 'NONE', #24982, #156671, #26918, .T. ) ;
#44366=AXIS2_PLACEMENT_3D ( 'NONE', #42528, #162506, #85472 ) ;
#44399=VECTOR ( 'NONE', #241934, 1000.000000000000000 ) ;
#44417=ORIENTED_EDGE ( 'NONE', *, *, #130630, .T. ) ;
#44433=ORIENTED_EDGE ( 'NONE', *, *, #254102, .T. ) ;
#44445=EDGE_CURVE ( 'NONE', #256245, #212201, #213024, .T. ) ;
#44473=DIRECTION ( 'NONE',  ( 0.000000000000000000, 0.000000000000000000, 1.000000000000000000 ) ) ;
#44474=CARTESIAN_POINT ( 'NONE',  ( 21.14999999999999858, 6.540656951701244282, 0.000000000000000000 ) ) ;
#44491=ADVANCED_FACE ( 'NONE', ( #50281 ), #160685, .F. ) ;
#44513=CARTESIAN_POINT ( 'NONE',  ( -18.59999999999999787, 11.64999999999999680, -21.35000000000000142 ) ) ;
#44539=AXIS2_PLACEMENT_3D ( 'NONE', #52427, #248074, #9461 ) ;
#44549=CARTESIAN_POINT ( 'NONE',  ( 23.14999999999999858, 0.000000000000000000, -35.50000000000000711 ) ) ;
#44577=FACE_OUTER_BOUND ( 'NONE', #175414, .T. ) ;
#44599=CARTESIAN_POINT ( 'NONE',  ( -20.94999999999999929, 1.261786168565025568, -8.086498963545480478 ) ) ;
#44611=DIRECTION ( 'NONE',  ( 1.000000000000000000, -0.000000000000000000, -0.000000000000000000 ) ) ;
#44657=VECTOR ( 'NONE', #53746, 1000.000000000000000 ) ;
#44702=TOROIDAL_SURFACE ( 'NONE', #3157, 0.2000000000000000111, 0.1000000000000000056 ) ;
#44715=VERTEX_POINT ( 'NONE', #159684 ) ;
#44748=DIRECTION ( 'NONE',  ( 0.000000000000000000, 0.000000000000000000, -1.000000000000000000 ) ) ;
#44802=DIRECTION ( 'NONE',  ( 0.000000000000000000, 0.000000000000000000, -1.000000000000000000 ) ) ;
#44809=VERTEX_POINT ( 'NONE', #29204 ) ;
#44826=CARTESIAN_POINT ( 'NONE',  ( -23.15000000000000213, 4.250000000000000000, -12.35000000000000142 ) ) ;
#44834=AXIS2_PLACEMENT_3D ( 'NONE', #64554, #144075, #5848 ) ;
#44852=VECTOR ( 'NONE', #61939, 1000.000000000000000 ) ;
#44860=CYLINDRICAL_SURFACE ( 'NONE', #233539, 0.09999999999999939493 ) ;
#44873=ADVANCED_FACE ( 'NONE', ( #185660 ), #146508, .F. ) ;
#44876=FACE_OUTER_BOUND ( 'NONE', #218190, .T. ) ;
#44877=AXIS2_PLACEMENT_3D ( 'NONE', #204578, #89762, #169357 ) ;
#44940=ORIENTED_EDGE ( 'NONE', *, *, #210132, .T. ) ;
#44986=CARTESIAN_POINT ( 'NONE',  ( -20.07928932188135107, 9.220710678118654968, -21.25000000000000000 ) ) ;
#44994=ORIENTED_EDGE ( 'NONE', *, *, #87991, .F. ) ;
#45002=DIRECTION ( 'NONE',  ( 0.000000000000000000, 0.000000000000000000, -1.000000000000000000 ) ) ;
#45005=CARTESIAN_POINT ( 'NONE',  ( -23.25000000000000000, -1.835859311443637010, -45.10443916879852821 ) ) ;
#45018=ORIENTED_EDGE ( 'NONE', *, *, #111677, .T. ) ;
#45020=ORIENTED_EDGE ( 'NONE', *, *, #141113, .F. ) ;
#45042=FACE_OUTER_BOUND ( 'NONE', #17827, .T. ) ;
#45091=AXIS2_PLACEMENT_3D ( 'NONE', #31751, #13446, #111259 ) ;
#45131=CARTESIAN_POINT ( 'NONE',  ( 20.94999999999999574, 8.926614585087095932, -8.471683019223121391 ) ) ;
#45136=DIRECTION ( 'NONE',  ( 0.000000000000000000, 0.000000000000000000, -1.000000000000000000 ) ) ;
#45160=CARTESIAN_POINT ( 'NONE',  ( -23.15000000000000213, -9.600000000000004974, -9.893969122652444881 ) ) ;
#45167=CARTESIAN_POINT ( 'NONE',  ( -21.05000000000000071, 11.75000000000000000, -26.48519422934605316 ) ) ;
#45173=CARTESIAN_POINT ( 'NONE',  ( -18.50000000000000000, -1.362429037193310988, -41.38888124792119783 ) ) ;
#45180=CARTESIAN_POINT ( 'NONE',  ( 22.50000000000000000, 11.64957080754479968, 0.09999999999999592548 ) ) ;
#45203=FACE_OUTER_BOUND ( 'NONE', #117382, .T. ) ;
#45223=CIRCLE ( 'NONE', #124346, 0.09999999999999939493 ) ;
#45251=ORIENTED_EDGE ( 'NONE', *, *, #242449, .F. ) ;
#45254=CARTESIAN_POINT ( 'NONE',  ( 23.14999999999999147, 4.149999999999999467, 5.082284216461513184E-16 ) ) ;
#45262=EDGE_CURVE ( 'NONE', #212201, #245427, #177232, .T. ) ;
#45344=VERTEX_POINT ( 'NONE', #24569 ) ;
#45378=EDGE_LOOP ( 'NONE', ( #50482, #230467, #127917, #197788 ) ) ;
#45380=FACE_OUTER_BOUND ( 'NONE', #97727, .T. ) ;
#45398=CIRCLE ( 'NONE', #141084, 0.09999999999999939493 ) ;
#45414=AXIS2_PLACEMENT_3D ( 'NONE', #168079, #106760, #243719 ) ;
#45462=LINE ( 'NONE', #125014, #133493 ) ;
#45468=VECTOR ( 'NONE', #8240, 1000.000000000000000 ) ;
#45491=CARTESIAN_POINT ( 'NONE',  ( 22.39999999999999503, 11.75000000000000000, -3.469446951953614189E-15 ) ) ;
#45500=DIRECTION ( 'NONE',  ( 0.000000000000000000, 0.000000000000000000, -1.000000000000000000 ) ) ;
#45521=AXIS2_PLACEMENT_3D ( 'NONE', #85583, #106441, #167760 ) ;
#45524=DIRECTION ( 'NONE',  ( -1.000000000000000000, -0.000000000000000000, 0.000000000000000000 ) ) ;
#45543=AXIS2_PLACEMENT_3D ( 'NONE', #11814, #59867, #239829 ) ;
#45544=ADVANCED_FACE ( 'NONE', ( #127498 ), #207038, .T. ) ;
#45576=EDGE_CURVE ( 'NONE', #243852, #109777, #205182, .T. ) ;
#45617=ORIENTED_EDGE ( 'NONE', *, *, #128956, .T. ) ;
#45631=CARTESIAN_POINT ( 'NONE',  ( -22.50014994444008209, 11.74971973189209606, 0.08308015671916883782 ) ) ;
#45657=ORIENTED_EDGE ( 'NONE', *, *, #193558, .F. ) ;
#45675=FACE_OUTER_BOUND ( 'NONE', #202802, .T. ) ;
#45690=CARTESIAN_POINT ( 'NONE',  ( -20.54999999999999716, 9.350000000000001421, -21.25000000000000000 ) ) ;
#45691=LINE ( 'NONE', #103075, #247524 ) ;
#45708=CARTESIAN_POINT ( 'NONE',  ( -20.64999999999999858, -9.500000000000003553, -9.893969122652444881 ) ) ;
#45719=DIRECTION ( 'NONE',  ( -1.000000000000000000, -0.000000000000000000, -0.000000000000000000 ) ) ;
#45753=LINE ( 'NONE', #40669, #37192 ) ;
#45770=AXIS2_PLACEMENT_3D ( 'NONE', #103226, #26289, #108390 ) ;
#45812=EDGE_CURVE ( 'NONE', #225666, #107696, #57977, .T. ) ;
#45814=ORIENTED_EDGE ( 'NONE', *, *, #153372, .T. ) ;
#45820=FACE_OUTER_BOUND ( 'NONE', #176904, .T. ) ;
#45832=VERTEX_POINT ( 'NONE', #218332 ) ;
#45838=ORIENTED_EDGE ( 'NONE', *, *, #19256, .T. ) ;
#45862=CARTESIAN_POINT ( 'NONE',  ( -21.05000000000000071, -1.835341550224411922, -11.55515129256297868 ) ) ;
#45890=EDGE_CURVE ( 'NONE', #143742, #206232, #72126, .T. ) ;
#45917=EDGE_CURVE ( 'NONE', #192810, #122573, #255403, .T. ) ;
#45938=EDGE_CURVE ( 'NONE', #185736, #242879, #30431, .T. ) ;
#45967=ORIENTED_EDGE ( 'NONE', *, *, #82177, .T. ) ;
#45977=DIRECTION ( 'NONE',  ( 1.000000000000000000, -0.000000000000000000, -0.000000000000000000 ) ) ;
#45991=DIRECTION ( 'NONE',  ( 0.000000000000000000, 0.000000000000000000, -1.000000000000000000 ) ) ;
#46002=VECTOR ( 'NONE', #244942, 1000.000000000000000 ) ;
#46052=DIRECTION ( 'NONE',  ( 0.000000000000000000, 0.000000000000000000, -1.000000000000000000 ) ) ;
#46090=CARTESIAN_POINT ( 'NONE',  ( 20.87155475150661132, 11.75000000000000355, -26.59558652915735522 ) ) ;
#46120=AXIS2_PLACEMENT_3D ( 'NONE', #196585, #17946, #177059 ) ;
#46156=VECTOR ( 'NONE', #157421, 1000.000000000000000 ) ;
#46165=CARTESIAN_POINT ( 'NONE',  ( 22.45305468355010348, -0.1008583690997046090, 11.74956712348972587 ) ) ;
#46168=ORIENTED_EDGE ( 'NONE', *, *, #92327, .T. ) ;
#46177=EDGE_LOOP ( 'NONE', ( #247976, #159391, #101618, #71749 ) ) ;
#46202=CIRCLE ( 'NONE', #33612, 0.1000000000000028644 ) ;
#46251=CIRCLE ( 'NONE', #137833, 11.75000000000000000 ) ;
#46268=SPHERICAL_SURFACE ( 'NONE', #25502, 0.1000000000000000056 ) ;
#46296=ADVANCED_FACE ( 'NONE', ( #10249 ), #250136, .T. ) ;
#46302=AXIS2_PLACEMENT_3D ( 'NONE', #159055, #40403, #80750 ) ;
#46323=ORIENTED_EDGE ( 'NONE', *, *, #128385, .F. ) ;
#46380=PLANE ( 'NONE',  #112834 ) ;
#46388=DIRECTION ( 'NONE',  ( 1.000000000000000000, 7.304098846218135653E-16, 0.000000000000000000 ) ) ;
#46410=ORIENTED_EDGE ( 'NONE', *, *, #157521, .F. ) ;
#46414=DIRECTION ( 'NONE',  ( 0.000000000000000000, 0.000000000000000000, -1.000000000000000000 ) ) ;
#46445=CARTESIAN_POINT ( 'NONE',  ( -21.05000000000000071, -0.09999999999999939493, 11.64957080754479968 ) ) ;
#46471=CARTESIAN_POINT ( 'NONE',  ( -18.40000000000000213, -9.500000000000007105, -7.032069396699661468 ) ) ;
#46519=DIRECTION ( 'NONE',  ( -0.7071067811865474617, -0.7071067811865474617, -0.000000000000000000 ) ) ;
#46524=PLANE ( 'NONE',  #104023 ) ;
#46540=ORIENTED_EDGE ( 'NONE', *, *, #86973, .T. ) ;
#46545=CARTESIAN_POINT ( 'NONE',  ( -23.15000000000000213, 4.349999999999999645, -12.35000000000000142 ) ) ;
#46554=ADVANCED_FACE ( 'NONE', ( #126009 ), #103863, .F. ) ;
#46595=ORIENTED_EDGE ( 'NONE', *, *, #192635, .T. ) ;
#46604=DIRECTION ( 'NONE',  ( 1.000000000000000000, 0.000000000000000000, 0.000000000000000000 ) ) ;
#46642=ORIENTED_EDGE ( 'NONE', *, *, #57104, .T. ) ;
#46682=FACE_OUTER_BOUND ( 'NONE', #129381, .T. ) ;
#46691=EDGE_LOOP ( 'NONE', ( #134503, #198780, #223081 ) ) ;
#46693=ORIENTED_EDGE ( 'NONE', *, *, #187147, .T. ) ;
#46729=CARTESIAN_POINT ( 'NONE',  ( 20.94999999999999929, 6.450000000000001066, -10.01702717044001822 ) ) ;
#46745=CARTESIAN_POINT ( 'NONE',  ( 23.14999999999999503, 6.550000000000000711, -12.35000000000000320 ) ) ;
#46757=DIRECTION ( 'NONE',  ( 0.000000000000000000, 0.4999999999999966693, -0.8660254037844405950 ) ) ;
#46762=ORIENTED_EDGE ( 'NONE', *, *, #246509, .F. ) ;
#46793=EDGE_LOOP ( 'NONE', ( #234619, #203746, #16300, #27935 ) ) ;
#46807=CIRCLE ( 'NONE', #67672, 11.75000000000000000 ) ;
#46810=EDGE_LOOP ( 'NONE', ( #1386, #104350, #80862, #250026 ) ) ;
#46818=CYLINDRICAL_SURFACE ( 'NONE', #12662, 0.09999999999999892308 ) ;
#46829=EDGE_LOOP ( 'NONE', ( #75098, #55327, #43866, #201098 ) ) ;
#46840=CIRCLE ( 'NONE', #113495, 0.09999999999999939493 ) ;
#46868=LINE ( 'NONE', #205958, #118312 ) ;
#46872=CIRCLE ( 'NONE', #105108, 0.1000000000000003803 ) ;
#46910=ORIENTED_EDGE ( 'NONE', *, *, #236469, .F. ) ;
#46920=EDGE_CURVE ( 'NONE', #110550, #72537, #205936, .T. ) ;
#46926=CARTESIAN_POINT ( 'NONE',  ( -20.94999999999999929, -1.135018845910178431, -41.21697688343231647 ) ) ;
#46942=CIRCLE ( 'NONE', #159411, 0.2000000000000005107 ) ;
#46976=CARTESIAN_POINT ( 'NONE',  ( -20.15000000000000568, 9.291421356237307805, -12.25000000000000000 ) ) ;
#46997=AXIS2_PLACEMENT_3D ( 'NONE', #246776, #88978, #225905 ) ;
#47000=CARTESIAN_POINT ( 'NONE',  ( -20.94999999999999929, 11.64999999999999680, -33.50000000000000000 ) ) ;
#47018=ORIENTED_EDGE ( 'NONE', *, *, #58403, .F. ) ;
#47043=CIRCLE ( 'NONE', #134518, 1.900000000000005906 ) ;
#47056=DIRECTION ( 'NONE',  ( 0.000000000000000000, 0.000000000000000000, -1.000000000000000000 ) ) ;
#47066=VERTEX_POINT ( 'NONE', #227384 ) ;
#47102=DIRECTION ( 'NONE',  ( -1.000000000000000000, -0.000000000000000000, -0.000000000000000000 ) ) ;
#47156=VERTEX_POINT ( 'NONE', #209107 ) ;
#47184=EDGE_CURVE ( 'NONE', #211780, #217631, #50911, .T. ) ;
#47195=DIRECTION ( 'NONE',  ( 0.000000000000000000, 0.000000000000000000, -1.000000000000000000 ) ) ;
#47239=SPHERICAL_SURFACE ( 'NONE', #126502, 0.1000000000000000056 ) ;
#47334=CARTESIAN_POINT ( 'NONE',  ( -18.59999999999999787, 11.74999999999999645, -12.15000000000000036 ) ) ;
#47340=CARTESIAN_POINT ( 'NONE',  ( -20.15000000000000568, 9.291421356237307805, -21.15000000000000213 ) ) ;
#47350=VERTEX_POINT ( 'NONE', #84973 ) ;
#47377=TOROIDAL_SURFACE ( 'NONE', #126688, 0.2000000000000000111, 0.1000000000000000056 ) ;
#47381=ORIENTED_EDGE ( 'NONE', *, *, #107381, .T. ) ;
#47439=ORIENTED_EDGE ( 'NONE', *, *, #44350, .T. ) ;
#47450=CARTESIAN_POINT ( 'NONE',  ( 23.14999999999999503, 14.05000000000000071, -27.98630492923908619 ) ) ;
#47455=DIRECTION ( 'NONE',  ( -1.000000000000000000, -3.265361837132813093E-16, 0.000000000000000000 ) ) ;
#47483=CARTESIAN_POINT ( 'NONE',  ( 18.51024323315077069, 10.31104185822948338, -39.02045169831058757 ) ) ;
#47518=EDGE_CURVE ( 'NONE', #110550, #34172, #176124, .T. ) ;
#47584=CARTESIAN_POINT ( 'NONE',  ( 18.59999999999999432, -1.162701749938009677, -8.099999999999999645 ) ) ;
#47590=EDGE_LOOP ( 'NONE', ( #33238, #39799, #79673, #195884 ) ) ;
#47591=CARTESIAN_POINT ( 'NONE',  ( 20.94999999999999929, 0.000000000000000000, -33.50000000000000000 ) ) ;
#47604=FACE_OUTER_BOUND ( 'NONE', #173037, .T. ) ;
#47607=DIRECTION ( 'NONE',  ( 0.000000000000000000, -0.1495327102803689356, -0.9887567792719336168 ) ) ;
#47659=CIRCLE ( 'NONE', #168359, 0.09999999999999939493 ) ;
#47677=AXIS2_PLACEMENT_3D ( 'NONE', #161659, #2543, #20867 ) ;
#47679=AXIS2_PLACEMENT_3D ( 'NONE', #225957, #223410, #86450 ) ;
#47684=AXIS2_PLACEMENT_3D ( 'NONE', #192455, #230284, #109050 ) ;
#47692=VECTOR ( 'NONE', #146957, 1000.000000000000000 ) ;
#47752=CARTESIAN_POINT ( 'NONE',  ( -18.43599941264911024, -9.519327428594779761, -6.972976789521343477 ) ) ;
#47778=ADVANCED_FACE ( 'NONE', ( #8679 ), #88182, .T. ) ;
#47828=CARTESIAN_POINT ( 'NONE',  ( 20.94999999999999929, 1.835341550224413698, -11.55515129256298401 ) ) ;
#47835=CARTESIAN_POINT ( 'NONE',  ( 23.15000000000000213, -11.74999999999999289, -12.25000000000000000 ) ) ;
#47849=ADVANCED_FACE ( 'NONE', ( #191197 ), #155874, .F. ) ;
#47864=ORIENTED_EDGE ( 'NONE', *, *, #10553, .T. ) ;
#47946=ORIENTED_EDGE ( 'NONE', *, *, #175147, .F. ) ;
#47964=SPHERICAL_SURFACE ( 'NONE', #234401, 0.1000000000000000056 ) ;
#47980=VERTEX_POINT ( 'NONE', #56752 ) ;
#47999=CARTESIAN_POINT ( 'NONE',  ( -23.25000000000000000, 11.75000000000000000, -33.50000000000000000 ) ) ;
#48067=CARTESIAN_POINT ( 'NONE',  ( 18.59999999999998366, 0.000000000000000000, -33.50000000000000000 ) ) ;
#48071=ORIENTED_EDGE ( 'NONE', *, *, #148886, .T. ) ;
#48135=EDGE_CURVE ( 'NONE', #68538, #257538, #150186, .T. ) ;
#48151=ORIENTED_EDGE ( 'NONE', *, *, #109051, .T. ) ;
#48176=AXIS2_PLACEMENT_3D ( 'NONE', #49055, #208159, #165162 ) ;
#48182=DIRECTION ( 'NONE',  ( -1.000000000000000000, 0.000000000000000000, 0.000000000000000000 ) ) ;
#48192=AXIS2_PLACEMENT_3D ( 'NONE', #80406, #196537, #177017 ) ;
#48206=AXIS2_PLACEMENT_3D ( 'NONE', #50378, #209480, #188630 ) ;
#48213=ADVANCED_FACE ( 'NONE', ( #50069 ), #112622, .F. ) ;
#48216=CARTESIAN_POINT ( 'NONE',  ( -21.78635804494510708, 7.035661485153180017, 0.09900506550767837477 ) ) ;
#48231=DIRECTION ( 'NONE',  ( 1.000000000000000000, -0.000000000000000000, -0.000000000000000000 ) ) ;
#48232=CIRCLE ( 'NONE', #202177, 0.1000000000000002554 ) ;
#48246=VECTOR ( 'NONE', #60003, 1000.000000000000114 ) ;
#48253=ORIENTED_EDGE ( 'NONE', *, *, #157233, .F. ) ;
#48260=ORIENTED_EDGE ( 'NONE', *, *, #20543, .F. ) ;
#48263=AXIS2_PLACEMENT_3D ( 'NONE', #28864, #91366, #69242 ) ;
#48268=ORIENTED_EDGE ( 'NONE', *, *, #187071, .F. ) ;
#48304=LINE ( 'NONE', #106983, #149366 ) ;
#48317=DIRECTION ( 'NONE',  ( 0.000000000000000000, 0.000000000000000000, -1.000000000000000000 ) ) ;
#48327=CARTESIAN_POINT ( 'NONE',  ( -21.05000000000000071, 6.478078221094754063, -0.09999993530616047011 ) ) ;
#48341=CIRCLE ( 'NONE', #2532, 0.09999999999999939493 ) ;
#48344=AXIS2_PLACEMENT_3D ( 'NONE', #117635, #197159, #214171 ) ;
#48377=ORIENTED_EDGE ( 'NONE', *, *, #35575, .F. ) ;
#48391=DIRECTION ( 'NONE',  ( -1.000000000000000000, -2.952720810173289112E-16, 0.000000000000000000 ) ) ;
#48393=DIRECTION ( 'NONE',  ( 1.000000000000000000, -0.000000000000000000, -0.000000000000000000 ) ) ;
#48404=EDGE_LOOP ( 'NONE', ( #187178, #4481, #210988, #114795 ) ) ;
#48465=AXIS2_PLACEMENT_3D ( 'NONE', #249326, #150225, #229742 ) ;
#48486=CARTESIAN_POINT ( 'NONE',  ( -20.94999999999999929, -11.64999999999999858, -3.100000000000001865 ) ) ;
#48498=ORIENTED_EDGE ( 'NONE', *, *, #23685, .T. ) ;
#48513=CIRCLE ( 'NONE', #194307, 0.4000000000000010214 ) ;
#48551=CARTESIAN_POINT ( 'NONE',  ( -21.05000000000000071, -1.249999999999999334, -8.000000000000000000 ) ) ;
#48573=ADVANCED_FACE ( 'NONE', ( #247961 ), #52317, .F. ) ;
#48639=CARTESIAN_POINT ( 'NONE',  ( 18.59999999999999076, 6.450000000000001066, -10.01702717044001822 ) ) ;
#48673=LINE ( 'NONE', #89085, #206375 ) ;
#48677=CARTESIAN_POINT ( 'NONE',  ( 18.52928932188133970, 10.27928932188134858, -21.35000000000000142 ) ) ;
#48686=CIRCLE ( 'NONE', #61178, 4.049999999999998934 ) ;
#48724=ADVANCED_FACE ( 'NONE', ( #193149 ), #15233, .T. ) ;
#48742=DIRECTION ( 'NONE',  ( 1.000000000000000000, 2.952720810173289112E-16, -0.000000000000000000 ) ) ;
#48756=FACE_OUTER_BOUND ( 'NONE', #256415, .T. ) ;
#48813=ORIENTED_EDGE ( 'NONE', *, *, #126569, .T. ) ;
#48822=EDGE_CURVE ( 'NONE', #217631, #239696, #2734, .T. ) ;
#48900=AXIS2_PLACEMENT_3D ( 'NONE', #116486, #60343, #199888 ) ;
#48912=ORIENTED_EDGE ( 'NONE', *, *, #113325, .F. ) ;
#48920=CIRCLE ( 'NONE', #107187, 0.6000000000000015321 ) ;
#48921=CARTESIAN_POINT ( 'NONE',  ( -21.05000000000000071, -1.835341550224411922, -11.55515129256297868 ) ) ;
#48926=EDGE_CURVE ( 'NONE', #106103, #250767, #202657, .T. ) ;
#48946=CARTESIAN_POINT ( 'NONE',  ( 20.94999999999999929, 11.65000000000000391, -26.71613433702190932 ) ) ;
#48960=CARTESIAN_POINT ( 'NONE',  ( -23.15000000000000213, 4.349999999999999645, -21.14999999999999858 ) ) ;
#48968=DIRECTION ( 'NONE',  ( -1.836970198721029934E-16, 1.000000000000000000, 0.000000000000000000 ) ) ;
#48982=AXIS2_PLACEMENT_3D ( 'NONE', #170867, #208672, #250343 ) ;
#49003=CARTESIAN_POINT ( 'NONE',  ( 20.91682497891422798, 10.32263460346243633, -39.06059579686719019 ) ) ;
#49039=ADVANCED_FACE ( 'NONE', ( #27381 ), #187716, .T. ) ;
#49042=ORIENTED_EDGE ( 'NONE', *, *, #223329, .T. ) ;
#49055=CARTESIAN_POINT ( 'NONE',  ( -23.15000000000000213, -11.65000000000000036, -30.39999999999999503 ) ) ;
#49062=CARTESIAN_POINT ( 'NONE',  ( -20.54999999999999716, 0.000000000000000000, 0.000000000000000000 ) ) ;
#49074=EDGE_CURVE ( 'NONE', #77408, #194720, #157066, .T. ) ;
#49099=VERTEX_POINT ( 'NONE', #66010 ) ;
#49128=ORIENTED_EDGE ( 'NONE', *, *, #61506, .T. ) ;
#49153=CIRCLE ( 'NONE', #228243, 4.300000000000032685 ) ;
#49158=VERTEX_POINT ( 'NONE', #168698 ) ;
#49181=DIRECTION ( 'NONE',  ( -1.000000000000000000, -7.304098846218134667E-16, 0.000000000000000000 ) ) ;
#49198=DIRECTION ( 'NONE',  ( 0.000000000000000000, -0.4791956752371546169, -0.8777080977375152360 ) ) ;
#49205=TOROIDAL_SURFACE ( 'NONE', #41048, 0.2000000000000000111, 0.1000000000000000056 ) ;
#49214=ORIENTED_EDGE ( 'NONE', *, *, #142696, .T. ) ;
#49215=DIRECTION ( 'NONE',  ( -1.000000000000000000, -0.000000000000000000, -0.000000000000000000 ) ) ;
#49248=CARTESIAN_POINT ( 'NONE',  ( 22.39999999999999503, 11.65000000000000746, 0.09999999999999592548 ) ) ;
#49320=VECTOR ( 'NONE', #69257, 1000.000000000000000 ) ;
#49334=EDGE_CURVE ( 'NONE', #224010, #56398, #92952, .T. ) ;
#49348=EDGE_CURVE ( 'NONE', #117400, #130735, #73427, .T. ) ;
#49353=DIRECTION ( 'NONE',  ( -0.000000000000000000, -0.000000000000000000, 1.000000000000000000 ) ) ;
#49356=DIRECTION ( 'NONE',  ( 0.000000000000000000, 0.000000000000000000, 1.000000000000000000 ) ) ;
#49368=CARTESIAN_POINT ( 'NONE',  ( 22.39999999999999503, 11.75000000000000711, -0.1000000000000028644 ) ) ;
#49375=AXIS2_PLACEMENT_3D ( 'NONE', #228573, #167331, #246829 ) ;
#49387=DIRECTION ( 'NONE',  ( 0.000000000000000000, 0.000000000000000000, 1.000000000000000000 ) ) ;
#49448=FACE_OUTER_BOUND ( 'NONE', #38655, .T. ) ;
#49450=DIRECTION ( 'NONE',  ( -1.000000000000000000, -0.000000000000000000, -0.000000000000000000 ) ) ;
#49474=CARTESIAN_POINT ( 'NONE',  ( -22.50000000000000000, 11.64957080754479968, 0.09999999999999571731 ) ) ;
#49508=CARTESIAN_POINT ( 'NONE',  ( -21.22070241538126112, 6.469946272869613324, 0.09891903053502529297 ) ) ;
#49525=VERTEX_POINT ( 'NONE', #109636 ) ;
#49554=DIRECTION ( 'NONE',  ( 1.000000000000000000, -0.000000000000000000, -0.000000000000000000 ) ) ;
#49568=CYLINDRICAL_SURFACE ( 'NONE', #30140, 11.75000000000000000 ) ;
#49600=ORIENTED_EDGE ( 'NONE', *, *, #247474, .F. ) ;
#49620=DIRECTION ( 'NONE',  ( 0.000000000000000000, 0.000000000000000000, 1.000000000000000000 ) ) ;
#49639=CARTESIAN_POINT ( 'NONE',  ( -21.05000000000000071, 1.835341550224411922, -11.55515129256298046 ) ) ;
#49642=EDGE_CURVE ( 'NONE', #133463, #247150, #88777, .T. ) ;
#49650=EDGE_CURVE ( 'NONE', #103069, #187669, #45223, .T. ) ;
#49709=CIRCLE ( 'NONE', #91411, 0.09999999999999939493 ) ;
#49765=( BOUNDED_CURVE ( )  B_SPLINE_CURVE ( 3, ( #251706, #95204, #211301, #254254 ),
 .UNSPECIFIED., .F., .T. ) 
 B_SPLINE_CURVE_WITH_KNOTS ( ( 4, 4 ),
 ( 3.141592653589793116, 4.712388980384689674 ),
 .UNSPECIFIED. ) 
 CURVE ( )  GEOMETRIC_REPRESENTATION_ITEM ( )  RATIONAL_B_SPLINE_CURVE ( ( 1.000000000000000000, 0.8047378541243649375, 0.8047378541243649375, 1.000000000000000000 ) ) 
 REPRESENTATION_ITEM ( '' )  );
#49773=ORIENTED_EDGE ( 'NONE', *, *, #49074, .T. ) ;
#49778=ORIENTED_EDGE ( 'NONE', *, *, #53486, .T. ) ;
#49782=DIRECTION ( 'NONE',  ( 1.000000000000000000, 0.000000000000000000, -0.000000000000000000 ) ) ;
#49785=CARTESIAN_POINT ( 'NONE',  ( -23.15000000000000213, 11.65000000000000036, -21.35000000000000142 ) ) ;
#49788=CARTESIAN_POINT ( 'NONE',  ( 23.14999999999999503, 11.65000000000000746, -21.35000000000000142 ) ) ;
#49797=AXIS2_PLACEMENT_3D ( 'NONE', #15640, #217627, #75605 ) ;
#49801=AXIS2_PLACEMENT_3D ( 'NONE', #67925, #88750, #206157 ) ;
#49813=CIRCLE ( 'NONE', #195592, 0.09999999999999761857 ) ;
#49829=CARTESIAN_POINT ( 'NONE',  ( -23.15000000000000213, 1.999999999999998224, -20.27537807723789953 ) ) ;
#49855=ORIENTED_EDGE ( 'NONE', *, *, #156202, .F. ) ;
#49863=ORIENTED_EDGE ( 'NONE', *, *, #235477, .F. ) ;
#49872=DIRECTION ( 'NONE',  ( 0.000000000000000000, 0.000000000000000000, -1.000000000000000000 ) ) ;
#49883=CARTESIAN_POINT ( 'NONE',  ( -23.15000000000000213, 4.349999999999999645, -21.35000000000000142 ) ) ;
#49897=ORIENTED_EDGE ( 'NONE', *, *, #240088, .T. ) ;
#49907=SPHERICAL_SURFACE ( 'NONE', #189828, 0.1000000000000000056 ) ;
#49914=CARTESIAN_POINT ( 'NONE',  ( -23.15000000000000213, 11.65000000000000036, 11.75000000000000000 ) ) ;
#49922=DIRECTION ( 'NONE',  ( 1.000000000000000000, -0.000000000000000000, -0.000000000000000000 ) ) ;
#49953=EDGE_CURVE ( 'NONE', #139879, #166580, #153619, .T. ) ;
#49960=VERTEX_POINT ( 'NONE', #85893 ) ;
#50037=DIRECTION ( 'NONE',  ( 2.557131231893036985E-16, -0.8660254037844383745, 0.5000000000000003331 ) ) ;
#50044=CARTESIAN_POINT ( 'NONE',  ( 21.05000000000000071, 0.000000000000000000, -33.50000000000000000 ) ) ;
#50050=DIRECTION ( 'NONE',  ( -1.000000000000000000, -1.875376730785737719E-16, -0.000000000000000000 ) ) ;
#50069=FACE_OUTER_BOUND ( 'NONE', #8122, .T. ) ;
#50127=DIRECTION ( 'NONE',  ( 0.000000000000000000, -0.1298341882520079038, -0.9915357197604846018 ) ) ;
#50143=ORIENTED_EDGE ( 'NONE', *, *, #35571, .T. ) ;
#50158=DIRECTION ( 'NONE',  ( 1.000000000000000000, 0.000000000000000000, 0.000000000000000000 ) ) ;
#50202=DIRECTION ( 'NONE',  ( 0.000000000000000000, 1.000000000000000000, 1.224646799147353207E-16 ) ) ;
#50224=DIRECTION ( 'NONE',  ( -1.000000000000000000, 0.000000000000000000, 0.000000000000000000 ) ) ;
#50229=EDGE_LOOP ( 'NONE', ( #179297, #85356, #28393, #128488 ) ) ;
#50237=DIRECTION ( 'NONE',  ( 7.304098846218134667E-16, -1.000000000000000000, 0.000000000000000000 ) ) ;
#50256=VERTEX_POINT ( 'NONE', #102579 ) ;
#50269=AXIS2_PLACEMENT_3D ( 'NONE', #207954, #218178, #216907 ) ;
#50273=ADVANCED_FACE ( 'NONE', ( #45203 ), #54018, .T. ) ;
#50275=DIRECTION ( 'NONE',  ( -1.000000000000000000, 0.000000000000000000, 0.000000000000000000 ) ) ;
#50281=FACE_OUTER_BOUND ( 'NONE', #236247, .T. ) ;
#50298=DIRECTION ( 'NONE',  ( -0.000000000000000000, 1.000000000000000000, -0.000000000000000000 ) ) ;
#50303=EDGE_CURVE ( 'NONE', #182491, #162495, #78886, .T. ) ;
#50304=CARTESIAN_POINT ( 'NONE',  ( 21.53551880898956838, 6.784797761416324846, 0.09896973457166428900 ) ) ;
#50313=CARTESIAN_POINT ( 'NONE',  ( 21.05000000000000071, 10.72371710470752504, -7.664913569087607570 ) ) ;
#50324=DIRECTION ( 'NONE',  ( 0.000000000000000000, 0.000000000000000000, -1.000000000000000000 ) ) ;
#50374=ADVANCED_FACE ( 'NONE', ( #83011 ), #137177, .T. ) ;
#50378=CARTESIAN_POINT ( 'NONE',  ( 23.14999999999998792, 11.65000000000000036, 0.000000000000000000 ) ) ;
#50405=AXIS2_PLACEMENT_3D ( 'NONE', #174144, #90699, #170296 ) ;
#50439=EDGE_LOOP ( 'NONE', ( #217475, #235929, #190404, #97950 ) ) ;
#50461=AXIS2_PLACEMENT_3D ( 'NONE', #66297, #224064, #166708 ) ;
#50467=DIRECTION ( 'NONE',  ( 1.000000000000000000, 0.000000000000000000, 0.000000000000000000 ) ) ;
#50482=ORIENTED_EDGE ( 'NONE', *, *, #202366, .T. ) ;
#50491=ORIENTED_EDGE ( 'NONE', *, *, #113275, .F. ) ;
#50500=DIRECTION ( 'NONE',  ( 0.000000000000000000, 0.000000000000000000, -1.000000000000000000 ) ) ;
#50509=CYLINDRICAL_SURFACE ( 'NONE', #189048, 0.5000000000000004441 ) ;
#50517=EDGE_CURVE ( 'NONE', #15975, #91559, #62350, .T. ) ;
#50557=ORIENTED_EDGE ( 'NONE', *, *, #138834, .T. ) ;
#50569=ORIENTED_EDGE ( 'NONE', *, *, #172116, .F. ) ;
#50599=CIRCLE ( 'NONE', #246260, 0.1000000000000004774 ) ;
#50712=ORIENTED_EDGE ( 'NONE', *, *, #67140, .F. ) ;
#50718=EDGE_CURVE ( 'NONE', #57106, #197965, #190538, .T. ) ;
#50733=AXIS2_PLACEMENT_3D ( 'NONE', #34001, #129213, #90064 ) ;
#50735=CARTESIAN_POINT ( 'NONE',  ( 20.94999999999999929, 1.835341550224413698, -11.55515129256298401 ) ) ;
#50744=ORIENTED_EDGE ( 'NONE', *, *, #169699, .T. ) ;
#50761=ORIENTED_EDGE ( 'NONE', *, *, #251912, .T. ) ;
#50774=ADVANCED_FACE ( 'NONE', ( #233509 ), #203993, .F. ) ;
#50779=ORIENTED_EDGE ( 'NONE', *, *, #38135, .T. ) ;
#50839=VERTEX_POINT ( 'NONE', #100365 ) ;
#50852=VERTEX_POINT ( 'NONE', #159112 ) ;
#50854=CARTESIAN_POINT ( 'NONE',  ( -21.14999999999999858, -7.589415207398531038E-16, 6.540656951701240729 ) ) ;
#50869=CARTESIAN_POINT ( 'NONE',  ( -21.05000000000000071, 6.304961112684661195, -0.02138556593757447166 ) ) ;
#50875=CIRCLE ( 'NONE', #167456, 0.09999999999999939493 ) ;
#50880=CARTESIAN_POINT ( 'NONE',  ( -18.44362607810621313, -9.490496158084827272, -7.057953866847126001 ) ) ;
#50891=LINE ( 'NONE', #226990, #125432 ) ;
#50895=DIRECTION ( 'NONE',  ( 1.000000000000000000, -0.000000000000000000, -0.000000000000000000 ) ) ;
#50898=CARTESIAN_POINT ( 'NONE',  ( -18.50000000000000000, -9.500000000000005329, -8.099999999999999645 ) ) ;
#50903=VECTOR ( 'NONE', #104337, 1000.000000000000114 ) ;
#50911=B_SPLINE_CURVE_WITH_KNOTS ( 'NONE', 3,
 ( #57726, #173889, #74780, #236376 ),
 .UNSPECIFIED., .F., .F.,
 ( 4, 4 ),
 ( 6.278991785631292523E-18, 0.0001058379652594621054 ),
 .UNSPECIFIED. ) ;
#50928=VECTOR ( 'NONE', #70831, 1000.000000000000000 ) ;
#50947=( BOUNDED_CURVE ( )  B_SPLINE_CURVE ( 3, ( #254750, #215652, #155733, #235233 ),
 .UNSPECIFIED., .F., .F. ) 
 B_SPLINE_CURVE_WITH_KNOTS ( ( 4, 4 ),
 ( 1.570796326794902997, 3.141592653589791784 ),
 .UNSPECIFIED. ) 
 CURVE ( )  GEOMETRIC_REPRESENTATION_ITEM ( )  RATIONAL_B_SPLINE_CURVE ( ( 1.000000000000000000, 0.8047378541243667138, 0.8047378541243667138, 1.000000000000000000 ) ) 
 REPRESENTATION_ITEM ( '' )  );
#50948=ORIENTED_EDGE ( 'NONE', *, *, #241622, .F. ) ;
#50995=DIRECTION ( 'NONE',  ( -1.000000000000000000, -0.000000000000000000, 0.000000000000000000 ) ) ;
#51039=CARTESIAN_POINT ( 'NONE',  ( 21.05000000000000071, -11.48912529307605901, -2.900000000000003464 ) ) ;
#51069=ADVANCED_FACE ( 'NONE', ( #147221 ), #46818, .F. ) ;
#51098=VERTEX_POINT ( 'NONE', #212354 ) ;
#51126=EDGE_LOOP ( 'NONE', ( #96585, #100426, #222115, #107793 ) ) ;
#51133=DIRECTION ( 'NONE',  ( -1.000000000000000000, 0.000000000000000000, 0.000000000000000000 ) ) ;
#51148=CARTESIAN_POINT ( 'NONE',  ( 18.49999999999999289, 11.75000000000000355, -8.099999999999999645 ) ) ;
#51178=EDGE_CURVE ( 'NONE', #71518, #81419, #154351, .T. ) ;
#51197=ADVANCED_FACE ( 'NONE', ( #117089 ), #217440, .T. ) ;
#51198=DIRECTION ( 'NONE',  ( 0.000000000000000000, 0.000000000000000000, 1.000000000000000000 ) ) ;
#51207=CARTESIAN_POINT ( 'NONE',  ( 20.94999999999999574, 0.000000000000000000, 0.000000000000000000 ) ) ;
#51214=CIRCLE ( 'NONE', #67809, 0.09999999999999892308 ) ;
#51231=CARTESIAN_POINT ( 'NONE',  ( -20.94999999999999929, -11.48912529307605901, -2.900000000000001688 ) ) ;
#51257=CARTESIAN_POINT ( 'NONE',  ( 20.94999999999999929, 4.999999999999997335, -21.09473398108690390 ) ) ;
#51262=ORIENTED_EDGE ( 'NONE', *, *, #194064, .F. ) ;
#51281=VERTEX_POINT ( 'NONE', #180912 ) ;
#51310=ORIENTED_EDGE ( 'NONE', *, *, #203286, .F. ) ;
#51317=AXIS2_PLACEMENT_3D ( 'NONE', #157218, #93352, #73831 ) ;
#51319=AXIS2_PLACEMENT_3D ( 'NONE', #161461, #240984, #62351 ) ;
#51329=CARTESIAN_POINT ( 'NONE',  ( 21.05000000000000071, 10.42338541491290727, -7.492051923870097774 ) ) ;
#51334=CARTESIAN_POINT ( 'NONE',  ( 21.14999999999999858, 11.65000000000000746, 11.75000000000000000 ) ) ;
#51343=ORIENTED_EDGE ( 'NONE', *, *, #163327, .F. ) ;
#51358=ORIENTED_EDGE ( 'NONE', *, *, #28610, .T. ) ;
#51361=ORIENTED_EDGE ( 'NONE', *, *, #29942, .T. ) ;
#51366=PLANE ( 'NONE',  #219506 ) ;
#51396=ORIENTED_EDGE ( 'NONE', *, *, #199348, .T. ) ;
#51414=ORIENTED_EDGE ( 'NONE', *, *, #240523, .F. ) ;
#51422=DIRECTION ( 'NONE',  ( 0.000000000000000000, 0.000000000000000000, 1.000000000000000000 ) ) ;
#51423=CARTESIAN_POINT ( 'NONE',  ( -2.995603634470884209E-16, -11.75000000000000000, -12.25000000000000000 ) ) ;
#51436=AXIS2_PLACEMENT_3D ( 'NONE', #146130, #23658, #165725 ) ;
#51470=DIRECTION ( 'NONE',  ( 0.000000000000000000, 0.000000000000000000, -1.000000000000000000 ) ) ;
#51529=EDGE_CURVE ( 'NONE', #193883, #90989, #13823, .T. ) ;
#51530=FACE_OUTER_BOUND ( 'NONE', #35030, .T. ) ;
#51583=DIRECTION ( 'NONE',  ( 0.000000000000000000, 0.000000000000000000, -1.000000000000000000 ) ) ;
#51611=VECTOR ( 'NONE', #61956, 1000.000000000000000 ) ;
#51625=DIRECTION ( 'NONE',  ( 0.000000000000000000, 1.000000000000000000, 0.000000000000000000 ) ) ;
#51655=CIRCLE ( 'NONE', #5876, 0.4000000000000010214 ) ;
#51662=ORIENTED_EDGE ( 'NONE', *, *, #46920, .F. ) ;
#51690=ADVANCED_FACE ( 'NONE', ( #29283 ), #25487, .F. ) ;
#51756=ORIENTED_EDGE ( 'NONE', *, *, #196185, .T. ) ;
#51768=CARTESIAN_POINT ( 'NONE',  ( -22.59999999999999787, 0.1008583690987122083, 11.74956712348939192 ) ) ;
#51790=ORIENTED_EDGE ( 'NONE', *, *, #233988, .F. ) ;
#51800=ORIENTED_EDGE ( 'NONE', *, *, #230181, .T. ) ;
#51831=AXIS2_PLACEMENT_3D ( 'NONE', #147849, #86545, #227366 ) ;
#51839=CARTESIAN_POINT ( 'NONE',  ( -23.15000000000000213, -9.000000000000001776, -24.10603087734756045 ) ) ;
#51867=CARTESIAN_POINT ( 'NONE',  ( 21.05000000000000071, 10.72371711692550100, -12.17623960113813020 ) ) ;
#51900=ORIENTED_EDGE ( 'NONE', *, *, #155228, .F. ) ;
#51902=DIRECTION ( 'NONE',  ( 1.000000000000000000, 0.000000000000000000, 0.000000000000000000 ) ) ;
#51903=FACE_OUTER_BOUND ( 'NONE', #133679, .T. ) ;
#51919=CARTESIAN_POINT ( 'NONE',  ( -18.59999999999999787, -9.480686695278976117, -40.44111516875784673 ) ) ;
#51925=STYLED_ITEM ( 'NONE', ( #74929 ), #157328 ) ;
#51932=CARTESIAN_POINT ( 'NONE',  ( -20.94999999999999929, -11.41227409414968719, -3.000000000000002665 ) ) ;
#51949=VECTOR ( 'NONE', #12867, 1000.000000000000000 ) ;
#51995=CARTESIAN_POINT ( 'NONE',  ( -23.15000000000000213, 0.000000000000000000, -4.049999999999998934 ) ) ;
#52039=VERTEX_POINT ( 'NONE', #196028 ) ;
#52059=DIRECTION ( 'NONE',  ( 1.000000000000000000, 0.000000000000000000, 0.000000000000000000 ) ) ;
#52069=EDGE_CURVE ( 'NONE', #17135, #140018, #58956, .T. ) ;
#52092=DIRECTION ( 'NONE',  ( -0.7071067811865388020, 0.7071067811865561215, 0.000000000000000000 ) ) ;
#52108=AXIS2_PLACEMENT_3D ( 'NONE', #128720, #70047, #149583 ) ;
#52139=VERTEX_POINT ( 'NONE', #25107 ) ;
#52140=AXIS2_PLACEMENT_3D ( 'NONE', #49062, #167763, #103883 ) ;
#52141=DIRECTION ( 'NONE',  ( -1.000000000000000000, -0.000000000000000000, -0.000000000000000000 ) ) ;
#52177=EDGE_CURVE ( 'NONE', #113692, #55133, #225817, .T. ) ;
#52178=CARTESIAN_POINT ( 'NONE',  ( -18.47653818581420637, -9.465280387762964764, -7.125960816139832232 ) ) ;
#52246=CARTESIAN_POINT ( 'NONE',  ( 23.14999999999998437, 0.000000000000000000, 0.000000000000000000 ) ) ;
#52285=CARTESIAN_POINT ( 'NONE',  ( 21.12757541349815682, 6.473380571251452942, 0.005161215809745128835 ) ) ;
#52302=LINE ( 'NONE', #172326, #37968 ) ;
#52317=SPHERICAL_SURFACE ( 'NONE', #14592, 0.1000000000000000056 ) ;
#52320=FACE_OUTER_BOUND ( 'NONE', #50229, .T. ) ;
#52327=DIRECTION ( 'NONE',  ( -0.000000000000000000, 1.000000000000000000, 1.734723475976807292E-15 ) ) ;
#52340=DIRECTION ( 'NONE',  ( 0.000000000000000000, -0.000000000000000000, 1.000000000000000000 ) ) ;
#52341=CIRCLE ( 'NONE', #47677, 6.258578643762712446 ) ;
#52349=ORIENTED_EDGE ( 'NONE', *, *, #105692, .F. ) ;
#52388=EDGE_CURVE ( 'NONE', #103673, #106788, #38328, .T. ) ;
#52389=FACE_OUTER_BOUND ( 'NONE', #183034, .T. ) ;
#52396=ORIENTED_EDGE ( 'NONE', *, *, #125305, .T. ) ;
#52410=CARTESIAN_POINT ( 'NONE',  ( 18.59999999999998366, 0.000000000000000000, -33.50000000000000000 ) ) ;
#52427=CARTESIAN_POINT ( 'NONE',  ( 21.05000000000000071, -9.000000000000000000, -23.60603087734755690 ) ) ;
#52480=ORIENTED_EDGE ( 'NONE', *, *, #240919, .F. ) ;
#52498=CARTESIAN_POINT ( 'NONE',  ( -21.14999999999999858, -11.75000000000000000, -2.900000000000001688 ) ) ;
#52512=EDGE_CURVE ( 'NONE', #238460, #179010, #129880, .T. ) ;
#52522=CARTESIAN_POINT ( 'NONE',  ( 21.14999999999999503, 11.75000000000000000, -3.469446951953614189E-15 ) ) ;
#52523=CIRCLE ( 'NONE', #44366, 0.09999999999999982514 ) ;
#52573=LINE ( 'NONE', #94272, #6045 ) ;
#52625=CIRCLE ( 'NONE', #65290, 0.1000000000000008799 ) ;
#52653=DIRECTION ( 'NONE',  ( -1.000000000000000000, -0.000000000000000000, -0.000000000000000000 ) ) ;
#52673=ORIENTED_EDGE ( 'NONE', *, *, #229146, .F. ) ;
#52680=ORIENTED_EDGE ( 'NONE', *, *, #249892, .F. ) ;
#52704=VERTEX_POINT ( 'NONE', #16540 ) ;
#52718=DIRECTION ( 'NONE',  ( 0.000000000000000000, 9.769962616701377556E-15, 1.000000000000000000 ) ) ;
#52722=EDGE_CURVE ( 'NONE', #175406, #230288, #192395, .T. ) ;
#52731=AXIS2_PLACEMENT_3D ( 'NONE', #189945, #249915, #71298 ) ;
#52732=DIRECTION ( 'NONE',  ( 0.000000000000000000, 2.891205793294679805E-16, -1.000000000000000000 ) ) ;
#52761=DIRECTION ( 'NONE',  ( 0.000000000000000000, 0.1350103645451876666, -0.9908441862701600211 ) ) ;
#52787=ORIENTED_EDGE ( 'NONE', *, *, #234296, .F. ) ;
#52820=EDGE_LOOP ( 'NONE', ( #186963, #120121, #174081, #163922 ) ) ;
#52863=DIRECTION ( 'NONE',  ( 1.000000000000000000, 0.000000000000000000, -0.000000000000000000 ) ) ;
#52898=FACE_OUTER_BOUND ( 'NONE', #46691, .T. ) ;
#52933=CARTESIAN_POINT ( 'NONE',  ( -20.54999999999999716, 4.349999999999999645, -12.35000000000000142 ) ) ;
#53027=DIRECTION ( 'NONE',  ( 0.000000000000000000, -0.9908441862701596881, 0.1350103645451904977 ) ) ;
#53052=LINE ( 'NONE', #188713, #26585 ) ;
#53164=CARTESIAN_POINT ( 'NONE',  ( -21.05000000000000071, 1.162701749938009677, -8.099999999999999645 ) ) ;
#53180=EDGE_CURVE ( 'NONE', #153971, #94181, #25648, .T. ) ;
#53187=FACE_OUTER_BOUND ( 'NONE', #254143, .T. ) ;
#53188=VECTOR ( 'NONE', #253415, 1000.000000000000114 ) ;
#53193=DIRECTION ( 'NONE',  ( 1.000000000000000000, 0.000000000000000000, -0.000000000000000000 ) ) ;
#53205=FACE_OUTER_BOUND ( 'NONE', #91831, .T. ) ;
#53215=CARTESIAN_POINT ( 'NONE',  ( 18.59999999999999432, 1.162701749938009677, -8.099999999999999645 ) ) ;
#53231=CARTESIAN_POINT ( 'NONE',  ( -18.50000000000000000, -9.421290279523317324, -40.32388217902604310 ) ) ;
#53255=EDGE_LOOP ( 'NONE', ( #147139, #92782, #233219, #125832 ) ) ;
#53260=CARTESIAN_POINT ( 'NONE',  ( -23.15000000000000213, -8.663551401869156621, -23.97589888193269658 ) ) ;
#53261=ADVANCED_FACE ( 'NONE', ( #159587 ), #162171, .T. ) ;
#53284=CARTESIAN_POINT ( 'NONE',  ( 18.39999999999999503, -9.499999999999996447, -6.999362097180139131 ) ) ;
#53297=CARTESIAN_POINT ( 'NONE',  ( 18.60000000000000142, -9.480686695278970788, -40.44111516875785384 ) ) ;
#53319=VECTOR ( 'NONE', #200291, 1000.000000000000000 ) ;
#53339=ORIENTED_EDGE ( 'NONE', *, *, #185465, .T. ) ;
#53341=CARTESIAN_POINT ( 'NONE',  ( -20.54999999999999716, 7.249999999999999112, -21.25000000000000000 ) ) ;
#53347=AXIS2_PLACEMENT_3D ( 'NONE', #102408, #163711, #223658 ) ;
#53350=EDGE_LOOP ( 'NONE', ( #49773, #60680, #62481, #67815 ) ) ;
#53357=EDGE_CURVE ( 'NONE', #67636, #204739, #104710, .T. ) ;
#53381=EDGE_CURVE ( 'NONE', #180654, #171717, #250497, .T. ) ;
#53389=CIRCLE ( 'NONE', #95079, 0.09999999999999954758 ) ;
#53391=ORIENTED_EDGE ( 'NONE', *, *, #80279, .T. ) ;
#53396=FACE_OUTER_BOUND ( 'NONE', #176773, .T. ) ;
#53421=ORIENTED_EDGE ( 'NONE', *, *, #162211, .F. ) ;
#53422=LINE ( 'NONE', #75582, #18164 ) ;
#53436=FACE_OUTER_BOUND ( 'NONE', #15571, .T. ) ;
#53443=CIRCLE ( 'NONE', #95133, 0.09999999999999939493 ) ;
#53446=CARTESIAN_POINT ( 'NONE',  ( 22.39999999999999503, 0.000000000000000000, 11.64957080754479968 ) ) ;
#53486=EDGE_CURVE ( 'NONE', #170111, #240969, #121371, .T. ) ;
#53497=CARTESIAN_POINT ( 'NONE',  ( 23.24999999999997513, 11.65000000000000746, -26.48519422934605672 ) ) ;
#53507=ORIENTED_EDGE ( 'NONE', *, *, #55829, .F. ) ;
#53538=DIRECTION ( 'NONE',  ( 0.000000000000000000, -0.000000000000000000, -1.000000000000000000 ) ) ;
#53547=FACE_OUTER_BOUND ( 'NONE', #121318, .T. ) ;
#53552=EDGE_LOOP ( 'NONE', ( #58565, #1047, #93679, #249201 ) ) ;
#53603=VERTEX_POINT ( 'NONE', #75892 ) ;
#53607=DIRECTION ( 'NONE',  ( -0.000000000000000000, -0.000000000000000000, -1.000000000000000000 ) ) ;
#53632=VERTEX_POINT ( 'NONE', #41606 ) ;
#53658=ORIENTED_EDGE ( 'NONE', *, *, #230123, .F. ) ;
#53660=ORIENTED_EDGE ( 'NONE', *, *, #237096, .F. ) ;
#53678=ORIENTED_EDGE ( 'NONE', *, *, #189097, .T. ) ;
#53700=DIRECTION ( 'NONE',  ( 1.000000000000000000, 6.938893903907222067E-15, 0.000000000000000000 ) ) ;
#53732=LINE ( 'NONE', #14631, #161448 ) ;
#53746=DIRECTION ( 'NONE',  ( -1.000000000000000000, -0.000000000000000000, -0.000000000000000000 ) ) ;
#53748=ORIENTED_EDGE ( 'NONE', *, *, #81527, .F. ) ;
#53766=EDGE_CURVE ( 'NONE', #4734, #162626, #186232, .T. ) ;
#53768=ORIENTED_EDGE ( 'NONE', *, *, #193579, .T. ) ;
#53784=DIRECTION ( 'NONE',  ( -0.000000000000000000, -0.8660254037844459241, -0.4999999999999873990 ) ) ;
#53785=ADVANCED_FACE ( 'NONE', ( #64985, #84504 ), #184938, .F. ) ;
#53809=AXIS2_PLACEMENT_3D ( 'NONE', #133272, #57564, #113704 ) ;
#53831=AXIS2_PLACEMENT_3D ( 'NONE', #63879, #65150, #142124 ) ;
#53863=CYLINDRICAL_SURFACE ( 'NONE', #101242, 0.5000000000000004441 ) ;
#53883=DIRECTION ( 'NONE',  ( 0.000000000000000000, 0.4930308989875165082, 0.8700118002898358238 ) ) ;
#53895=ORIENTED_EDGE ( 'NONE', *, *, #120942, .T. ) ;
#53901=CARTESIAN_POINT ( 'NONE',  ( -23.15000000000000213, 11.65000000000000036, -12.15000000000000036 ) ) ;
#53914=DIRECTION ( 'NONE',  ( 1.000000000000000000, 0.000000000000000000, 0.000000000000000000 ) ) ;
#53930=DIRECTION ( 'NONE',  ( -1.000000000000000000, -1.040834085586090568E-13, 0.000000000000000000 ) ) ;
#53984=DIRECTION ( 'NONE',  ( 1.000000000000000000, -0.000000000000000000, -0.000000000000000000 ) ) ;
#54017=DIRECTION ( 'NONE',  ( -1.000000000000000000, 0.000000000000000000, 0.000000000000000000 ) ) ;
#54018=( BOUNDED_SURFACE ( )  B_SPLINE_SURFACE ( 3, 2, ( 
 ( #46471, #68629, #43921 ),
 ( #127311, #85572, #47752 ),
 ( #124752, #206849, #84272 ),
 ( #183443, #145578, #6066 ),
 ( #144275, #25649, #223823 ),
 ( #126015, #105132, #29527 ),
 ( #109015, #4766, #204263 ),
 ( #24382, #28245, #205545 ) ),
 .UNSPECIFIED., .F., .F., .F. ) 
 B_SPLINE_SURFACE_WITH_KNOTS ( ( 4, 2, 2, 4 ),
 ( 3, 3 ),
 ( 0.0001723339234021441008, 0.0002782939632049931823, 0.0003842540030078422908, 0.0005961740826135404538 ),
 ( 0.000000000000000000, 1.000000000000000000 ),
 .UNSPECIFIED. ) 
 GEOMETRIC_REPRESENTATION_ITEM ( )  RATIONAL_B_SPLINE_SURFACE ( (
 ( 1.000000000000000000, 0.9504532311154585411, 1.000000000000000000),
 ( 1.000000000000000000, 0.9506023220709699517, 1.000000000000000000),
 ( 1.000000000000000000, 0.9395774818181729104, 1.000000000000000000),
 ( 1.000000000000000000, 0.9079328464647203889, 1.000000000000000000),
 ( 1.000000000000000000, 0.8875702416204832579, 1.000000000000000000),
 ( 1.000000000000000000, 0.8205919608041678526, 1.000000000000000000),
 ( 1.000000000000000000, 0.7666842783597330735, 1.000000000000000000),
 ( 1.000000000000000000, 0.7071067811864603092, 1.000000000000000000) ) ) 
 REPRESENTATION_ITEM ( '' )  SURFACE ( )  );
#54070=AXIS2_PLACEMENT_3D ( 'NONE', #188251, #89142, #168745 ) ;
#54073=DIRECTION ( 'NONE',  ( 1.000000000000000000, 3.265361837132813093E-16, -0.000000000000000000 ) ) ;
#54103=DIRECTION ( 'NONE',  ( -1.000000000000000000, 0.000000000000000000, 0.000000000000000000 ) ) ;
#54109=FACE_OUTER_BOUND ( 'NONE', #88918, .T. ) ;
#54130=ADVANCED_FACE ( 'NONE', ( #161225 ), #245895, .T. ) ;
#54132=ORIENTED_EDGE ( 'NONE', *, *, #164510, .T. ) ;
#54140=DIRECTION ( 'NONE',  ( -0.000000000000000000, -0.9875055080513799322, 0.1575844902526464253 ) ) ;
#54150=CARTESIAN_POINT ( 'NONE',  ( -23.15000000000000213, -11.65000000000000036, -30.39999999999999503 ) ) ;
#54176=CARTESIAN_POINT ( 'NONE',  ( 21.05000000000000071, 10.62872031400434736, -7.664913569087605794 ) ) ;
#54179=EDGE_CURVE ( 'NONE', #54887, #129010, #46840, .T. ) ;
#54180=LINE ( 'NONE', #68627, #215450 ) ;
#54186=CARTESIAN_POINT ( 'NONE',  ( -20.64999999999999858, -9.000000000000003553, -9.393969122652443104 ) ) ;
#54240=CIRCLE ( 'NONE', #249888, 1.900000000000005906 ) ;
#54274=CARTESIAN_POINT ( 'NONE',  ( 22.47007471830798053, 1.834461605516000565E-15, 7.720710651926451895 ) ) ;
#54301=DIRECTION ( 'NONE',  ( 0.000000000000000000, 0.000000000000000000, 1.000000000000000000 ) ) ;
#54316=DIRECTION ( 'NONE',  ( 0.000000000000000000, 0.000000000000000000, 1.000000000000000000 ) ) ;
#54326=CARTESIAN_POINT ( 'NONE',  ( -22.59080734064477625, 11.75000000000000355, 0.03074970809701978169 ) ) ;
#54355=EDGE_CURVE ( 'NONE', #90335, #20565, #180321, .T. ) ;
#54370=CARTESIAN_POINT ( 'NONE',  ( -23.15000000000000213, 0.000000000000000000, -33.50000000000000000 ) ) ;
#54383=DIRECTION ( 'NONE',  ( 0.000000000000000000, 0.000000000000000000, 1.000000000000000000 ) ) ;
#54396=PLANE ( 'NONE',  #166882 ) ;
#54434=DIRECTION ( 'NONE',  ( 1.000000000000000000, -0.000000000000000000, -0.000000000000000000 ) ) ;
#54467=ORIENTED_EDGE ( 'NONE', *, *, #50718, .F. ) ;
#54509=LINE ( 'NONE', #111943, #220319 ) ;
#54512=AXIS2_PLACEMENT_3D ( 'NONE', #200724, #39103, #118638 ) ;
#54518=AXIS2_PLACEMENT_3D ( 'NONE', #221291, #239604, #218725 ) ;
#54554=CARTESIAN_POINT ( 'NONE',  ( 18.39999999999999858, -9.519327731092435130, -6.972976376559340217 ) ) ;
#54564=ORIENTED_EDGE ( 'NONE', *, *, #121316, .F. ) ;
#54576=EDGE_CURVE ( 'NONE', #213315, #40685, #33002, .T. ) ;
#54598=DIRECTION ( 'NONE',  ( 1.000000000000000000, 0.000000000000000000, 0.000000000000000000 ) ) ;
#54649=ORIENTED_EDGE ( 'NONE', *, *, #38397, .T. ) ;
#54676=DIRECTION ( 'NONE',  ( 0.000000000000000000, 0.9876197685951252359, -0.1568667991644863424 ) ) ;
#54783=CIRCLE ( 'NONE', #200534, 11.89999999999999858 ) ;
#54786=DIRECTION ( 'NONE',  ( -1.000000000000000000, 0.000000000000000000, 0.000000000000000000 ) ) ;
#54848=DIRECTION ( 'NONE',  ( 0.000000000000000000, 0.6728971962616869806, -0.7397360091702719354 ) ) ;
#54887=VERTEX_POINT ( 'NONE', #144875 ) ;
#54915=LINE ( 'NONE', #254387, #25182 ) ;
#54939=CARTESIAN_POINT ( 'NONE',  ( -23.15000000000000213, -11.48912529307605546, -30.50000000000000000 ) ) ;
#54952=CARTESIAN_POINT ( 'NONE',  ( 18.59999999999996945, 10.33248238082518711, -39.09484654391314962 ) ) ;
#54991=EDGE_CURVE ( 'NONE', #251409, #60900, #31401, .T. ) ;
#54995=ORIENTED_EDGE ( 'NONE', *, *, #75518, .T. ) ;
#55007=EDGE_LOOP ( 'NONE', ( #60397, #208724, #104882, #43835 ) ) ;
#55039=FACE_OUTER_BOUND ( 'NONE', #254899, .T. ) ;
#55077=DIRECTION ( 'NONE',  ( 0.000000000000000000, 0.000000000000000000, 1.000000000000000000 ) ) ;
#55079=ORIENTED_EDGE ( 'NONE', *, *, #63523, .T. ) ;
#55082=CYLINDRICAL_SURFACE ( 'NONE', #15014, 0.09999999999999939493 ) ;
#55085=ADVANCED_FACE ( 'NONE', ( #150047 ), #70526, .F. ) ;
#55095=FACE_OUTER_BOUND ( 'NONE', #208988, .T. ) ;
#55126=CARTESIAN_POINT ( 'NONE',  ( -18.59999999999999787, -26.43935341560094443, -18.14150860750746475 ) ) ;
#55133=VERTEX_POINT ( 'NONE', #33979 ) ;
#55164=VECTOR ( 'NONE', #246475, 999.9999999999998863 ) ;
#55174=DIRECTION ( 'NONE',  ( 0.000000000000000000, 0.000000000000000000, -1.000000000000000000 ) ) ;
#55187=CIRCLE ( 'NONE', #238374, 0.09999999999999761857 ) ;
#55241=ORIENTED_EDGE ( 'NONE', *, *, #183659, .F. ) ;
#55267=VECTOR ( 'NONE', #210380, 1000.000000000000000 ) ;
#55275=DIRECTION ( 'NONE',  ( 0.000000000000000000, 0.000000000000000000, 1.000000000000000000 ) ) ;
#55276=CARTESIAN_POINT ( 'NONE',  ( -18.59999999999999787, 1.162701749938009677, -8.099999999999999645 ) ) ;
#55309=CYLINDRICAL_SURFACE ( 'NONE', #170474, 11.74999999999999645 ) ;
#55315=CARTESIAN_POINT ( 'NONE',  ( 21.06490991615909536, 10.72489134758711238, -12.20371135353312830 ) ) ;
#55327=ORIENTED_EDGE ( 'NONE', *, *, #96836, .T. ) ;
#55353=DIRECTION ( 'NONE',  ( 1.000000000000000000, 0.000000000000000000, 0.000000000000000000 ) ) ;
#55355=CARTESIAN_POINT ( 'NONE',  ( 21.14999999999999858, -0.09999999999999939493, 6.540656951701244282 ) ) ;
#55356=ORIENTED_EDGE ( 'NONE', *, *, #69326, .F. ) ;
#55358=CARTESIAN_POINT ( 'NONE',  ( -23.15000000000000213, 1.999999999999998224, -20.77537807723789953 ) ) ;
#55364=VECTOR ( 'NONE', #76482, 1000.000000000000000 ) ;
#55377=AXIS2_PLACEMENT_3D ( 'NONE', #163632, #161067, #1958 ) ;
#55379=EDGE_CURVE ( 'NONE', #172600, #225538, #51655, .T. ) ;
#55408=AXIS2_PLACEMENT_3D ( 'NONE', #116190, #131881, #195735 ) ;
#55454=CARTESIAN_POINT ( 'NONE',  ( 23.14999999999999147, 0.000000000000000000, 0.000000000000000000 ) ) ;
#55469=ADVANCED_FACE ( 'NONE', ( #56673 ), #75025, .T. ) ;
#55501=EDGE_LOOP ( 'NONE', ( #230470, #75316, #64775, #127019, #188659 ) ) ;
#55509=VERTEX_POINT ( 'NONE', #236620 ) ;
#55523=ORIENTED_EDGE ( 'NONE', *, *, #234368, .T. ) ;
#55529=CIRCLE ( 'NONE', #192963, 0.5999999999999998668 ) ;
#55530=DIRECTION ( 'NONE',  ( 1.000000000000000000, 0.000000000000000000, 0.000000000000000000 ) ) ;
#55560=DIRECTION ( 'NONE',  ( 0.000000000000000000, 0.000000000000000000, -1.000000000000000000 ) ) ;
#55611=CARTESIAN_POINT ( 'NONE',  ( -18.46902351632713035, -9.509470118680869888, -6.986453934257316867 ) ) ;
#55678=EDGE_LOOP ( 'NONE', ( #6311, #126468, #67675, #115085 ) ) ;
#55688=VECTOR ( 'NONE', #247932, 1000.000000000000000 ) ;
#55708=CARTESIAN_POINT ( 'NONE',  ( 20.94999999999999574, 1.162701749938009677, -8.099999999999999645 ) ) ;
#55758=CARTESIAN_POINT ( 'NONE',  ( 21.05000000000000071, -8.730841121495327428, -9.598074718984332065 ) ) ;
#55768=ORIENTED_EDGE ( 'NONE', *, *, #127259, .T. ) ;
#55784=DIRECTION ( 'NONE',  ( 2.694716079187272946E-16, -1.000000000000000000, 0.000000000000000000 ) ) ;
#55791=EDGE_LOOP ( 'NONE', ( #243649, #80888, #122806, #98019 ) ) ;
#55793=CARTESIAN_POINT ( 'NONE',  ( -21.05000000000000426, 6.332272273935660500, -0.03753606328566801847 ) ) ;
#55803=FACE_OUTER_BOUND ( 'NONE', #28801, .T. ) ;
#55811=ORIENTED_EDGE ( 'NONE', *, *, #230789, .T. ) ;
#55815=CIRCLE ( 'NONE', #176673, 0.09999999999999939493 ) ;
#55821=CARTESIAN_POINT ( 'NONE',  ( 18.46163235739470920, -9.480150806918276274, -40.15761053987758800 ) ) ;
#55829=EDGE_CURVE ( 'NONE', #169542, #251285, #22857, .T. ) ;
#55855=DIRECTION ( 'NONE',  ( 0.000000000000000000, 0.000000000000000000, -1.000000000000000000 ) ) ;
#55880=ADVANCED_FACE ( 'NONE', ( #77246 ), #7563, .T. ) ;
#55935=FACE_OUTER_BOUND ( 'NONE', #148903, .T. ) ;
#55955=AXIS2_PLACEMENT_3D ( 'NONE', #130036, #186187, #187483 ) ;
#55965=ORIENTED_EDGE ( 'NONE', *, *, #198069, .F. ) ;
#55980=CARTESIAN_POINT ( 'NONE',  ( 22.49999999999999645, 0.08880997638693272078, 11.64976291803192154 ) ) ;
#55982=CARTESIAN_POINT ( 'NONE',  ( -20.94999999999999929, 0.000000000000000000, -33.50000000000000000 ) ) ;
#55986=DIRECTION ( 'NONE',  ( 0.000000000000000000, -1.000000000000000000, 0.000000000000000000 ) ) ;
#56004=CARTESIAN_POINT ( 'NONE',  ( 20.94999999999999929, -9.000000000000001776, -9.893969122652443104 ) ) ;
#56011=DIRECTION ( 'NONE',  ( 0.000000000000000000, 0.008583690987127922528, 0.9999631594459055250 ) ) ;
#56071=DIRECTION ( 'NONE',  ( -0.000000000000000000, 1.000000000000000000, -0.000000000000000000 ) ) ;
#56092=CARTESIAN_POINT ( 'NONE',  ( 23.14999999999999503, 11.65000000000000746, -12.25000000000000000 ) ) ;
#56107=ADVANCED_FACE ( 'NONE', ( #88787 ), #148799, .T. ) ;
#56135=EDGE_CURVE ( 'NONE', #231683, #214079, #31069, .T. ) ;
#56177=DIRECTION ( 'NONE',  ( -1.000000000000000000, -7.304098846218134667E-16, 0.000000000000000000 ) ) ;
#56184=VERTEX_POINT ( 'NONE', #156531 ) ;
#56194=VERTEX_POINT ( 'NONE', #152673 ) ;
#56198=DIRECTION ( 'NONE',  ( 0.000000000000000000, 0.000000000000000000, 1.000000000000000000 ) ) ;
#56235=AXIS2_PLACEMENT_3D ( 'NONE', #85391, #244502, #125833 ) ;
#56255=AXIS2_PLACEMENT_3D ( 'NONE', #6122, #163939, #183499 ) ;
#56332=VECTOR ( 'NONE', #129871, 1000.000000000000000 ) ;
#56353=EDGE_CURVE ( 'NONE', #106103, #249368, #93745, .T. ) ;
#56356=CARTESIAN_POINT ( 'NONE',  ( 20.85000000000000142, 0.1610488207187191212, -33.21581015563977957 ) ) ;
#56393=DIRECTION ( 'NONE',  ( 0.000000000000000000, 0.9274965247785529332, 0.3738317757009255171 ) ) ;
#56398=VERTEX_POINT ( 'NONE', #71013 ) ;
#56439=EDGE_CURVE ( 'NONE', #218249, #129969, #77171, .T. ) ;
#56441=AXIS2_PLACEMENT_3D ( 'NONE', #201648, #125952, #202931 ) ;
#56447=DIRECTION ( 'NONE',  ( 0.000000000000000000, 0.000000000000000000, -1.000000000000000000 ) ) ;
#56466=EDGE_CURVE ( 'NONE', #73461, #256381, #18735, .T. ) ;
#56467=VERTEX_POINT ( 'NONE', #11014 ) ;
#56468=VECTOR ( 'NONE', #246418, 1000.000000000000000 ) ;
#56505=DIRECTION ( 'NONE',  ( -0.000000000000000000, 0.000000000000000000, 1.000000000000000000 ) ) ;
#56529=EDGE_LOOP ( 'NONE', ( #250358, #72252, #67200, #188205, #238764 ) ) ;
#56536=VERTEX_POINT ( 'NONE', #155692 ) ;
#56539=DIRECTION ( 'NONE',  ( 0.000000000000000000, 0.000000000000000000, -1.000000000000000000 ) ) ;
#56567=EDGE_CURVE ( 'NONE', #234900, #68838, #143987, .T. ) ;
#56598=CARTESIAN_POINT ( 'NONE',  ( 21.08750232978087524, 10.72486338601016520, -12.22885817299956912 ) ) ;
#56645=DIRECTION ( 'NONE',  ( 0.000000000000000000, 0.000000000000000000, -1.000000000000000000 ) ) ;
#56668=VECTOR ( 'NONE', #230971, 1000.000000000000114 ) ;
#56673=FACE_OUTER_BOUND ( 'NONE', #148054, .T. ) ;
#56684=CARTESIAN_POINT ( 'NONE',  ( 20.94999999999999929, -1.135018845910178431, -41.21697688343231647 ) ) ;
#56685=ORIENTED_EDGE ( 'NONE', *, *, #25433, .F. ) ;
#56721=ADVANCED_FACE ( 'NONE', ( #146034 ), #23224, .T. ) ;
#56752=CARTESIAN_POINT ( 'NONE',  ( 20.04142135623730070, 11.75000000000000355, -24.65000000000000213 ) ) ;
#56803=AXIS2_PLACEMENT_3D ( 'NONE', #146941, #128695, #68713 ) ;
#56815=VERTEX_POINT ( 'NONE', #72961 ) ;
#56818=CARTESIAN_POINT ( 'NONE',  ( 21.93340585898732442, -5.963111948670274387E-16, 7.324147022127360351 ) ) ;
#56903=DIRECTION ( 'NONE',  ( 0.000000000000000000, 1.000000000000000000, 0.000000000000000000 ) ) ;
#56955=VERTEX_POINT ( 'NONE', #58469 ) ;
#56985=AXIS2_PLACEMENT_3D ( 'NONE', #151884, #9767, #89297 ) ;
#56994=DIRECTION ( 'NONE',  ( 0.000000000000000000, 1.000000000000000000, 0.000000000000000000 ) ) ;
#57001=DIRECTION ( 'NONE',  ( 0.000000000000000000, 0.000000000000000000, -1.000000000000000000 ) ) ;
#57055=CARTESIAN_POINT ( 'NONE',  ( 21.05000000000000071, 6.304516329264039598, -0.02110330805900034398 ) ) ;
#57098=DIRECTION ( 'NONE',  ( 1.000000000000000000, 3.265361837132813093E-16, -0.000000000000000000 ) ) ;
#57104=EDGE_CURVE ( 'NONE', #176398, #202160, #73301, .T. ) ;
#57106=VERTEX_POINT ( 'NONE', #7504 ) ;
#57123=CARTESIAN_POINT ( 'NONE',  ( -21.04999999999999716, 11.74999999999999645, -6.783865662978152855 ) ) ;
#57146=ORIENTED_EDGE ( 'NONE', *, *, #95023, .T. ) ;
#57152=TOROIDAL_SURFACE ( 'NONE', #123833, 0.2000000000000000111, 0.1000000000000000056 ) ;
#57177=AXIS2_PLACEMENT_3D ( 'NONE', #225852, #169812, #145060 ) ;
#57184=CIRCLE ( 'NONE', #74004, 0.09999999999999939493 ) ;
#57251=CARTESIAN_POINT ( 'NONE',  ( -23.25000000000000000, 11.75000000000000000, 0.000000000000000000 ) ) ;
#57270=CARTESIAN_POINT ( 'NONE',  ( 20.74625933824092172, 8.882913521084280006, -8.555171024121042578 ) ) ;
#57274=CARTESIAN_POINT ( 'NONE',  ( 23.15000000000000213, -11.65000000000000036, 3.469446951953614189E-15 ) ) ;
#57298=CARTESIAN_POINT ( 'NONE',  ( -22.49917693094574389, 0.08522996422167167241, 11.64979578453066367 ) ) ;
#57352=DIRECTION ( 'NONE',  ( 1.000000000000000000, -0.000000000000000000, -0.000000000000000000 ) ) ;
#57361=ADVANCED_FACE ( 'NONE', ( #17754 ), #169351, .T. ) ;
#57369=DIRECTION ( 'NONE',  ( -1.000000000000000000, 0.000000000000000000, 0.000000000000000000 ) ) ;
#57384=CIRCLE ( 'NONE', #7505, 11.75000000000000000 ) ;
#57389=EDGE_CURVE ( 'NONE', #131644, #81419, #206715, .T. ) ;
#57395=DIRECTION ( 'NONE',  ( 0.000000000000000000, 0.1350103645451876666, -0.9908441862701600211 ) ) ;
#57416=LINE ( 'NONE', #113558, #171026 ) ;
#57440=DIRECTION ( 'NONE',  ( 0.000000000000000000, 1.000000000000000000, 0.000000000000000000 ) ) ;
#57451=ORIENTED_EDGE ( 'NONE', *, *, #10764, .T. ) ;
#57465=CARTESIAN_POINT ( 'NONE',  ( 20.95545211741311320, 10.58641331154394472, -7.586146859588289715 ) ) ;
#57478=TOROIDAL_SURFACE ( 'NONE', #74282, 0.4000000000000010214, 0.1000000000000000056 ) ;
#57511=ADVANCED_FACE ( 'NONE', ( #45042 ), #68468, .F. ) ;
#57548=VERTEX_POINT ( 'NONE', #63308 ) ;
#57564=DIRECTION ( 'NONE',  ( 0.000000000000000000, -0.000000000000000000, 1.000000000000000000 ) ) ;
#57566=AXIS2_PLACEMENT_3D ( 'NONE', #111537, #35869, #97059 ) ;
#57577=EDGE_CURVE ( 'NONE', #17846, #58858, #252495, .T. ) ;
#57615=AXIS2_PLACEMENT_3D ( 'NONE', #174023, #52732, #196115 ) ;
#57643=DIRECTION ( 'NONE',  ( -1.000000000000000000, -2.952720810173289112E-16, 0.000000000000000000 ) ) ;
#57648=EDGE_LOOP ( 'NONE', ( #4890, #58769, #28012 ) ) ;
#57668=CARTESIAN_POINT ( 'NONE',  ( -18.39999999999999858, -9.682403433476396870, -40.15684337741279109 ) ) ;
#57703=AXIS2_PLACEMENT_3D ( 'NONE', #142254, #2730, #41903 ) ;
#57726=CARTESIAN_POINT ( 'NONE',  ( 22.57320508075687115, 11.75000000000000000, 0.000000000000000000 ) ) ;
#57731=EDGE_CURVE ( 'NONE', #177411, #140135, #87513, .T. ) ;
#57734=FACE_OUTER_BOUND ( 'NONE', #103121, .T. ) ;
#57740=DIRECTION ( 'NONE',  ( 1.000000000000000000, 3.469446951953704435E-14, -2.003086131649669752E-14 ) ) ;
#57746=DIRECTION ( 'NONE',  ( 0.000000000000000000, 0.000000000000000000, -1.000000000000000000 ) ) ;
#57761=DIRECTION ( 'NONE',  ( -1.000000000000000000, -0.000000000000000000, 0.000000000000000000 ) ) ;
#57804=ORIENTED_EDGE ( 'NONE', *, *, #153466, .T. ) ;
#57836=EDGE_CURVE ( 'NONE', #143460, #31770, #50947, .T. ) ;
#57837=DIRECTION ( 'NONE',  ( -1.000000000000000000, 0.000000000000000000, 0.000000000000000000 ) ) ;
#57845=VERTEX_POINT ( 'NONE', #206388 ) ;
#57860=CARTESIAN_POINT ( 'NONE',  ( 20.12500000000000355, 9.258049272917324046, -8.363338837142434201 ) ) ;
#57871=CIRCLE ( 'NONE', #37079, 2.000000000000002665 ) ;
#57876=CIRCLE ( 'NONE', #37084, 0.09999999999999939493 ) ;
#57891=CARTESIAN_POINT ( 'NONE',  ( -20.94999999999999929, 0.000000000000000000, 0.000000000000000000 ) ) ;
#57900=CARTESIAN_POINT ( 'NONE',  ( 21.05000000000000071, 10.72371710470752149, -12.15000000000000036 ) ) ;
#57918=ORIENTED_EDGE ( 'NONE', *, *, #115872, .T. ) ;
#57926=EDGE_LOOP ( 'NONE', ( #112584, #193582, #154192, #345 ) ) ;
#57929=ORIENTED_EDGE ( 'NONE', *, *, #117338, .T. ) ;
#57932=CARTESIAN_POINT ( 'NONE',  ( -23.15000000000000213, 0.000000000000000000, -33.50000000000000000 ) ) ;
#57935=CARTESIAN_POINT ( 'NONE',  ( -23.25000000000000000, 1.999999999999998224, -13.22462192276210224 ) ) ;
#57938=DIRECTION ( 'NONE',  ( -1.000000000000000000, -2.952720810173289112E-16, 0.000000000000000000 ) ) ;
#57940=LINE ( 'NONE', #197463, #254557 ) ;
#57977=LINE ( 'NONE', #137515, #97009 ) ;
#57984=EDGE_LOOP ( 'NONE', ( #213048, #129397, #145971, #150721 ) ) ;
#57990=CARTESIAN_POINT ( 'NONE',  ( 23.14999999999999503, 6.550000000000000711, -21.25000000000000000 ) ) ;
#57992=ADVANCED_FACE ( 'NONE', ( #72023 ), #154161, .T. ) ;
#57997=ORIENTED_EDGE ( 'NONE', *, *, #44138, .F. ) ;
#58037=CARTESIAN_POINT ( 'NONE',  ( 21.05000000000000071, 5.399999999999998579, -21.09473398108690390 ) ) ;
#58051=AXIS2_PLACEMENT_3D ( 'NONE', #13330, #233665, #134530 ) ;
#58089=EDGE_CURVE ( 'NONE', #244818, #226285, #14627, .T. ) ;
#58094=CARTESIAN_POINT ( 'NONE',  ( 18.49999999999999645, 1.835341550224411922, -11.55515129256298046 ) ) ;
#58107=ORIENTED_EDGE ( 'NONE', *, *, #49348, .T. ) ;
#58174=ORIENTED_EDGE ( 'NONE', *, *, #111020, .T. ) ;
#58179=DIRECTION ( 'NONE',  ( 1.000000000000000000, 0.000000000000000000, 0.000000000000000000 ) ) ;
#58188=ORIENTED_EDGE ( 'NONE', *, *, #217165, .T. ) ;
#58194=ORIENTED_EDGE ( 'NONE', *, *, #71457, .F. ) ;
#58202=ORIENTED_EDGE ( 'NONE', *, *, #95806, .T. ) ;
#58204=CYLINDRICAL_SURFACE ( 'NONE', #18759, 0.1000000000000008105 ) ;
#58207=CARTESIAN_POINT ( 'NONE',  ( 20.94999999999999929, 5.399999999999998579, -21.09473398108690390 ) ) ;
#58239=VERTEX_POINT ( 'NONE', #243913 ) ;
#58258=CARTESIAN_POINT ( 'NONE',  ( 20.95512820512820440, 8.876151316288115822, -8.558628995140949769 ) ) ;
#58293=LINE ( 'NONE', #256445, #100876 ) ;
#58296=CARTESIAN_POINT ( 'NONE',  ( -22.50000000000094147, 0.09999999999989445110, 11.64957080754481744 ) ) ;
#58313=CIRCLE ( 'NONE', #154071, 0.1000000000000001305 ) ;
#58337=CARTESIAN_POINT ( 'NONE',  ( 21.05000000000000071, 6.258847123079377184, 0.03175835305537381276 ) ) ;
#58396=DIRECTION ( 'NONE',  ( 1.000000000000000000, 2.952720810173289112E-16, -0.000000000000000000 ) ) ;
#58403=EDGE_CURVE ( 'NONE', #26537, #158092, #249082, .T. ) ;
#58449=CARTESIAN_POINT ( 'NONE',  ( 23.24999999999999289, 6.649999999999999467, -12.35000000000000320 ) ) ;
#58463=CARTESIAN_POINT ( 'NONE',  ( -21.11927991906891222, 0.009083679473871926827, 6.448493118491512632 ) ) ;
#58469=CARTESIAN_POINT ( 'NONE',  ( -20.00857864376270001, 9.350000000000001421, -12.25000000000000000 ) ) ;
#58491=CARTESIAN_POINT ( 'NONE',  ( -18.50000000000000000, -1.835859311443640340, -45.00443916879852679 ) ) ;
#58529=EDGE_CURVE ( 'NONE', #32374, #51098, #119236, .T. ) ;
#58535=ORIENTED_EDGE ( 'NONE', *, *, #167746, .T. ) ;
#58557=CARTESIAN_POINT ( 'NONE',  ( 20.58091095332318332, 9.018470153352529550, -8.418650182158506468 ) ) ;
#58565=ORIENTED_EDGE ( 'NONE', *, *, #128023, .T. ) ;
#58586=FACE_OUTER_BOUND ( 'NONE', #102394, .T. ) ;
#58604=ORIENTED_EDGE ( 'NONE', *, *, #59562, .T. ) ;
#58605=CARTESIAN_POINT ( 'NONE',  ( -21.05000000000000071, 6.540656951701240729, -0.09999999999999939493 ) ) ;
#58612=CARTESIAN_POINT ( 'NONE',  ( 18.56308993302899069, 10.38069115532423581, -24.73922263893877371 ) ) ;
#58616=EDGE_LOOP ( 'NONE', ( #51262, #68377, #39924, #155165 ) ) ;
#58617=DIRECTION ( 'NONE',  ( 1.000000000000000000, 0.000000000000000000, 0.000000000000000000 ) ) ;
#58629=DIRECTION ( 'NONE',  ( 0.000000000000000000, 0.000000000000000000, -1.000000000000000000 ) ) ;
#58685=DIRECTION ( 'NONE',  ( 0.000000000000000000, 0.000000000000000000, -1.000000000000000000 ) ) ;
#58724=CARTESIAN_POINT ( 'NONE',  ( 23.14999999999999503, 11.65000000000000746, -26.58519422934605814 ) ) ;
#58731=DIRECTION ( 'NONE',  ( -1.000000000000000000, -7.304098846218134667E-16, 0.000000000000000000 ) ) ;
#58737=CARTESIAN_POINT ( 'NONE',  ( 20.95566103547454517, 10.61824765094706358, -7.631840192980594573 ) ) ;
#58769=ORIENTED_EDGE ( 'NONE', *, *, #8078, .T. ) ;
#58820=EDGE_CURVE ( 'NONE', #124226, #113211, #160896, .T. ) ;
#58846=VECTOR ( 'NONE', #205411, 1000.000000000000000 ) ;
#58858=VERTEX_POINT ( 'NONE', #20093 ) ;
#58918=CIRCLE ( 'NONE', #212898, 0.09999999999999939493 ) ;
#58922=AXIS2_PLACEMENT_3D ( 'NONE', #178928, #158093, #242 ) ;
#58928=AXIS2_PLACEMENT_3D ( 'NONE', #124313, #103432, #82571 ) ;
#58944=ORIENTED_EDGE ( 'NONE', *, *, #86680, .F. ) ;
#58956=CIRCLE ( 'NONE', #254745, 0.09999999999999982514 ) ;
#58977=CARTESIAN_POINT ( 'NONE',  ( 23.15000000000000213, -8.663551401869154844, -23.97589888193268948 ) ) ;
#59020=VERTEX_POINT ( 'NONE', #202573 ) ;
#59034=CARTESIAN_POINT ( 'NONE',  ( 20.94999999999999929, 0.000000000000000000, 0.000000000000000000 ) ) ;
#59041=FACE_OUTER_BOUND ( 'NONE', #9092, .T. ) ;
#59071=ORIENTED_EDGE ( 'NONE', *, *, #87330, .F. ) ;
#59114=ORIENTED_EDGE ( 'NONE', *, *, #118288, .T. ) ;
#59116=ADVANCED_FACE ( 'NONE', ( #15964 ), #169917, .F. ) ;
#59118=EDGE_LOOP ( 'NONE', ( #104916, #60491, #177355, #208383 ) ) ;
#59157=ORIENTED_EDGE ( 'NONE', *, *, #37427, .F. ) ;
#59179=DIRECTION ( 'NONE',  ( 0.000000000000000000, -0.7899159663865552572, -0.6132151058540507016 ) ) ;
#59208=VECTOR ( 'NONE', #226533, 1000.000000000000000 ) ;
#59219=ORIENTED_EDGE ( 'NONE', *, *, #229025, .T. ) ;
#59235=CARTESIAN_POINT ( 'NONE',  ( 20.85000000000000142, -1.835859311443637010, -45.00443916879852679 ) ) ;
#59243=DIRECTION ( 'NONE',  ( 0.000000000000000000, -0.000000000000000000, -1.000000000000000000 ) ) ;
#59253=EDGE_LOOP ( 'NONE', ( #111021, #244834, #148512, #172121, #33862, #142947 ) ) ;
#59292=CARTESIAN_POINT ( 'NONE',  ( 20.85000000000000142, 0.000000000000000000, -33.50000000000000000 ) ) ;
#59343=CARTESIAN_POINT ( 'NONE',  ( -21.05000000000000071, 5.849999999999949019, -10.13249722427796762 ) ) ;
#59361=ORIENTED_EDGE ( 'NONE', *, *, #183289, .F. ) ;
#59400=LINE ( 'NONE', #138940, #18792 ) ;
#59413=EDGE_CURVE ( 'NONE', #240172, #191070, #74355, .T. ) ;
#59419=VERTEX_POINT ( 'NONE', #153910 ) ;
#59432=DIRECTION ( 'NONE',  ( 0.000000000000000000, 0.000000000000000000, -1.000000000000000000 ) ) ;
#59474=EDGE_CURVE ( 'NONE', #221017, #23701, #213828, .T. ) ;
#59484=VECTOR ( 'NONE', #1370, 1000.000000000000000 ) ;
#59515=DIRECTION ( 'NONE',  ( 0.000000000000000000, 0.000000000000000000, 1.000000000000000000 ) ) ;
#59540=DIRECTION ( 'NONE',  ( 1.000000000000000000, -0.000000000000000000, -0.000000000000000000 ) ) ;
#59546=ADVANCED_FACE ( 'NONE', ( #218953 ), #117300, .F. ) ;
#59562=EDGE_CURVE ( 'NONE', #136985, #17846, #61785, .T. ) ;
#59582=AXIS2_PLACEMENT_3D ( 'NONE', #254164, #235888, #18138 ) ;
#59594=ADVANCED_FACE ( 'NONE', ( #176011 ), #208498, .T. ) ;
#59610=DIRECTION ( 'NONE',  ( -1.000000000000000000, -0.000000000000000000, -0.000000000000000000 ) ) ;
#59650=CARTESIAN_POINT ( 'NONE',  ( 22.45380639572288928, 1.426688889968629469E-07, 11.75043289110677591 ) ) ;
#59651=CARTESIAN_POINT ( 'NONE',  ( 23.14999999999999503, 14.10000000000000142, -27.89970238886063925 ) ) ;
#59653=CYLINDRICAL_SURFACE ( 'NONE', #248519, 0.09999999999999939493 ) ;
#59681=VECTOR ( 'NONE', #240614, 1000.000000000000000 ) ;
#59713=UNCERTAINTY_MEASURE_WITH_UNIT (LENGTH_MEASURE( 1.000000000000000082E-05 ), #192260, 'distance_accuracy_value', 'NONE');
#59744=CARTESIAN_POINT ( 'NONE',  ( -21.09813707148783735, 0.03135149952943332152, 6.385062105736676763 ) ) ;
#59754=AXIS2_PLACEMENT_3D ( 'NONE', #256222, #172955, #115495 ) ;
#59784=CARTESIAN_POINT ( 'NONE',  ( 21.00000000000000000, 9.749999999999998224, -12.35000000000000320 ) ) ;
#59834=CARTESIAN_POINT ( 'NONE',  ( 20.77766267348356166, 10.44904239061880702, -7.592708915877627973 ) ) ;
#59860=DIRECTION ( 'NONE',  ( -1.000000000000000000, 0.000000000000000000, -0.000000000000000000 ) ) ;
#59863=DIRECTION ( 'NONE',  ( 0.000000000000000000, 0.000000000000000000, -1.000000000000000000 ) ) ;
#59867=DIRECTION ( 'NONE',  ( -1.000000000000000000, 0.000000000000000000, 0.000000000000000000 ) ) ;
#59871=ADVANCED_FACE ( 'NONE', ( #12778 ), #200104, .T. ) ;
#59895=ORIENTED_EDGE ( 'NONE', *, *, #217400, .F. ) ;
#59914=EDGE_CURVE ( 'NONE', #145230, #170111, #67008, .T. ) ;
#59922=CARTESIAN_POINT ( 'NONE',  ( -23.15000000000000213, 5.950000000000007283, -23.19429769496518645 ) ) ;
#59955=ORIENTED_EDGE ( 'NONE', *, *, #169932, .T. ) ;
#59964=LINE ( 'NONE', #238629, #125099 ) ;
#59968=ORIENTED_EDGE ( 'NONE', *, *, #161801, .F. ) ;
#59973=DIRECTION ( 'NONE',  ( -1.000000000000000000, 0.000000000000000000, 0.000000000000000000 ) ) ;
#59986=VECTOR ( 'NONE', #37630, 1000.000000000000000 ) ;
#60003=DIRECTION ( 'NONE',  ( 0.000000000000000000, -0.8660254037844383745, 0.5000000000000003331 ) ) ;
#60005=EDGE_CURVE ( 'NONE', #68838, #180003, #150423, .T. ) ;
#60013=ADVANCED_FACE ( 'NONE', ( #187105 ), #46268, .T. ) ;
#60018=EDGE_LOOP ( 'NONE', ( #93564, #76226, #118653, #159220 ) ) ;
#60062=VECTOR ( 'NONE', #7872, 1000.000000000000114 ) ;
#60077=ORIENTED_EDGE ( 'NONE', *, *, #135403, .F. ) ;
#60090=ORIENTED_EDGE ( 'NONE', *, *, #204308, .T. ) ;
#60156=EDGE_LOOP ( 'NONE', ( #1123, #254123, #63713, #20352 ) ) ;
#60204=ORIENTED_EDGE ( 'NONE', *, *, #196952, .F. ) ;
#60278=ORIENTED_EDGE ( 'NONE', *, *, #213156, .T. ) ;
#60316=ORIENTED_EDGE ( 'NONE', *, *, #201474, .F. ) ;
#60321=CARTESIAN_POINT ( 'NONE',  ( -20.94999999999999929, -1.261786168565025568, -8.086498963545480478 ) ) ;
#60343=DIRECTION ( 'NONE',  ( 7.304098846218134667E-16, -1.000000000000000000, 0.000000000000000000 ) ) ;
#60373=ADVANCED_FACE ( 'NONE', ( #122195 ), #102582, .T. ) ;
#60397=ORIENTED_EDGE ( 'NONE', *, *, #166871, .F. ) ;
#60431=CARTESIAN_POINT ( 'NONE',  ( 20.94999999999999929, -1.835859311443637010, -45.00443916879852679 ) ) ;
#60459=( GEOMETRIC_REPRESENTATION_CONTEXT ( 3 ) GLOBAL_UNCERTAINTY_ASSIGNED_CONTEXT ( ( #59713 ) ) GLOBAL_UNIT_ASSIGNED_CONTEXT ( ( #192260, #210525, #190985 ) ) REPRESENTATION_CONTEXT ( 'NONE', 'WORKASPACE' ) );
#60491=ORIENTED_EDGE ( 'NONE', *, *, #73530, .T. ) ;
#60495=ORIENTED_EDGE ( 'NONE', *, *, #125824, .F. ) ;
#60515=VECTOR ( 'NONE', #103268, 1000.000000000000000 ) ;
#60520=EDGE_LOOP ( 'NONE', ( #160965, #250610, #23981, #24978 ) ) ;
#60524=EDGE_CURVE ( 'NONE', #19453, #143109, #229696, .T. ) ;
#60529=AXIS2_PLACEMENT_3D ( 'NONE', #124549, #244476, #205334 ) ;
#60539=CARTESIAN_POINT ( 'NONE',  ( -21.05000000000000071, -11.65000000000000036, -2.900000000000001688 ) ) ;
#60605=CARTESIAN_POINT ( 'NONE',  ( 20.04142135623730070, 11.75000000000000355, -21.35000000000000142 ) ) ;
#60609=DIRECTION ( 'NONE',  ( 0.000000000000000000, 0.000000000000000000, -1.000000000000000000 ) ) ;
#60680=ORIENTED_EDGE ( 'NONE', *, *, #174256, .F. ) ;
#60694=ORIENTED_EDGE ( 'NONE', *, *, #62228, .F. ) ;
#60724=ORIENTED_EDGE ( 'NONE', *, *, #96091, .T. ) ;
#60792=AXIS2_PLACEMENT_3D ( 'NONE', #74319, #91288, #70473 ) ;
#60837=EDGE_CURVE ( 'NONE', #160000, #44809, #180004, .T. ) ;
#60855=EDGE_CURVE ( 'NONE', #31598, #82492, #104921, .T. ) ;
#60882=DIRECTION ( 'NONE',  ( 0.000000000000000000, 0.000000000000000000, -1.000000000000000000 ) ) ;
#60886=CIRCLE ( 'NONE', #198267, 0.09999999999999939493 ) ;
#60896=CIRCLE ( 'NONE', #144264, 0.1999999999999987899 ) ;
#60900=VERTEX_POINT ( 'NONE', #90441 ) ;
#60913=AXIS2_PLACEMENT_3D ( 'NONE', #177530, #116248, #157972 ) ;
#60925=CARTESIAN_POINT ( 'NONE',  ( -23.15000000000000213, -9.000000000000001776, -23.60603087734756045 ) ) ;
#60957=DIRECTION ( 'NONE',  ( -0.000000000000000000, 1.000000000000000000, 0.000000000000000000 ) ) ;
#60971=EDGE_CURVE ( 'NONE', #93175, #109469, #109046, .T. ) ;
#60979=ORIENTED_EDGE ( 'NONE', *, *, #56567, .F. ) ;
#60986=DIRECTION ( 'NONE',  ( 7.304098846218134667E-16, 1.000000000000000000, -0.000000000000000000 ) ) ;
#61026=VERTEX_POINT ( 'NONE', #252094 ) ;
#61051=CARTESIAN_POINT ( 'NONE',  ( -21.29999999999995808, 0.000000000000000000, 0.000000000000000000 ) ) ;
#61064=EDGE_LOOP ( 'NONE', ( #36591, #32545, #91815, #144439 ) ) ;
#61081=DIRECTION ( 'NONE',  ( 0.000000000000000000, 0.000000000000000000, -1.000000000000000000 ) ) ;
#61094=ADVANCED_FACE ( 'NONE', ( #57734 ), #12228, .F. ) ;
#61107=EDGE_CURVE ( 'NONE', #207698, #210716, #213474, .T. ) ;
#61115=LINE ( 'NONE', #98931, #35836 ) ;
#61132=AXIS2_PLACEMENT_3D ( 'NONE', #178495, #97618, #119802 ) ;
#61133=ORIENTED_EDGE ( 'NONE', *, *, #226880, .T. ) ;
#61178=AXIS2_PLACEMENT_3D ( 'NONE', #137172, #34259, #135870 ) ;
#61189=CARTESIAN_POINT ( 'NONE',  ( 23.14999999999999503, 6.450000000000001066, -12.35000000000000320 ) ) ;
#61229=DIRECTION ( 'NONE',  ( -1.000000000000000000, -0.000000000000000000, 0.000000000000000000 ) ) ;
#61281=EDGE_LOOP ( 'NONE', ( #150200, #182342, #66532, #182967 ) ) ;
#61307=EDGE_CURVE ( 'NONE', #6193, #56955, #230051, .T. ) ;
#61340=CARTESIAN_POINT ( 'NONE',  ( 22.01447462590973458, 0.09903700005953483543, 7.263800201229913434 ) ) ;
#61342=VECTOR ( 'NONE', #63471, 1000.000000000000000 ) ;
#61383=CARTESIAN_POINT ( 'NONE',  ( 21.05000000000000071, 0.000000000000000000, -33.50000000000000000 ) ) ;
#61402=ORIENTED_EDGE ( 'NONE', *, *, #122360, .F. ) ;
#61410=DIRECTION ( 'NONE',  ( 0.000000000000000000, 0.6728971962616965286, -0.7397360091702632756 ) ) ;
#61411=DIRECTION ( 'NONE',  ( -0.000000000000000000, -0.000000000000000000, 1.000000000000000000 ) ) ;
#61417=CARTESIAN_POINT ( 'NONE',  ( 20.85000000000000142, -1.135018845910178431, -41.21697688343231647 ) ) ;
#61471=DIRECTION ( 'NONE',  ( -0.000000000000000000, -1.265107689135680095E-16, 1.000000000000000000 ) ) ;
#61476=LINE ( 'NONE', #163155, #89435 ) ;
#61489=DIRECTION ( 'NONE',  ( 0.000000000000000000, -0.000000000000000000, -1.000000000000000000 ) ) ;
#61497=ORIENTED_EDGE ( 'NONE', *, *, #239153, .F. ) ;
#61506=EDGE_CURVE ( 'NONE', #207105, #239230, #200477, .T. ) ;
#61542=CARTESIAN_POINT ( 'NONE',  ( 20.95512820512820795, 10.62384868371188240, -12.20016201942441647 ) ) ;
#61571=EDGE_CURVE ( 'NONE', #187669, #256381, #63513, .T. ) ;
#61572=LINE ( 'NONE', #120301, #251098 ) ;
#61586=ORIENTED_EDGE ( 'NONE', *, *, #137323, .F. ) ;
#61587=CYLINDRICAL_SURFACE ( 'NONE', #249018, 0.09999999999999939493 ) ;
#61588=AXIS2_PLACEMENT_3D ( 'NONE', #158267, #201199, #240342 ) ;
#61607=ORIENTED_EDGE ( 'NONE', *, *, #216542, .T. ) ;
#61614=VERTEX_POINT ( 'NONE', #222576 ) ;
#61664=ORIENTED_EDGE ( 'NONE', *, *, #103433, .F. ) ;
#61671=ORIENTED_EDGE ( 'NONE', *, *, #85258, .F. ) ;
#61704=CARTESIAN_POINT ( 'NONE',  ( -1.820710678118658388, -9.929289321881341834, -24.65000000000000213 ) ) ;
#61718=DIRECTION ( 'NONE',  ( -0.000000000000000000, 0.8660254037844383745, -0.5000000000000003331 ) ) ;
#61763=DIRECTION ( 'NONE',  ( 1.000000000000000000, 0.000000000000000000, -0.000000000000000000 ) ) ;
#61785=B_SPLINE_CURVE_WITH_KNOTS ( 'NONE', 3,
 ( #18196, #139403, #19491, #177306, #78151, #119891 ),
 .UNSPECIFIED., .F., .F.,
 ( 4, 2, 4 ),
 ( 0.000000000000000000, 0.0001891491689349584983, 0.0003782983378699169967 ),
 .UNSPECIFIED. ) ;
#61792=EDGE_CURVE ( 'NONE', #16790, #138899, #195050, .T. ) ;
#61796=CARTESIAN_POINT ( 'NONE',  ( -20.94999999999999929, 0.000000000000000000, 0.000000000000000000 ) ) ;
#61874=AXIS2_PLACEMENT_3D ( 'NONE', #69714, #149254, #206637 ) ;
#61875=CYLINDRICAL_SURFACE ( 'NONE', #88274, 0.09999999999999939493 ) ;
#61919=ORIENTED_EDGE ( 'NONE', *, *, #41500, .F. ) ;
#61921=ADVANCED_FACE ( 'NONE', ( #37260 ), #234145, .T. ) ;
#61939=DIRECTION ( 'NONE',  ( -0.000000000000000000, 0.000000000000000000, 1.000000000000000000 ) ) ;
#61956=DIRECTION ( 'NONE',  ( -1.000000000000000000, 0.000000000000000000, 0.000000000000000000 ) ) ;
#61962=CIRCLE ( 'NONE', #228563, 0.09999999999999961697 ) ;
#61965=ADVANCED_FACE ( 'NONE', ( #3228 ), #41118, .F. ) ;
#61972=AXIS2_PLACEMENT_3D ( 'NONE', #65998, #142944, #222481 ) ;
#62021=DIRECTION ( 'NONE',  ( 1.836970198721029934E-16, -1.000000000000000000, -0.000000000000000000 ) ) ;
#62028=FACE_OUTER_BOUND ( 'NONE', #122574, .T. ) ;
#62053=CARTESIAN_POINT ( 'NONE',  ( 23.14999999999999858, 0.000000000000000000, -33.50000000000000000 ) ) ;
#62072=DIRECTION ( 'NONE',  ( -1.000000000000000000, 0.000000000000000000, 0.000000000000000000 ) ) ;
#62080=ORIENTED_EDGE ( 'NONE', *, *, #87330, .T. ) ;
#62086=EDGE_CURVE ( 'NONE', #234302, #216880, #117989, .T. ) ;
#62100=ORIENTED_EDGE ( 'NONE', *, *, #218095, .T. ) ;
#62113=ORIENTED_EDGE ( 'NONE', *, *, #71554, .T. ) ;
#62135=VERTEX_POINT ( 'NONE', #227429 ) ;
#62144=ORIENTED_EDGE ( 'NONE', *, *, #119255, .T. ) ;
#62179=CARTESIAN_POINT ( 'NONE',  ( -22.45437739390953880, -1.124859753953710850E-15, 11.64957081159447405 ) ) ;
#62185=ORIENTED_EDGE ( 'NONE', *, *, #94363, .T. ) ;
#62211=CIRCLE ( 'NONE', #53831, 0.09999999999999939493 ) ;
#62226=FACE_OUTER_BOUND ( 'NONE', #28031, .T. ) ;
#62228=EDGE_CURVE ( 'NONE', #103673, #136601, #13537, .T. ) ;
#62255=VERTEX_POINT ( 'NONE', #175219 ) ;
#62276=AXIS2_PLACEMENT_3D ( 'NONE', #113467, #58617, #213858 ) ;
#62310=LINE ( 'NONE', #105235, #47692 ) ;
#62328=VERTEX_POINT ( 'NONE', #162046 ) ;
#62345=VERTEX_POINT ( 'NONE', #104586 ) ;
#62350=CIRCLE ( 'NONE', #4082, 4.099999999999999645 ) ;
#62351=DIRECTION ( 'NONE',  ( 0.000000000000000000, 0.000000000000000000, 1.000000000000000000 ) ) ;
#62372=EDGE_LOOP ( 'NONE', ( #139940, #23893, #210272, #124538 ) ) ;
#62378=LINE ( 'NONE', #122353, #90524 ) ;
#62437=DIRECTION ( 'NONE',  ( -0.000000000000000000, 0.000000000000000000, 1.000000000000000000 ) ) ;
#62457=VERTEX_POINT ( 'NONE', #198573 ) ;
#62478=ORIENTED_EDGE ( 'NONE', *, *, #251257, .F. ) ;
#62481=ORIENTED_EDGE ( 'NONE', *, *, #184738, .T. ) ;
#62491=FACE_OUTER_BOUND ( 'NONE', #73950, .T. ) ;
#62537=DIRECTION ( 'NONE',  ( -1.000000000000000000, 0.000000000000000000, 0.000000000000000000 ) ) ;
#62559=FACE_OUTER_BOUND ( 'NONE', #7739, .T. ) ;
#62571=DIRECTION ( 'NONE',  ( 0.000000000000000000, 0.000000000000000000, 1.000000000000000000 ) ) ;
#62579=CARTESIAN_POINT ( 'NONE',  ( 22.57320508075688537, 11.65000000000000036, 0.000000000000000000 ) ) ;
#62585=CIRCLE ( 'NONE', #208343, 0.09999999999999939493 ) ;
#62592=VECTOR ( 'NONE', #227954, 1000.000000000000000 ) ;
#62597=CARTESIAN_POINT ( 'NONE',  ( -21.05000000000000071, 5.900000000000005684, -23.28090023534363340 ) ) ;
#62626=EDGE_CURVE ( 'NONE', #172615, #209763, #244117, .T. ) ;
#62678=DIRECTION ( 'NONE',  ( 1.000000000000000000, -0.000000000000000000, -0.000000000000000000 ) ) ;
#62691=VERTEX_POINT ( 'NONE', #36671 ) ;
#62757=DIRECTION ( 'NONE',  ( 0.000000000000000000, -0.1298341882520022694, -0.9915357197604853789 ) ) ;
#62783=DIRECTION ( 'NONE',  ( -0.7071067811865474617, -0.7071067811865474617, -0.000000000000000000 ) ) ;
#62789=CYLINDRICAL_SURFACE ( 'NONE', #120171, 0.09999999999999939493 ) ;
#62806=DIRECTION ( 'NONE',  ( 0.000000000000000000, 0.000000000000000000, -1.000000000000000000 ) ) ;
#62814=FACE_BOUND ( 'NONE', #9704, .T. ) ;
#62851=DIRECTION ( 'NONE',  ( -0.000000000000000000, -0.000000000000000000, -1.000000000000000000 ) ) ;
#62855=EDGE_CURVE ( 'NONE', #243446, #81993, #163589, .T. ) ;
#62874=DIRECTION ( 'NONE',  ( 0.000000000000000000, 0.000000000000000000, -1.000000000000000000 ) ) ;
#62880=ADVANCED_FACE ( 'NONE', ( #187722 ), #130828, .T. ) ;
#62889=AXIS2_PLACEMENT_3D ( 'NONE', #239295, #144029, #41116 ) ;
#62904=VECTOR ( 'NONE', #232282, 1000.000000000000000 ) ;
#62923=ADVANCED_FACE ( 'NONE', ( #247674 ), #167515, .T. ) ;
#62935=DIRECTION ( 'NONE',  ( -1.000000000000000000, 0.000000000000000000, 0.000000000000000000 ) ) ;
#63006=FACE_OUTER_BOUND ( 'NONE', #72950, .T. ) ;
#63069=VERTEX_POINT ( 'NONE', #176810 ) ;
#63071=CIRCLE ( 'NONE', #196352, 0.09999999999999939493 ) ;
#63110=CARTESIAN_POINT ( 'NONE',  ( -20.64999999999999858, 4.250000000000000000, -21.14999999999999858 ) ) ;
#63122=ORIENTED_EDGE ( 'NONE', *, *, #74646, .F. ) ;
#63148=EDGE_CURVE ( 'NONE', #126038, #250243, #181930, .T. ) ;
#63156=CARTESIAN_POINT ( 'NONE',  ( 21.00000000000000000, 9.749999999999998224, -21.25000000000000000 ) ) ;
#63169=CARTESIAN_POINT ( 'NONE',  ( -21.05000000000000071, 0.000000000000000000, -33.50000000000000000 ) ) ;
#63174=TOROIDAL_SURFACE ( 'NONE', #129813, 0.2000000000000000111, 0.1000000000000000056 ) ;
#63187=CARTESIAN_POINT ( 'NONE',  ( -21.05000000000000071, 0.000000000000000000, 0.000000000000000000 ) ) ;
#63204=CARTESIAN_POINT ( 'NONE',  ( 20.94999999999999574, 14.00000000000000178, -5.427092530382545021 ) ) ;
#63276=CYLINDRICAL_SURFACE ( 'NONE', #38675, 0.1000000000000000472 ) ;
#63284=CARTESIAN_POINT ( 'NONE',  ( 20.94999999999999574, 1.835341550224411922, -11.55515129256298046 ) ) ;
#63292=LINE ( 'NONE', #124574, #98044 ) ;
#63299=ORIENTED_EDGE ( 'NONE', *, *, #41213, .F. ) ;
#63308=CARTESIAN_POINT ( 'NONE',  ( -18.59999999999999787, 11.64999999999999680, -21.25000000000000000 ) ) ;
#63313=CIRCLE ( 'NONE', #104806, 4.049999999999998934 ) ;
#63331=ORIENTED_EDGE ( 'NONE', *, *, #69986, .F. ) ;
#63344=CARTESIAN_POINT ( 'NONE',  ( -20.94999999999999929, 5.204170427930421283E-15, -2.899999999999982592 ) ) ;
#63352=DIRECTION ( 'NONE',  ( 0.000000000000000000, 0.000000000000000000, 1.000000000000000000 ) ) ;
#63368=EDGE_CURVE ( 'NONE', #15628, #207337, #14130, .T. ) ;
#63385=AXIS2_PLACEMENT_3D ( 'NONE', #78370, #96626, #176220 ) ;
#63388=DIRECTION ( 'NONE',  ( 1.000000000000000000, 0.000000000000000000, 0.000000000000000000 ) ) ;
#63428=LINE ( 'NONE', #201662, #25282 ) ;
#63451=CARTESIAN_POINT ( 'NONE',  ( 21.05000000000000071, 5.900000000000005684, -23.28090023534362629 ) ) ;
#63471=DIRECTION ( 'NONE',  ( -0.000000000000000000, -0.000000000000000000, 1.000000000000000000 ) ) ;
#63472=CARTESIAN_POINT ( 'NONE',  ( -21.52071067811865746, 7.779289321881349473, -21.25000000000000000 ) ) ;
#63478=CARTESIAN_POINT ( 'NONE',  ( -21.44999999999999929, 7.249999999999999112, -12.34999999999999964 ) ) ;
#63488=VERTEX_POINT ( 'NONE', #138607 ) ;
#63489=DIRECTION ( 'NONE',  ( 0.000000000000000000, 0.000000000000000000, -1.000000000000000000 ) ) ;
#63492=DIRECTION ( 'NONE',  ( 1.000000000000000000, 0.000000000000000000, 0.000000000000000000 ) ) ;
#63511=CARTESIAN_POINT ( 'NONE',  ( 23.24999999999999645, -3.899999999999999467, -33.50000000000000000 ) ) ;
#63513=LINE ( 'NONE', #103908, #246971 ) ;
#63519=DIRECTION ( 'NONE',  ( 1.000000000000000000, 0.000000000000000000, 0.000000000000000000 ) ) ;
#63523=EDGE_CURVE ( 'NONE', #103673, #167893, #222173, .T. ) ;
#63525=CARTESIAN_POINT ( 'NONE',  ( -20.05000000000000426, 9.250000000000001776, -21.25000000000000000 ) ) ;
#63536=AXIS2_PLACEMENT_3D ( 'NONE', #148225, #32160, #92099 ) ;
#63553=CARTESIAN_POINT ( 'NONE',  ( -20.95000000000000284, 11.74999999999999822, -6.841600689897113341 ) ) ;
#63586=CARTESIAN_POINT ( 'NONE',  ( -21.05000000000000071, -11.48912529307605901, -3.000000000000002665 ) ) ;
#63602=AXIS2_PLACEMENT_3D ( 'NONE', #217012, #97032, #114063 ) ;
#63617=CARTESIAN_POINT ( 'NONE',  ( -23.25000000000000000, 0.000000000000000000, -41.40000000000000568 ) ) ;
#63665=DIRECTION ( 'NONE',  ( 0.000000000000000000, 0.000000000000000000, -1.000000000000000000 ) ) ;
#63688=CARTESIAN_POINT ( 'NONE',  ( -20.00857864376270001, 9.150000000000002132, -12.34999999999999964 ) ) ;
#63689=ORIENTED_EDGE ( 'NONE', *, *, #4608, .F. ) ;
#63690=AXIS2_PLACEMENT_3D ( 'NONE', #78831, #59243, #123130 ) ;
#63693=VERTEX_POINT ( 'NONE', #210188 ) ;
#63694=ORIENTED_EDGE ( 'NONE', *, *, #71554, .F. ) ;
#63696=ORIENTED_EDGE ( 'NONE', *, *, #29942, .F. ) ;
#63713=ORIENTED_EDGE ( 'NONE', *, *, #237164, .F. ) ;
#63787=CIRCLE ( 'NONE', #76245, 0.2000000000000005107 ) ;
#63796=AXIS2_PLACEMENT_3D ( 'NONE', #121937, #43680, #197601 ) ;
#63806=EDGE_CURVE ( 'NONE', #24262, #67636, #93382, .T. ) ;
#63827=ORIENTED_EDGE ( 'NONE', *, *, #85094, .F. ) ;
#63832=TOROIDAL_SURFACE ( 'NONE', #138792, 0.9750000000000019762, 0.1000000000000000056 ) ;
#63835=ORIENTED_EDGE ( 'NONE', *, *, #142696, .F. ) ;
#63874=ADVANCED_FACE ( 'NONE', ( #137056 ), #30886, .F. ) ;
#63879=CARTESIAN_POINT ( 'NONE',  ( 22.39999999999999503, 0.09999999999999939493, 7.790779598373383408 ) ) ;
#63914=CARTESIAN_POINT ( 'NONE',  ( 21.05000000000000071, 0.000000000000000000, 0.000000000000000000 ) ) ;
#63920=CARTESIAN_POINT ( 'NONE',  ( 21.14999999999999503, 11.65000000000000746, -3.469446951953614189E-15 ) ) ;
#63943=ORIENTED_EDGE ( 'NONE', *, *, #16437, .F. ) ;
#63983=VERTEX_POINT ( 'NONE', #160211 ) ;
#63987=CARTESIAN_POINT ( 'NONE',  ( -21.05000000000000071, 0.000000000000000000, 0.000000000000000000 ) ) ;
#64022=DIRECTION ( 'NONE',  ( 0.000000000000000000, 0.000000000000000000, 1.000000000000000000 ) ) ;
#64042=CARTESIAN_POINT ( 'NONE',  ( -20.64999999999999858, 0.000000000000000000, -33.50000000000000000 ) ) ;
#64054=AXIS2_PLACEMENT_3D ( 'NONE', #149219, #173949, #108780 ) ;
#64060=CIRCLE ( 'NONE', #5774, 11.70000000000000462 ) ;
#64063=EDGE_LOOP ( 'NONE', ( #132994, #29485, #171768, #6828 ) ) ;
#64066=TOROIDAL_SURFACE ( 'NONE', #139038, 0.4000000000000012990, 0.1000000000000000056 ) ;
#64071=ADVANCED_FACE ( 'NONE', ( #186168 ), #194169, .F. ) ;
#64077=CARTESIAN_POINT ( 'NONE',  ( 21.08479644141223019, 0.05855444256413740861, 6.345038657731894460 ) ) ;
#64085=DIRECTION ( 'NONE',  ( -1.000000000000000000, -0.000000000000000000, -0.000000000000000000 ) ) ;
#64117=CARTESIAN_POINT ( 'NONE',  ( 23.14999999999999858, 0.000000000000000000, -33.50000000000000000 ) ) ;
#64118=ORIENTED_EDGE ( 'NONE', *, *, #47518, .F. ) ;
#64284=ORIENTED_EDGE ( 'NONE', *, *, #117240, .F. ) ;
#64295=EDGE_LOOP ( 'NONE', ( #65272, #193046, #69437, #229636 ) ) ;
#64349=LINE ( 'NONE', #202569, #229056 ) ;
#64359=CARTESIAN_POINT ( 'NONE',  ( -18.55807992284872299, 10.32898536000685574, -39.08266832227644016 ) ) ;
#64368=ORIENTED_EDGE ( 'NONE', *, *, #158656, .T. ) ;
#64369=CARTESIAN_POINT ( 'NONE',  ( -20.85000000000000142, 11.74999999999999645, -26.71613433702190576 ) ) ;
#64384=AXIS2_PLACEMENT_3D ( 'NONE', #76939, #95225, #114791 ) ;
#64390=CARTESIAN_POINT ( 'NONE',  ( 18.59999999999999076, -1.164121893241208960, -41.41484808557160591 ) ) ;
#64430=CARTESIAN_POINT ( 'NONE',  ( -23.15000000000000213, -11.48912529307605546, -30.39999999999999858 ) ) ;
#64464=VERTEX_POINT ( 'NONE', #124604 ) ;
#64501=AXIS2_PLACEMENT_3D ( 'NONE', #185276, #187863, #90013 ) ;
#64511=DIRECTION ( 'NONE',  ( 0.000000000000000000, -0.8660254037844411501, -0.4999999999999956146 ) ) ;
#64538=EDGE_CURVE ( 'NONE', #233908, #141418, #118727, .T. ) ;
#64554=CARTESIAN_POINT ( 'NONE',  ( 20.94999999999999574, 14.00000000000000178, -5.427092530382545021 ) ) ;
#64556=DIRECTION ( 'NONE',  ( 0.000000000000000000, -1.000000000000000000, 0.000000000000000000 ) ) ;
#64562=ORIENTED_EDGE ( 'NONE', *, *, #18937, .F. ) ;
#64622=ORIENTED_EDGE ( 'NONE', *, *, #169215, .F. ) ;
#64655=ORIENTED_EDGE ( 'NONE', *, *, #147470, .T. ) ;
#64664=AXIS2_PLACEMENT_3D ( 'NONE', #80491, #160092, #239614 ) ;
#64673=DIRECTION ( 'NONE',  ( 0.000000000000000000, 0.000000000000000000, -1.000000000000000000 ) ) ;
#64715=CARTESIAN_POINT ( 'NONE',  ( -20.94999999999999929, 10.29270135740183179, -38.95736188715193293 ) ) ;
#64740=CARTESIAN_POINT ( 'NONE',  ( -23.25000000000000000, 5.950000000000007283, -23.19429769496518645 ) ) ;
#64763=DIRECTION ( 'NONE',  ( 0.000000000000000000, 0.008583690987124399305, -0.9999631594459055250 ) ) ;
#64775=ORIENTED_EDGE ( 'NONE', *, *, #19986, .T. ) ;
#64776=DIRECTION ( 'NONE',  ( 0.000000000000000000, 0.000000000000000000, -1.000000000000000000 ) ) ;
#64817=DIRECTION ( 'NONE',  ( -1.000000000000000000, -0.000000000000000000, -0.000000000000000000 ) ) ;
#64836=DIRECTION ( 'NONE',  ( 0.000000000000000000, -1.000000000000000000, 0.000000000000000000 ) ) ;
#64846=ORIENTED_EDGE ( 'NONE', *, *, #233901, .F. ) ;
#64854=AXIS2_PLACEMENT_3D ( 'NONE', #31261, #149903, #173348 ) ;
#64859=CARTESIAN_POINT ( 'NONE',  ( -20.85000000000000142, -1.835859311443637010, -45.00443916879852679 ) ) ;
#64873=DIRECTION ( 'NONE',  ( 2.952720810173289112E-16, -1.000000000000000000, 0.000000000000000000 ) ) ;
#64920=EDGE_CURVE ( 'NONE', #43421, #129336, #106388, .T. ) ;
#64958=ORIENTED_EDGE ( 'NONE', *, *, #198164, .T. ) ;
#64962=DIRECTION ( 'NONE',  ( -0.000000000000000000, -1.000000000000000000, -0.000000000000000000 ) ) ;
#64985=FACE_OUTER_BOUND ( 'NONE', #200829, .T. ) ;
#64987=AXIS2_PLACEMENT_3D ( 'NONE', #74465, #40475, #62571 ) ;
#65017=EDGE_LOOP ( 'NONE', ( #183775, #201367, #129924, #108224 ) ) ;
#65040=DIRECTION ( 'NONE',  ( 0.000000000000000000, -0.8700118002898322711, 0.4930308989875231140 ) ) ;
#65042=VECTOR ( 'NONE', #239335, 1000.000000000000000 ) ;
#65053=ORIENTED_EDGE ( 'NONE', *, *, #199289, .T. ) ;
#65075=DIRECTION ( 'NONE',  ( -0.000000000000000000, 0.000000000000000000, 1.000000000000000000 ) ) ;
#65078=CARTESIAN_POINT ( 'NONE',  ( 21.53752568617668572, 6.786807874503922200, 0.09897446126639813935 ) ) ;
#65083=DIRECTION ( 'NONE',  ( 0.000000000000000000, -1.000000000000000000, 0.000000000000000000 ) ) ;
#65108=ORIENTED_EDGE ( 'NONE', *, *, #172978, .F. ) ;
#65118=DIRECTION ( 'NONE',  ( 0.000000000000000000, 0.000000000000000000, -1.000000000000000000 ) ) ;
#65150=DIRECTION ( 'NONE',  ( 0.000000000000000000, -0.000000000000000000, -1.000000000000000000 ) ) ;
#65181=CARTESIAN_POINT ( 'NONE',  ( 21.40925344232283223, 0.09895018861964713364, 6.658518859390456512 ) ) ;
#65192=EDGE_CURVE ( 'NONE', #31598, #165206, #225307, .T. ) ;
#65214=ORIENTED_EDGE ( 'NONE', *, *, #198580, .T. ) ;
#65235=EDGE_LOOP ( 'NONE', ( #231858, #48498 ) ) ;
#65265=VERTEX_POINT ( 'NONE', #250033 ) ;
#65272=ORIENTED_EDGE ( 'NONE', *, *, #131224, .F. ) ;
#65274=CARTESIAN_POINT ( 'NONE',  ( -18.59999999999999787, -1.164121893241208960, -41.21484808557161017 ) ) ;
#65290=AXIS2_PLACEMENT_3D ( 'NONE', #84201, #196830, #56011 ) ;
#65304=ORIENTED_EDGE ( 'NONE', *, *, #81759, .T. ) ;
#65319=AXIS2_PLACEMENT_3D ( 'NONE', #21131, #96752, #176346 ) ;
#65407=ORIENTED_EDGE ( 'NONE', *, *, #8759, .T. ) ;
#65422=CIRCLE ( 'NONE', #44212, 0.09999999999999939493 ) ;
#65423=FACE_OUTER_BOUND ( 'NONE', #218544, .T. ) ;
#65438=CARTESIAN_POINT ( 'NONE',  ( -20.64999999999999858, 7.249999999999999112, -12.34999999999999964 ) ) ;
#65474=ADVANCED_FACE ( 'NONE', ( #75276 ), #189807, .T. ) ;
#65481=DIRECTION ( 'NONE',  ( 0.000000000000000000, -1.734723475976810250E-14, 1.000000000000000000 ) ) ;
#65483=CARTESIAN_POINT ( 'NONE',  ( -23.25000000000000000, -1.736705739467587772, -45.01742258762372728 ) ) ;
#65494=DIRECTION ( 'NONE',  ( 0.000000000000000000, 0.000000000000000000, -1.000000000000000000 ) ) ;
#65496=EDGE_CURVE ( 'NONE', #137417, #206232, #48341, .T. ) ;
#65535=ORIENTED_EDGE ( 'NONE', *, *, #146696, .F. ) ;
#65547=EDGE_LOOP ( 'NONE', ( #24883, #179477, #172032 ) ) ;
#65548=ADVANCED_FACE ( 'NONE', ( #125910 ), #165039, .T. ) ;
#65557=CARTESIAN_POINT ( 'NONE',  ( -23.15000000000000213, 1.999999999999998224, -13.22462192276210224 ) ) ;
#65594=CIRCLE ( 'NONE', #207071, 0.09999999999999939493 ) ;
#65609=CARTESIAN_POINT ( 'NONE',  ( -18.59999999999999787, -1.162701749938009677, -8.099999999999999645 ) ) ;
#65643=VECTOR ( 'NONE', #84602, 1000.000000000000000 ) ;
#65671=DIRECTION ( 'NONE',  ( 0.000000000000000000, -0.000000000000000000, -1.000000000000000000 ) ) ;
#65674=VECTOR ( 'NONE', #53984, 1000.000000000000000 ) ;
#65701=DIRECTION ( 'NONE',  ( -0.7071067811865475727, -0.7071067811865475727, 0.000000000000000000 ) ) ;
#65760=AXIS2_PLACEMENT_3D ( 'NONE', #192093, #113815, #94247 ) ;
#65770=B_SPLINE_CURVE_WITH_KNOTS ( 'NONE', 3,
 ( #15442, #250189, #94947, #234459, #55793, #135354, #115810, #110673 ),
 .UNSPECIFIED., .F., .F.,
 ( 4, 2, 2, 4 ),
 ( 0.000000000000000000, 9.550056980124818076E-05, 0.0001910011396024963615, 0.0003820022792049927230 ),
 .UNSPECIFIED. ) ;
#65774=CIRCLE ( 'NONE', #211530, 11.80000000000000249 ) ;
#65795=EDGE_LOOP ( 'NONE', ( #72544, #225921, #130422, #130242 ) ) ;
#65832=EDGE_CURVE ( 'NONE', #59020, #40483, #127637, .T. ) ;
#65858=DIRECTION ( 'NONE',  ( 0.000000000000000000, 0.000000000000000000, -1.000000000000000000 ) ) ;
#65882=EDGE_CURVE ( 'NONE', #128006, #85343, #173659, .T. ) ;
#65890=DIRECTION ( 'NONE',  ( 0.000000000000000000, 0.000000000000000000, 1.000000000000000000 ) ) ;
#65895=ADVANCED_FACE ( 'NONE', ( #34548 ), #36259, .F. ) ;
#65909=EDGE_CURVE ( 'NONE', #33536, #53603, #152788, .T. ) ;
#65937=ADVANCED_FACE ( 'NONE', ( #242986 ), #255792, .T. ) ;
#65943=ADVANCED_FACE ( 'NONE', ( #42237 ), #186072, .F. ) ;
#65964=CYLINDRICAL_SURFACE ( 'NONE', #12915, 0.09999999999999999167 ) ;
#65971=FACE_OUTER_BOUND ( 'NONE', #210500, .T. ) ;
#65974=ORIENTED_EDGE ( 'NONE', *, *, #77540, .F. ) ;
#65993=ORIENTED_EDGE ( 'NONE', *, *, #52388, .F. ) ;
#65998=CARTESIAN_POINT ( 'NONE',  ( 18.59999999999999787, -1.835341550224411922, -11.55515129256297868 ) ) ;
#66000=CARTESIAN_POINT ( 'NONE',  ( -23.15000000000000213, -9.500000000000001776, -23.60603087734756045 ) ) ;
#66010=CARTESIAN_POINT ( 'NONE',  ( 20.94999999999999929, 11.65000000000000391, -33.50000000000000000 ) ) ;
#66015=DIRECTION ( 'NONE',  ( 0.000000000000000000, -1.000000000000000000, 0.000000000000000000 ) ) ;
#66041=AXIS2_PLACEMENT_3D ( 'NONE', #54370, #234284, #50500 ) ;
#66043=DIRECTION ( 'NONE',  ( 0.000000000000000000, 0.008583690987127922528, 0.9999631594459055250 ) ) ;
#66055=FACE_OUTER_BOUND ( 'NONE', #130165, .T. ) ;
#66121=ORIENTED_EDGE ( 'NONE', *, *, #223024, .F. ) ;
#66133=AXIS2_PLACEMENT_3D ( 'NONE', #121222, #181172, #42933 ) ;
#66150=CARTESIAN_POINT ( 'NONE',  ( 18.59999999999999432, -1.261786168565025568, -8.086498963545480478 ) ) ;
#66151=EDGE_CURVE ( 'NONE', #119315, #188675, #48686, .T. ) ;
#66156=CIRCLE ( 'NONE', #219701, 0.1000000000000002554 ) ;
#66164=EDGE_LOOP ( 'NONE', ( #148657, #157346, #162899, #132254 ) ) ;
#66174=DIRECTION ( 'NONE',  ( 1.000000000000000000, 0.000000000000000000, 0.000000000000000000 ) ) ;
#66178=TOROIDAL_SURFACE ( 'NONE', #99298, 7.800000000000000711, 0.1000000000000000056 ) ;
#66181=FACE_OUTER_BOUND ( 'NONE', #107917, .T. ) ;
#66190=CARTESIAN_POINT ( 'NONE',  ( -18.50000000000000000, 11.74999999999999645, 11.75000000000000000 ) ) ;
#66199=CIRCLE ( 'NONE', #174593, 4.049999999999998934 ) ;
#66206=DIRECTION ( 'NONE',  ( 0.000000000000000000, -0.1350103645451904977, 0.9908441862701596881 ) ) ;
#66212=CARTESIAN_POINT ( 'NONE',  ( -20.94999999999999929, -11.65000000000000036, -30.50000000000000000 ) ) ;
#66234=EDGE_LOOP ( 'NONE', ( #121017, #77709, #43672, #170820 ) ) ;
#66240=CARTESIAN_POINT ( 'NONE',  ( 20.94999999999999929, -8.663551401869158397, -9.524101118067305194 ) ) ;
#66246=CARTESIAN_POINT ( 'NONE',  ( -23.15000000000000213, -8.596261682242992919, -9.450127517150276546 ) ) ;
#66297=CARTESIAN_POINT ( 'NONE',  ( 20.94999999999999929, -11.48912529307605546, -30.39999999999999503 ) ) ;
#66324=DIRECTION ( 'NONE',  ( 1.000000000000000000, -0.000000000000000000, -0.000000000000000000 ) ) ;
#66355=DIRECTION ( 'NONE',  ( 0.000000000000000000, 0.000000000000000000, -1.000000000000000000 ) ) ;
#66375=CIRCLE ( 'NONE', #212127, 2.000000000000001776 ) ;
#66379=ORIENTED_EDGE ( 'NONE', *, *, #59413, .T. ) ;
#66423=CARTESIAN_POINT ( 'NONE',  ( 21.87500000000000355, 9.749999999999998224, -21.15000000000000213 ) ) ;
#66424=EDGE_CURVE ( 'NONE', #56194, #4734, #83267, .T. ) ;
#66474=ORIENTED_EDGE ( 'NONE', *, *, #34723, .F. ) ;
#66480=CARTESIAN_POINT ( 'NONE',  ( 20.95512820512820440, 10.62384868371188062, -12.15000000000000036 ) ) ;
#66484=VERTEX_POINT ( 'NONE', #251347 ) ;
#66486=ADVANCED_FACE ( 'NONE', ( #93565 ), #169298, .T. ) ;
#66497=CARTESIAN_POINT ( 'NONE',  ( -23.25000000000000000, -8.596261682242992919, -9.450127517150276546 ) ) ;
#66503=EDGE_CURVE ( 'NONE', #208882, #243771, #15601, .T. ) ;
#66521=LINE ( 'NONE', #186468, #163762 ) ;
#66531=DIRECTION ( 'NONE',  ( 2.952720810173289112E-16, -1.000000000000000000, -0.000000000000000000 ) ) ;
#66532=ORIENTED_EDGE ( 'NONE', *, *, #122360, .T. ) ;
#66535=DIRECTION ( 'NONE',  ( -1.000000000000000000, 0.000000000000000000, 0.000000000000000000 ) ) ;
#66593=ORIENTED_EDGE ( 'NONE', *, *, #207887, .F. ) ;
#66605=ORIENTED_EDGE ( 'NONE', *, *, #218740, .F. ) ;
#66607=CARTESIAN_POINT ( 'NONE',  ( 18.39999999999999858, -9.499999999999998224, -7.032069396699667685 ) ) ;
#66631=VECTOR ( 'NONE', #68245, 1000.000000000000000 ) ;
#66670=ORIENTED_EDGE ( 'NONE', *, *, #186160, .T. ) ;
#66673=AXIS2_PLACEMENT_3D ( 'NONE', #163332, #65494, #105886 ) ;
#66705=ORIENTED_EDGE ( 'NONE', *, *, #73190, .F. ) ;
#66714=ORIENTED_EDGE ( 'NONE', *, *, #150204, .F. ) ;
#66730=EDGE_CURVE ( 'NONE', #70460, #180003, #240786, .T. ) ;
#66734=ORIENTED_EDGE ( 'NONE', *, *, #103433, .T. ) ;
#66748=AXIS2_PLACEMENT_3D ( 'NONE', #96820, #117697, #36922 ) ;
#66755=FACE_OUTER_BOUND ( 'NONE', #169831, .T. ) ;
#66827=TOROIDAL_SURFACE ( 'NONE', #21066, 11.65000000000000036, 0.1000000000000000056 ) ;
#66831=FACE_OUTER_BOUND ( 'NONE', #248803, .T. ) ;
#66875=CARTESIAN_POINT ( 'NONE',  ( 23.14999999999999503, 11.65000000000000746, -12.15000000000000036 ) ) ;
#66877=CARTESIAN_POINT ( 'NONE',  ( 20.94999999999999929, 6.550000000000000711, -10.01702717044001822 ) ) ;
#66879=AXIS2_PLACEMENT_3D ( 'NONE', #1157, #241099, #2449 ) ;
#66936=DIRECTION ( 'NONE',  ( 0.000000000000000000, -0.000000000000000000, 1.000000000000000000 ) ) ;
#66947=CARTESIAN_POINT ( 'NONE',  ( 20.96077737575330957, 11.62390063400469487, -26.64079195710655412 ) ) ;
#66968=VERTEX_POINT ( 'NONE', #137495 ) ;
#66982=DIRECTION ( 'NONE',  ( 0.000000000000000000, 0.000000000000000000, -1.000000000000000000 ) ) ;
#67008=CIRCLE ( 'NONE', #212765, 0.1000000000000028644 ) ;
#67019=AXIS2_PLACEMENT_3D ( 'NONE', #148323, #68791, #227853 ) ;
#67036=ADVANCED_FACE ( 'NONE', ( #82641 ), #205173, .T. ) ;
#67055=DIRECTION ( 'NONE',  ( 0.000000000000000000, 0.000000000000000000, -1.000000000000000000 ) ) ;
#67105=ORIENTED_EDGE ( 'NONE', *, *, #129606, .F. ) ;
#67130=CARTESIAN_POINT ( 'NONE',  ( 20.94999999999999929, -1.835341550224413698, -11.55515129256298046 ) ) ;
#67134=DIRECTION ( 'NONE',  ( 1.000000000000000000, -0.000000000000000000, -0.000000000000000000 ) ) ;
#67140=EDGE_CURVE ( 'NONE', #230477, #52139, #232441, .T. ) ;
#67142=VERTEX_POINT ( 'NONE', #48677 ) ;
#67148=ORIENTED_EDGE ( 'NONE', *, *, #82177, .F. ) ;
#67151=DIRECTION ( 'NONE',  ( 0.000000000000000000, 0.000000000000000000, -1.000000000000000000 ) ) ;
#67168=AXIS2_PLACEMENT_3D ( 'NONE', #73749, #132420, #93277 ) ;
#67189=ORIENTED_EDGE ( 'NONE', *, *, #120101, .F. ) ;
#67200=ORIENTED_EDGE ( 'NONE', *, *, #18480, .T. ) ;
#67209=FACE_OUTER_BOUND ( 'NONE', #228482, .T. ) ;
#67220=DIRECTION ( 'NONE',  ( -1.000000000000000000, 0.000000000000000000, 0.000000000000000000 ) ) ;
#67228=CARTESIAN_POINT ( 'NONE',  ( -23.15000000000000213, 1.999999999999998224, -20.27537807723789953 ) ) ;
#67236=DIRECTION ( 'NONE',  ( 0.000000000000000000, -0.1350103645451876666, -0.9908441862701600211 ) ) ;
#67251=CARTESIAN_POINT ( 'NONE',  ( -20.94999999999999929, 11.59999999999999964, -26.57179676972449656 ) ) ;
#67270=EDGE_CURVE ( 'NONE', #185478, #158940, #102828, .T. ) ;
#67287=CARTESIAN_POINT ( 'NONE',  ( 20.92356734117541706, 10.31973158070286622, -39.05053347133544150 ) ) ;
#67294=CARTESIAN_POINT ( 'NONE',  ( 21.06086055315977390, 8.774707514956258336, -12.20232215515397023 ) ) ;
#67300=CARTESIAN_POINT ( 'NONE',  ( -20.85000000000000142, 11.74999999999999645, -26.71613433702190576 ) ) ;
#67307=FACE_OUTER_BOUND ( 'NONE', #87037, .T. ) ;
#67326=AXIS2_PLACEMENT_3D ( 'NONE', #55708, #173187, #117014 ) ;
#67334=B_SPLINE_CURVE_WITH_KNOTS ( 'NONE', 3,
 ( #19914, #21214, #182851, #103260, #238957, #121600, #179012, #237665 ),
 .UNSPECIFIED., .F., .F.,
 ( 4, 2, 2, 4 ),
 ( 0.000000000000000000, 0.0002114466876442075882, 0.0003171700314663105421, 0.0004228933752884134960 ),
 .UNSPECIFIED. ) ;
#67369=AXIS2_PLACEMENT_3D ( 'NONE', #28249, #149469, #227688 ) ;
#67374=CARTESIAN_POINT ( 'NONE',  ( 21.05000000000000426, 0.09843750000031840919, 6.299230910092287417 ) ) ;
#67378=DIRECTION ( 'NONE',  ( 0.000000000000000000, 0.000000000000000000, -1.000000000000000000 ) ) ;
#67391=TOROIDAL_SURFACE ( 'NONE', #13244, 0.4000000000000012990, 0.1000000000000000056 ) ;
#67410=ADVANCED_FACE ( 'NONE', ( #10266 ), #11555, .F. ) ;
#67441=ADVANCED_FACE ( 'NONE', ( #211027 ), #159152, .T. ) ;
#67461=CARTESIAN_POINT ( 'NONE',  ( -23.25000000000000000, 2.571758278209444422E-16, -31.39999999999999858 ) ) ;
#67476=EDGE_CURVE ( 'NONE', #174560, #109031, #257459, .T. ) ;
#67507=CYLINDRICAL_SURFACE ( 'NONE', #242845, 0.09999999999999939493 ) ;
#67510=ORIENTED_EDGE ( 'NONE', *, *, #124153, .F. ) ;
#67558=CARTESIAN_POINT ( 'NONE',  ( 21.14999999999999503, -11.74999999999999112, 11.75000000000000000 ) ) ;
#67614=VERTEX_POINT ( 'NONE', #249534 ) ;
#67636=VERTEX_POINT ( 'NONE', #125712 ) ;
#67672=AXIS2_PLACEMENT_3D ( 'NONE', #138987, #17773, #178179 ) ;
#67675=ORIENTED_EDGE ( 'NONE', *, *, #84155, .F. ) ;
#67685=DIRECTION ( 'NONE',  ( 0.7071067811865475727, 0.7071067811865475727, 2.044391222244500083E-16 ) ) ;
#67686=CARTESIAN_POINT ( 'NONE',  ( -21.05000000000000071, -9.519327731092440459, -6.972976376559336664 ) ) ;
#67700=ORIENTED_EDGE ( 'NONE', *, *, #84634, .T. ) ;
#67723=AXIS2_PLACEMENT_3D ( 'NONE', #203452, #103040, #143465 ) ;
#67736=B_SPLINE_CURVE_WITH_KNOTS ( 'NONE', 3,
 ( #92736, #210143, #34102, #154061, #193147, #112327, #111029, #191882 ),
 .UNSPECIFIED., .F., .F.,
 ( 4, 2, 2, 4 ),
 ( 0.000000000000000000, 6.534141206311569483E-05, 0.0001306828241262313897, 0.0002613656482524659235 ),
 .UNSPECIFIED. ) ;
#67787=DIRECTION ( 'NONE',  ( 0.000000000000000000, 0.000000000000000000, -1.000000000000000000 ) ) ;
#67809=AXIS2_PLACEMENT_3D ( 'NONE', #247358, #251201, #127425 ) ;
#67815=ORIENTED_EDGE ( 'NONE', *, *, #250059, .F. ) ;
#67831=AXIS2_PLACEMENT_3D ( 'NONE', #125397, #244038, #240218 ) ;
#67837=EDGE_CURVE ( 'NONE', #195886, #12754, #69731, .T. ) ;
#67856=CIRCLE ( 'NONE', #209495, 11.80000000000000426 ) ;
#67874=CARTESIAN_POINT ( 'NONE',  ( -21.05000000000000071, -0.01465611851314312965, 6.496686585767865729 ) ) ;
#67897=DIRECTION ( 'NONE',  ( -0.000000000000000000, 1.000000000000000000, -0.000000000000000000 ) ) ;
#67907=VECTOR ( 'NONE', #225235, 1000.000000000000227 ) ;
#67911=EDGE_CURVE ( 'NONE', #85343, #192073, #67334, .T. ) ;
#67925=CARTESIAN_POINT ( 'NONE',  ( -23.15000000000000213, 4.776122516674676300E-16, -29.60000000000000142 ) ) ;
#67952=DIRECTION ( 'NONE',  ( -1.000000000000000000, -2.952720810173289112E-16, 0.000000000000000000 ) ) ;
#67962=DIRECTION ( 'NONE',  ( 2.952720810173289112E-16, -1.000000000000000000, 0.000000000000000000 ) ) ;
#67995=CIRCLE ( 'NONE', #30601, 11.65000000000000036 ) ;
#68048=AXIS2_PLACEMENT_3D ( 'NONE', #21327, #137378, #116551 ) ;
#68065=CIRCLE ( 'NONE', #197248, 12.97499999999999787 ) ;
#68071=SPHERICAL_SURFACE ( 'NONE', #111663, 0.1000000000000000056 ) ;
#68086=ORIENTED_EDGE ( 'NONE', *, *, #27868, .F. ) ;
#68154=CARTESIAN_POINT ( 'NONE',  ( -21.45000000000000284, 7.708578643762696636, -12.34999999999999964 ) ) ;
#68185=ORIENTED_EDGE ( 'NONE', *, *, #230207, .T. ) ;
#68187=DIRECTION ( 'NONE',  ( 0.000000000000000000, 0.1575844902526769009, 0.9875055080513748251 ) ) ;
#68242=CARTESIAN_POINT ( 'NONE',  ( 20.85000000000000142, -1.736705739467587772, -45.01742258762372728 ) ) ;
#68245=DIRECTION ( 'NONE',  ( -0.000000000000000000, -0.000000000000000000, 1.000000000000000000 ) ) ;
#68319=VERTEX_POINT ( 'NONE', #200798 ) ;
#68326=DIRECTION ( 'NONE',  ( -1.000000000000000000, -0.000000000000000000, -0.000000000000000000 ) ) ;
#68331=CARTESIAN_POINT ( 'NONE',  ( 21.14999999999999858, 11.65000000000000746, -12.15000000000000036 ) ) ;
#68333=LINE ( 'NONE', #212658, #29268 ) ;
#68365=FACE_OUTER_BOUND ( 'NONE', #143521, .T. ) ;
#68377=ORIENTED_EDGE ( 'NONE', *, *, #23368, .T. ) ;
#68465=ORIENTED_EDGE ( 'NONE', *, *, #42190, .F. ) ;
#68468=CYLINDRICAL_SURFACE ( 'NONE', #27702, 0.5000000000000022204 ) ;
#68538=VERTEX_POINT ( 'NONE', #234463 ) ;
#68546=FACE_OUTER_BOUND ( 'NONE', #93940, .T. ) ;
#68566=AXIS2_PLACEMENT_3D ( 'NONE', #95966, #252473, #254987 ) ;
#68572=CIRCLE ( 'NONE', #1903, 0.09999999999999939493 ) ;
#68608=VECTOR ( 'NONE', #149362, 1000.000000000000000 ) ;
#68623=CARTESIAN_POINT ( 'NONE',  ( 21.05000000000000071, -0.09999999999999939493, 6.540656951701244282 ) ) ;
#68627=CARTESIAN_POINT ( 'NONE',  ( -23.25000000000000000, -11.75000000000000000, -30.39999999999999858 ) ) ;
#68629=CARTESIAN_POINT ( 'NONE',  ( -18.40000000000000213, -9.500000000000007105, -6.999362097180126696 ) ) ;
#68637=LINE ( 'NONE', #251096, #56332 ) ;
#68640=DIRECTION ( 'NONE',  ( 6.938893903907224433E-15, -1.000000000000000000, -2.891205793294679805E-16 ) ) ;
#68665=LINE ( 'NONE', #26991, #19935 ) ;
#68698=EDGE_LOOP ( 'NONE', ( #40032, #209497, #208244, #30393 ) ) ;
#68705=CARTESIAN_POINT ( 'NONE',  ( -21.03571358705741190, 11.74999999999999645, -6.825106822058594425 ) ) ;
#68713=DIRECTION ( 'NONE',  ( 0.000000000000000000, 0.000000000000000000, 1.000000000000000000 ) ) ;
#68723=CIRCLE ( 'NONE', #52140, 12.97499999999999609 ) ;
#68767=AXIS2_PLACEMENT_3D ( 'NONE', #45254, #100062, #102628 ) ;
#68791=DIRECTION ( 'NONE',  ( 1.000000000000000000, 0.000000000000000000, -0.000000000000000000 ) ) ;
#68799=DIRECTION ( 'NONE',  ( 0.000000000000000000, 0.000000000000000000, -1.000000000000000000 ) ) ;
#68838=VERTEX_POINT ( 'NONE', #83059 ) ;
#68849=ADVANCED_FACE ( 'NONE', ( #184761 ), #46524, .F. ) ;
#68882=TOROIDAL_SURFACE ( 'NONE', #202142, 1.900000000000002576, 0.1000000000000000056 ) ;
#68908=ORIENTED_EDGE ( 'NONE', *, *, #11219, .F. ) ;
#68911=CARTESIAN_POINT ( 'NONE',  ( 20.95512820512820440, 10.62384868371187707, -12.14999999999999858 ) ) ;
#68931=DIRECTION ( 'NONE',  ( 1.000000000000000000, -0.000000000000000000, -0.000000000000000000 ) ) ;
#68946=AXIS2_PLACEMENT_3D ( 'NONE', #224608, #45977, #206348 ) ;
#69028=CARTESIAN_POINT ( 'NONE',  ( 21.00000000000000000, 9.749999999999998224, -21.15000000000000213 ) ) ;
#69042=AXIS2_PLACEMENT_3D ( 'NONE', #255776, #156752, #98001 ) ;
#69059=CARTESIAN_POINT ( 'NONE',  ( -22.50000000000000000, 11.64987090376337875, 0.08251989087296193737 ) ) ;
#69061=DIRECTION ( 'NONE',  ( 1.000000000000000000, 0.000000000000000000, 0.000000000000000000 ) ) ;
#69083=ORIENTED_EDGE ( 'NONE', *, *, #101500, .F. ) ;
#69087=CARTESIAN_POINT ( 'NONE',  ( -21.12642695952773764, 6.375659922035164406, 0.09890328318936436602 ) ) ;
#69094=ORIENTED_EDGE ( 'NONE', *, *, #127046, .T. ) ;
#69127=ORIENTED_EDGE ( 'NONE', *, *, #232248, .T. ) ;
#69134=CIRCLE ( 'NONE', #160735, 0.1000000000000000056 ) ;
#69161=DIRECTION ( 'NONE',  ( -1.000000000000000000, 0.000000000000000000, 0.000000000000000000 ) ) ;
#69179=ORIENTED_EDGE ( 'NONE', *, *, #40372, .F. ) ;
#69201=CARTESIAN_POINT ( 'NONE',  ( 18.50000000000000000, -9.399999999999998579, -6.999285677838848585 ) ) ;
#69230=VERTEX_POINT ( 'NONE', #141481 ) ;
#69242=DIRECTION ( 'NONE',  ( -0.8660254037843746477, 0.000000000000000000, -0.5000000000001108003 ) ) ;
#69244=ORIENTED_EDGE ( 'NONE', *, *, #138194, .F. ) ;
#69257=DIRECTION ( 'NONE',  ( -0.000000000000000000, -0.000000000000000000, 1.000000000000000000 ) ) ;
#69265=DIRECTION ( 'NONE',  ( -0.000000000000000000, 0.1350103645451904977, 0.9908441862701597991 ) ) ;
#69288=CARTESIAN_POINT ( 'NONE',  ( 21.14999999999999858, 11.65000000000000391, -12.15000000000000036 ) ) ;
#69290=DIRECTION ( 'NONE',  ( 1.000000000000000000, 0.000000000000000000, 0.000000000000000000 ) ) ;
#69303=CARTESIAN_POINT ( 'NONE',  ( 20.94999999999999929, -9.000000000000000000, -23.60603087734755690 ) ) ;
#69326=EDGE_CURVE ( 'NONE', #70529, #44319, #161060, .T. ) ;
#69329=ORIENTED_EDGE ( 'NONE', *, *, #48926, .T. ) ;
#69376=CARTESIAN_POINT ( 'NONE',  ( 21.14999999999999858, 0.000000000000000000, -12.15000000000000036 ) ) ;
#69422=SPHERICAL_SURFACE ( 'NONE', #236575, 0.1000000000000000056 ) ;
#69435=ORIENTED_EDGE ( 'NONE', *, *, #141113, .T. ) ;
#69437=ORIENTED_EDGE ( 'NONE', *, *, #208134, .T. ) ;
#69502=DIRECTION ( 'NONE',  ( 0.000000000000000000, -1.000000000000000000, 0.000000000000000000 ) ) ;
#69532=DIRECTION ( 'NONE',  ( 1.000000000000000000, 0.000000000000000000, 0.000000000000000000 ) ) ;
#69609=LINE ( 'NONE', #126997, #107338 ) ;
#69649=CIRCLE ( 'NONE', #23874, 0.1999999999999987899 ) ;
#69655=DIRECTION ( 'NONE',  ( 0.000000000000000000, 0.000000000000000000, -1.000000000000000000 ) ) ;
#69661=CARTESIAN_POINT ( 'NONE',  ( -23.25000000000000000, 0.000000000000000000, -33.50000000000000000 ) ) ;
#69687=VECTOR ( 'NONE', #256711, 1000.000000000000114 ) ;
#69712=AXIS2_PLACEMENT_3D ( 'NONE', #117216, #118517, #61081 ) ;
#69714=CARTESIAN_POINT ( 'NONE',  ( 23.24999999999999289, 11.75000000000000711, 11.75000000000000000 ) ) ;
#69719=DIRECTION ( 'NONE',  ( 1.000000000000000000, 0.000000000000000000, 0.000000000000000000 ) ) ;
#69731=CIRCLE ( 'NONE', #90369, 11.65000000000000036 ) ;
#69743=FACE_OUTER_BOUND ( 'NONE', #184883, .T. ) ;
#69756=EDGE_CURVE ( 'NONE', #242536, #247150, #89426, .T. ) ;
#69759=DIRECTION ( 'NONE',  ( 1.000000000000000000, 0.000000000000000000, -0.000000000000000000 ) ) ;
#69763=DIRECTION ( 'NONE',  ( -3.265361837132813093E-16, 1.000000000000000000, 0.000000000000000000 ) ) ;
#69766=CARTESIAN_POINT ( 'NONE',  ( -21.05000000000000071, 5.849999999999952571, -10.13249722427796762 ) ) ;
#69862=VECTOR ( 'NONE', #59540, 1000.000000000000000 ) ;
#69864=ORIENTED_EDGE ( 'NONE', *, *, #27578, .F. ) ;
#69871=CIRCLE ( 'NONE', #198839, 0.4000000000000010214 ) ;
#69879=CARTESIAN_POINT ( 'NONE',  ( 20.94788355080264353, 10.30207779524867462, -38.98955207167824000 ) ) ;
#69883=DIRECTION ( 'NONE',  ( 0.000000000000000000, 1.000000000000000000, 0.000000000000000000 ) ) ;
#69893=ORIENTED_EDGE ( 'NONE', *, *, #100861, .F. ) ;
#69900=CIRCLE ( 'NONE', #173978, 0.1000000000000016431 ) ;
#69907=LINE ( 'NONE', #150704, #10088 ) ;
#69913=EDGE_CURVE ( 'NONE', #135260, #7751, #137965, .T. ) ;
#69976=CARTESIAN_POINT ( 'NONE',  ( 18.49999999999998934, 6.550000000000000711, -21.15000000000000213 ) ) ;
#69986=EDGE_CURVE ( 'NONE', #10818, #226600, #2112, .T. ) ;
#70045=CLOSED_SHELL ( 'NONE', ( #31416, #72148, #13180, #182625, #187317, #78204, #229293, #77655, #236123, #171953, #250748, #51690, #254646, #198358, #134691, #155607, #243864, #86274, #117461, #246817, #202243, #174936, #212779, #176402, #160561, #59116, #194141, #113215, #215299, #53261, #225929, #73540, #137377, #81269, #24742, #149155, #135635, #40063, #107032, #235455, #184903, #129351, #90376, #180318, #86144, #116587, #12009, #220399, #124330, #121447, #29144, #238935, #254504, #129716, #249231, #83999, #100747, #13819, #15931, #129930, #256309, #85116, #256475, #34266, #73016, #99823, #255296, #200370, #169811, #99110, #175376, #223605, #179503, #223116, #21125, #97049, #222962, #59546, #7382, #42390, #221832, #107669, #149252, #45544, #85211, #116805, #228710, #225636, #137065, #126759, #242551, #239356, #202473, #74908, #138292, #72039, #175500, #225175, #124343, #212007, #243527, #257793, #129413, #79867, #238948, #20290, #18838, #194282, #86520, #76728, #104564, #53785, #187045, #130018, #144334, #123487, #10446, #776, #22009, #126726, #8380, #54130, #76739, #218398, #93899, #253378, #211631, #57511, #142524, #35398, #37807, #235152, #186251, #88541, #29858, #179763, #142912, #172936, #96423, #245531, #226727, #196246, #212718, #68849, #97544, #245705, #220221, #24202, #9917, #213130, #98446, #249139, #80017, #118821, #7665, #232917, #27360, #67410, #40180, #213940, #246838, #134088, #222757, #8376, #143804, #203893, #139915, #214533, #206926, #76860, #156601, #97924, #1349, #109670, #180587, #249726, #199213, #200376, #221314, #229344, #232234, #236524, #65937, #130072, #100188, #114629, #51069, #147995, #145783, #60373, #79436, #205551, #170705, #14348, #181773, #103581, #187195, #178923, #111457, #243969, #107336, #78648, #196553, #139658, #49039, #27469, #176514, #154927, #137412, #71860, #104151, #107143, #236729, #160466, #249955, #193265, #56107, #94964, #122998, #113457, #57992, #60013, #61094, #138304, #28945, #159171, #94377, #43532, #213238, #182716, #164927, #81860, #74509, #247194, #214915, #243926, #129898, #175139, #152850, #124814, #87532, #27958, #131602, #46296, #146625, #20845, #226555, #77811, #83800, #123432, #220132, #232435, #213920, #41952, #254197, #175972, #48213, #88822, #153325, #90208, #63874, #211100, #100408, #172422, #165143, #203092, #19048, #226061, #193180, #190760, #62880, #55469, #103487, #248264, #59871, #190187, #131772, #90791, #133616, #111097, #117415, #113756, #189610, #50374, #27085, #67036, #37045, #156683, #80070, #132099, #251239, #130101, #7899, #44491, #212483, #239267, #34040, #16292, #56721, #165778, #61921, #176030, #153804, #141291, #197174, #99308, #192423, #115033, #247445, #59594, #21776, #141852, #73751, #251981, #2308, #7411, #43641, #168661, #195973, #5889, #50774, #156060, #977, #77055, #218138, #117276, #205275, #65943, #225122, #229006, #67441, #94529, #2539, #61965, #20460, #188939, #247490, #13580, #243333, #92318, #242171, #55085, #222146, #164216, #51197, #50273, #235937, #227371, #219442, #74794, #27580, #216329, #212194, #66486, #176825, #38122, #246344, #18657, #93612, #115310, #197544, #203570, #41718, #80328, #239792, #48724, #142033, #158250, #22502, #48573, #83363, #168347, #65895, #128270, #173417, #204537, #111995, #5992, #94126, #209422, #47778, #42661, #117260, #132716, #195446, #82996, #203662, #171532, #139601, #179776, #82066, #65548, #19816, #57361, #183096, #14982, #152969, #137394, #199369, #155076, #211366, #35093, #98182, #125876, #13050, #47849, #245857, #176510, #257104, #84118, #207155, #179180, #185686, #35385, #246044, #23263, #149692, #185826, #77736, #160002, #188857, #247512, #78197, #234802, #211044, #103279, #65474, #101616, #96151, #20193, #246057, #175297, #99721, #244855, #131758, #46554, #64071, #17191, #185730, #180052, #158537, #215124, #157137, #151368, #256913, #226043, #76331, #44873, #118441, #18557, #119143, #187781, #33824, #157204, #198730, #154776, #62923, #93178, #254828, #121720, #75617, #164217, #17628, #32596, #171457, #34361, #163161, #17098, #76338, #145409, #41016, #37054, #55880, #107057, #207190, #255523, #28961, #27314 ) ) ;
#70047=DIRECTION ( 'NONE',  ( -1.000000000000000000, -0.000000000000000000, 0.000000000000000000 ) ) ;
#70089=ORIENTED_EDGE ( 'NONE', *, *, #113638, .T. ) ;
#70118=ORIENTED_EDGE ( 'NONE', *, *, #85466, .F. ) ;
#70142=ORIENTED_EDGE ( 'NONE', *, *, #19451, .T. ) ;
#70154=ORIENTED_EDGE ( 'NONE', *, *, #232700, .F. ) ;
#70161=CARTESIAN_POINT ( 'NONE',  ( 21.14999999999999858, 8.786607556600111835, -12.25000000000000000 ) ) ;
#70188=ORIENTED_EDGE ( 'NONE', *, *, #34414, .T. ) ;
#70197=CIRCLE ( 'NONE', #36880, 0.09999999999999939493 ) ;
#70262=CARTESIAN_POINT ( 'NONE',  ( -18.58744394320964233, -9.566385154548546765, -40.32284805387602944 ) ) ;
#70274=DIRECTION ( 'NONE',  ( -0.000000000000000000, -0.000000000000000000, 1.000000000000000000 ) ) ;
#70308=FACE_OUTER_BOUND ( 'NONE', #176237, .T. ) ;
#70325=CARTESIAN_POINT ( 'NONE',  ( 18.33996824403465808, -9.569639859431823936, -40.31906563751653039 ) ) ;
#70339=CARTESIAN_POINT ( 'NONE',  ( 18.50000000000000000, -9.399999999999998579, -7.297259759663296208 ) ) ;
#70359=EDGE_LOOP ( 'NONE', ( #141866, #187877, #33487, #217256 ) ) ;
#70369=AXIS2_PLACEMENT_3D ( 'NONE', #89639, #242300, #63665 ) ;
#70412=DIRECTION ( 'NONE',  ( -0.000000000000000000, 1.000000000000000000, 0.000000000000000000 ) ) ;
#70460=VERTEX_POINT ( 'NONE', #127093 ) ;
#70473=DIRECTION ( 'NONE',  ( 0.000000000000000000, 0.000000000000000000, -1.000000000000000000 ) ) ;
#70476=ORIENTED_EDGE ( 'NONE', *, *, #79494, .F. ) ;
#70511=DIRECTION ( 'NONE',  ( -0.000000000000000000, 0.000000000000000000, 1.000000000000000000 ) ) ;
#70524=ORIENTED_EDGE ( 'NONE', *, *, #191298, .F. ) ;
#70526=CYLINDRICAL_SURFACE ( 'NONE', #230582, 0.09999999999999939493 ) ;
#70527=CARTESIAN_POINT ( 'NONE',  ( -18.50000000000000000, -9.400000000000005684, -40.38204184817266906 ) ) ;
#70529=VERTEX_POINT ( 'NONE', #91822 ) ;
#70593=CARTESIAN_POINT ( 'NONE',  ( 21.05000000000000071, 8.776282895292474961, 0.000000000000000000 ) ) ;
#70635=DIRECTION ( 'NONE',  ( 1.000000000000000000, -0.000000000000000000, -0.000000000000000000 ) ) ;
#70658=ORIENTED_EDGE ( 'NONE', *, *, #82777, .T. ) ;
#70680=CARTESIAN_POINT ( 'NONE',  ( 18.59999999999999076, 10.24999999999999822, -24.75000000000000000 ) ) ;
#70697=ORIENTED_EDGE ( 'NONE', *, *, #25762, .F. ) ;
#70704=AXIS2_PLACEMENT_3D ( 'NONE', #7269, #86796, #63388 ) ;
#70717=DIRECTION ( 'NONE',  ( -1.000000000000000000, 0.000000000000000000, -0.000000000000000000 ) ) ;
#70764=AXIS2_PLACEMENT_3D ( 'NONE', #137563, #38491, #15079 ) ;
#70780=FACE_OUTER_BOUND ( 'NONE', #200322, .T. ) ;
#70784=DIRECTION ( 'NONE',  ( 0.000000000000000000, 0.9875055080513743810, -0.1575844902526802316 ) ) ;
#70792=CARTESIAN_POINT ( 'NONE',  ( 20.85000000000000142, 0.000000000000000000, -33.50000000000000000 ) ) ;
#70805=FACE_OUTER_BOUND ( 'NONE', #175668, .T. ) ;
#70824=CONICAL_SURFACE ( 'NONE', #212457, 7.750000000000026645, 0.7853981633974531640 ) ;
#70831=DIRECTION ( 'NONE',  ( 0.000000000000000000, -0.000000000000000000, 1.000000000000000000 ) ) ;
#70849=DIRECTION ( 'NONE',  ( 1.000000000000000000, 0.000000000000000000, 0.000000000000000000 ) ) ;
#70917=ORIENTED_EDGE ( 'NONE', *, *, #85576, .F. ) ;
#70932=EDGE_CURVE ( 'NONE', #256624, #85343, #77476, .T. ) ;
#70937=FACE_BOUND ( 'NONE', #234940, .T. ) ;
#71010=ORIENTED_EDGE ( 'NONE', *, *, #92792, .T. ) ;
#71013=CARTESIAN_POINT ( 'NONE',  ( 18.39999999999999858, -9.499999999999998224, -7.032069396699667685 ) ) ;
#71036=AXIS2_PLACEMENT_3D ( 'NONE', #79725, #159312, #40672 ) ;
#71041=LINE ( 'NONE', #170167, #230597 ) ;
#71070=CIRCLE ( 'NONE', #195977, 0.1000000000000028644 ) ;
#71076=ORIENTED_EDGE ( 'NONE', *, *, #111677, .F. ) ;
#71153=EDGE_CURVE ( 'NONE', #71514, #196401, #25752, .T. ) ;
#71167=CARTESIAN_POINT ( 'NONE',  ( 21.14999999999999858, 8.786607556600111835, -12.35000000000000320 ) ) ;
#71227=VERTEX_POINT ( 'NONE', #32192 ) ;
#71243=LINE ( 'NONE', #133754, #258084 ) ;
#71298=DIRECTION ( 'NONE',  ( 0.000000000000000000, 0.000000000000000000, 1.000000000000000000 ) ) ;
#71323=CARTESIAN_POINT ( 'NONE',  ( -21.76363531954647357, 0.09900187429944841411, 7.012936547871741588 ) ) ;
#71333=AXIS2_PLACEMENT_3D ( 'NONE', #127432, #105256, #222660 ) ;
#71337=VERTEX_POINT ( 'NONE', #115547 ) ;
#71348=CARTESIAN_POINT ( 'NONE',  ( 23.14999999999999858, 5.499999999999998224, -12.40526601891309788 ) ) ;
#71351=DIRECTION ( 'NONE',  ( 0.000000000000000000, 0.000000000000000000, 1.000000000000000000 ) ) ;
#71370=VERTEX_POINT ( 'NONE', #76415 ) ;
#71396=FACE_OUTER_BOUND ( 'NONE', #40864, .T. ) ;
#71400=CARTESIAN_POINT ( 'NONE',  ( 20.94999999999999929, -9.500000000000001776, -9.893969122652443104 ) ) ;
#71413=CARTESIAN_POINT ( 'NONE',  ( 21.05000000000000071, 8.876614585087102327, -8.385080478844674445 ) ) ;
#71419=CARTESIAN_POINT ( 'NONE',  ( -20.85000000000000142, -1.164121893241208960, -41.41484808557160591 ) ) ;
#71457=EDGE_CURVE ( 'NONE', #163426, #79894, #235905, .T. ) ;
#71460=ORIENTED_EDGE ( 'NONE', *, *, #248130, .F. ) ;
#71476=ORIENTED_EDGE ( 'NONE', *, *, #144500, .T. ) ;
#71514=VERTEX_POINT ( 'NONE', #181954 ) ;
#71518=VERTEX_POINT ( 'NONE', #164951 ) ;
#71519=CARTESIAN_POINT ( 'NONE',  ( 18.59999999999999076, 11.65000000000000391, -24.85000000000000142 ) ) ;
#71520=FACE_BOUND ( 'NONE', #105761, .T. ) ;
#71554=EDGE_CURVE ( 'NONE', #217421, #145230, #101069, .T. ) ;
#71606=DIRECTION ( 'NONE',  ( 0.000000000000000000, -1.000000000000000000, -0.000000000000000000 ) ) ;
#71618=ORIENTED_EDGE ( 'NONE', *, *, #250059, .T. ) ;
#71621=CARTESIAN_POINT ( 'NONE',  ( -21.14999999999999858, -0.09999999999999939493, 11.64957080754479968 ) ) ;
#71650=AXIS2_PLACEMENT_3D ( 'NONE', #208429, #209690, #132735 ) ;
#71661=ORIENTED_EDGE ( 'NONE', *, *, #149373, .T. ) ;
#71677=CARTESIAN_POINT ( 'NONE',  ( -21.05000000000000071, 0.000000000000000000, -7.900000000000000355 ) ) ;
#71739=CARTESIAN_POINT ( 'NONE',  ( 22.49066049874202022, 0.05634325153222827925, 11.65001223751710313 ) ) ;
#71749=ORIENTED_EDGE ( 'NONE', *, *, #179705, .F. ) ;
#71750=CARTESIAN_POINT ( 'NONE',  ( -21.05000000000000071, 0.05132743234157015333, 6.300183336267757284 ) ) ;
#71762=DIRECTION ( 'NONE',  ( -0.000000000000000000, -0.000000000000000000, 1.000000000000000000 ) ) ;
#71783=EDGE_CURVE ( 'NONE', #97122, #233908, #202952, .T. ) ;
#71800=ORIENTED_EDGE ( 'NONE', *, *, #134276, .T. ) ;
#71806=CIRCLE ( 'NONE', #109177, 0.09999999999999939493 ) ;
#71836=FACE_OUTER_BOUND ( 'NONE', #61281, .T. ) ;
#71841=CARTESIAN_POINT ( 'NONE',  ( -21.05000000000000071, 5.265981236333565222E-16, 4.299999999999956302 ) ) ;
#71860=ADVANCED_FACE ( 'NONE', ( #241620 ), #26439, .F. ) ;
#71864=LINE ( 'NONE', #92682, #170327 ) ;
#71883=VERTEX_POINT ( 'NONE', #162106 ) ;
#71901=CARTESIAN_POINT ( 'NONE',  ( 18.49999999999999289, 6.649999999999999467, -21.35000000000000142 ) ) ;
#71925=CARTESIAN_POINT ( 'NONE',  ( -18.59999999999999787, -1.687074390091559906, 12.81457296654165212 ) ) ;
#71940=DIRECTION ( 'NONE',  ( 0.000000000000000000, -1.000000000000000000, -0.000000000000000000 ) ) ;
#72006=AXIS2_PLACEMENT_3D ( 'NONE', #98509, #178120, #257570 ) ;
#72018=DIRECTION ( 'NONE',  ( -1.000000000000000000, -2.952720810173289112E-16, 0.000000000000000000 ) ) ;
#72023=FACE_OUTER_BOUND ( 'NONE', #186409, .T. ) ;
#72039=ADVANCED_FACE ( 'NONE', ( #210213 ), #27747, .F. ) ;
#72046=CYLINDRICAL_SURFACE ( 'NONE', #109824, 0.09999999999999982514 ) ;
#72050=ORIENTED_EDGE ( 'NONE', *, *, #247429, .F. ) ;
#72105=DIRECTION ( 'NONE',  ( 0.000000000000000000, 0.000000000000000000, -1.000000000000000000 ) ) ;
#72117=DIRECTION ( 'NONE',  ( 1.000000000000000000, 2.952720810173289112E-16, -0.000000000000000000 ) ) ;
#72118=CIRCLE ( 'NONE', #76176, 0.09999999999999939493 ) ;
#72126=CIRCLE ( 'NONE', #147122, 0.1000000000000000472 ) ;
#72134=DIRECTION ( 'NONE',  ( 1.000000000000000000, -7.304098846218134667E-16, -4.217023435051626718E-16 ) ) ;
#72148=ADVANCED_FACE ( 'NONE', ( #78375 ), #85841, .T. ) ;
#72182=VERTEX_POINT ( 'NONE', #121407 ) ;
#72228=DIRECTION ( 'NONE',  ( 1.000000000000000000, 0.000000000000000000, 0.000000000000000000 ) ) ;
#72235=DIRECTION ( 'NONE',  ( -0.000000000000000000, 0.000000000000000000, 1.000000000000000000 ) ) ;
#72239=CARTESIAN_POINT ( 'NONE',  ( 23.14999999999999858, 5.499999999999998224, -21.09473398108690390 ) ) ;
#72247=DIRECTION ( 'NONE',  ( -1.000000000000000000, 0.000000000000000000, 0.000000000000000000 ) ) ;
#72252=ORIENTED_EDGE ( 'NONE', *, *, #175685, .T. ) ;
#72259=DIRECTION ( 'NONE',  ( 1.000000000000000000, 0.000000000000000000, -0.000000000000000000 ) ) ;
#72275=ORIENTED_EDGE ( 'NONE', *, *, #98367, .T. ) ;
#72284=CARTESIAN_POINT ( 'NONE',  ( 21.14999999999999858, 6.550000000000000711, -12.15000000000000036 ) ) ;
#72309=VERTEX_POINT ( 'NONE', #227836 ) ;
#72326=CARTESIAN_POINT ( 'NONE',  ( -20.64999999999999858, 0.000000000000000000, -33.50000000000000000 ) ) ;
#72335=CIRCLE ( 'NONE', #176399, 0.09999999999999954758 ) ;
#72420=DIRECTION ( 'NONE',  ( 0.000000000000000000, -1.000000000000000000, 0.000000000000000000 ) ) ;
#72422=ORIENTED_EDGE ( 'NONE', *, *, #134239, .F. ) ;
#72433=CARTESIAN_POINT ( 'NONE',  ( 18.52928932188133970, 10.27928932188134858, -24.65000000000000213 ) ) ;
#72452=CARTESIAN_POINT ( 'NONE',  ( 21.06277459767449756, 8.872862438268244389, -12.20399919235636155 ) ) ;
#72458=CARTESIAN_POINT ( 'NONE',  ( 20.94999999999999929, -12.41227409414968541, -30.50000000000000000 ) ) ;
#72477=CARTESIAN_POINT ( 'NONE',  ( 20.94999999999999929, 10.38178547072394764, -39.00784536388417223 ) ) ;
#72485=CARTESIAN_POINT ( 'NONE',  ( 21.05000000000000071, 10.47338541491290265, -7.578654464248540279 ) ) ;
#72537=VERTEX_POINT ( 'NONE', #80284 ) ;
#72544=ORIENTED_EDGE ( 'NONE', *, *, #32710, .T. ) ;
#72597=EDGE_CURVE ( 'NONE', #41537, #226810, #198475, .T. ) ;
#72636=CARTESIAN_POINT ( 'NONE',  ( 21.30000000000002558, 0.000000000000000000, 0.000000000000000000 ) ) ;
#72647=CARTESIAN_POINT ( 'NONE',  ( -23.25000000000000000, 0.000000000000000000, -4.049999999999998934 ) ) ;
#72682=CARTESIAN_POINT ( 'NONE',  ( -18.50000000000000000, 6.846123162352588665, -37.23772626684986164 ) ) ;
#72726=AXIS2_PLACEMENT_3D ( 'NONE', #20422, #75274, #217298 ) ;
#72736=ORIENTED_EDGE ( 'NONE', *, *, #246037, .F. ) ;
#72737=AXIS2_PLACEMENT_3D ( 'NONE', #224785, #25345, #243076 ) ;
#72741=ORIENTED_EDGE ( 'NONE', *, *, #161868, .F. ) ;
#72742=DIRECTION ( 'NONE',  ( -4.391705002472929091E-16, 1.000000000000000000, 0.000000000000000000 ) ) ;
#72748=CIRCLE ( 'NONE', #89258, 0.1000000000000028644 ) ;
#72766=DIRECTION ( 'NONE',  ( 0.000000000000000000, 1.000000000000000000, -1.224646799147353207E-16 ) ) ;
#72773=VECTOR ( 'NONE', #62851, 1000.000000000000000 ) ;
#72774=CARTESIAN_POINT ( 'NONE',  ( 21.08804281139606118, 10.62183430184116339, -12.34999996737854566 ) ) ;
#72788=CIRCLE ( 'NONE', #256032, 0.09999999999999939493 ) ;
#72815=EDGE_CURVE ( 'NONE', #144794, #136985, #244441, .T. ) ;
#72826=CARTESIAN_POINT ( 'NONE',  ( -18.46154800491006398, -9.480206274242036102, -40.15745083838135798 ) ) ;
#72868=EDGE_LOOP ( 'NONE', ( #74593, #221773, #145715, #95195 ) ) ;
#72877=CARTESIAN_POINT ( 'NONE',  ( 18.39999999999999858, -9.500000000000000000, -7.032069396699673014 ) ) ;
#72878=CARTESIAN_POINT ( 'NONE',  ( 20.94999999999999574, 1.261786168565025568, -8.086498963545480478 ) ) ;
#72902=CYLINDRICAL_SURFACE ( 'NONE', #150558, 0.09999999999999939493 ) ;
#72925=AXIS2_PLACEMENT_3D ( 'NONE', #13362, #113735, #208981 ) ;
#72932=SPHERICAL_SURFACE ( 'NONE', #2143, 0.1000000000000000056 ) ;
#72933=CARTESIAN_POINT ( 'NONE',  ( -18.59999999999999787, 11.64999999999999680, -21.35000000000000142 ) ) ;
#72950=EDGE_LOOP ( 'NONE', ( #160845, #226507, #155347, #36909, #223444 ) ) ;
#72961=CARTESIAN_POINT ( 'NONE',  ( 21.05000000000000071, 6.350000000000004974, -9.843822089683129661 ) ) ;
#72989=ORIENTED_EDGE ( 'NONE', *, *, #66424, .F. ) ;
#72992=VERTEX_POINT ( 'NONE', #66877 ) ;
#73002=DIRECTION ( 'NONE',  ( 0.000000000000000000, 1.776356839400250267E-15, 1.000000000000000000 ) ) ;
#73014=AXIS2_PLACEMENT_3D ( 'NONE', #133652, #228909, #91956 ) ;
#73016=ADVANCED_FACE ( 'NONE', ( #43462 ), #102116, .F. ) ;
#73022=ORIENTED_EDGE ( 'NONE', *, *, #170397, .T. ) ;
#73043=ORIENTED_EDGE ( 'NONE', *, *, #35409, .T. ) ;
#73078=CARTESIAN_POINT ( 'NONE',  ( -22.47120815636973745, 0.02890382190389122891, 11.64993198875349734 ) ) ;
#73179=CIRCLE ( 'NONE', #48192, 11.79999999999999716 ) ;
#73190=EDGE_CURVE ( 'NONE', #203969, #66968, #111362, .T. ) ;
#73238=EDGE_CURVE ( 'NONE', #243786, #239652, #53732, .T. ) ;
#73276=AXIS2_PLACEMENT_3D ( 'NONE', #158892, #100141, #117179 ) ;
#73287=ORIENTED_EDGE ( 'NONE', *, *, #220206, .T. ) ;
#73293=ORIENTED_EDGE ( 'NONE', *, *, #59413, .F. ) ;
#73301=CIRCLE ( 'NONE', #248243, 0.1000000000000002831 ) ;
#73330=CARTESIAN_POINT ( 'NONE',  ( 21.05000000000000071, -9.400000000000000355, -23.60603087734755690 ) ) ;
#73345=LINE ( 'NONE', #51148, #169603 ) ;
#73379=VECTOR ( 'NONE', #186290, 1000.000000000000000 ) ;
#73393=ORIENTED_EDGE ( 'NONE', *, *, #172646, .F. ) ;
#73410=DIRECTION ( 'NONE',  ( -3.265361837132813093E-16, 1.000000000000000000, -0.000000000000000000 ) ) ;
#73425=DIRECTION ( 'NONE',  ( -0.000000000000000000, -0.000000000000000000, 1.000000000000000000 ) ) ;
#73427=LINE ( 'NONE', #151686, #169582 ) ;
#73450=DIRECTION ( 'NONE',  ( 0.000000000000000000, 0.000000000000000000, -1.000000000000000000 ) ) ;
#73461=VERTEX_POINT ( 'NONE', #30046 ) ;
#73465=DIRECTION ( 'NONE',  ( 0.7071067811865474617, 0.7071067811865474617, 0.000000000000000000 ) ) ;
#73479=FACE_OUTER_BOUND ( 'NONE', #257190, .T. ) ;
#73500=AXIS2_PLACEMENT_3D ( 'NONE', #26551, #30402, #188185 ) ;
#73516=ORIENTED_EDGE ( 'NONE', *, *, #124426, .F. ) ;
#73527=CARTESIAN_POINT ( 'NONE',  ( -21.05000000000000071, -11.75000000000000000, -30.59999999999999432 ) ) ;
#73530=EDGE_CURVE ( 'NONE', #20565, #138502, #223775, .T. ) ;
#73534=CYLINDRICAL_SURFACE ( 'NONE', #181795, 0.09999999999999939493 ) ;
#73537=EDGE_CURVE ( 'NONE', #108030, #252270, #177261, .T. ) ;
#73540=ADVANCED_FACE ( 'NONE', ( #212526 ), #18150, .T. ) ;
#73549=CARTESIAN_POINT ( 'NONE',  ( 20.94999999999999929, 4.999999999999997335, -12.40526601891309788 ) ) ;
#73554=AXIS2_PLACEMENT_3D ( 'NONE', #138361, #163105, #256996 ) ;
#73555=AXIS2_PLACEMENT_3D ( 'NONE', #131000, #69763, #187149 ) ;
#73588=DIRECTION ( 'NONE',  ( -0.000000000000000000, 1.000000000000000000, -0.000000000000000000 ) ) ;
#73601=AXIS2_PLACEMENT_3D ( 'NONE', #63156, #222217, #219666 ) ;
#73645=SURFACE_STYLE_USAGE ( .BOTH. , #151895 ) ;
#73658=CARTESIAN_POINT ( 'NONE',  ( -23.25000000000000000, 0.000000000000000000, -33.50000000000000000 ) ) ;
#73663=DIRECTION ( 'NONE',  ( 0.000000000000000000, 0.000000000000000000, -1.000000000000000000 ) ) ;
#73671=EDGE_CURVE ( 'NONE', #201752, #227236, #240725, .T. ) ;
#73705=CARTESIAN_POINT ( 'NONE',  ( 23.14999999999999503, 6.450000000000001066, -21.15000000000000213 ) ) ;
#73707=DIRECTION ( 'NONE',  ( -0.000000000000000000, -0.000000000000000000, 1.000000000000000000 ) ) ;
#73708=VERTEX_POINT ( 'NONE', #79392 ) ;
#73719=FACE_OUTER_BOUND ( 'NONE', #224976, .T. ) ;
#73749=CARTESIAN_POINT ( 'NONE',  ( -18.59999999999999787, 1.835341550224411922, -11.55515129256298046 ) ) ;
#73751=ADVANCED_FACE ( 'NONE', ( #46682 ), #107960, .F. ) ;
#73757=ORIENTED_EDGE ( 'NONE', *, *, #160036, .F. ) ;
#73761=LINE ( 'NONE', #34633, #133149 ) ;
#73831=DIRECTION ( 'NONE',  ( 1.000000000000000000, 0.000000000000000000, 0.000000000000000000 ) ) ;
#73839=ORIENTED_EDGE ( 'NONE', *, *, #221568, .T. ) ;
#73854=ORIENTED_EDGE ( 'NONE', *, *, #229800, .T. ) ;
#73859=AXIS2_PLACEMENT_3D ( 'NONE', #18665, #99459, #193468 ) ;
#73902=ORIENTED_EDGE ( 'NONE', *, *, #210611, .F. ) ;
#73917=DIRECTION ( 'NONE',  ( 1.000000000000000000, 0.000000000000000000, 0.000000000000000000 ) ) ;
#73935=CARTESIAN_POINT ( 'NONE',  ( 21.14999999999999858, 11.75000000000000711, -12.15000000000000036 ) ) ;
#73950=EDGE_LOOP ( 'NONE', ( #29460, #249069, #108520, #76096 ) ) ;
#73974=ORIENTED_EDGE ( 'NONE', *, *, #91523, .T. ) ;
#74004=AXIS2_PLACEMENT_3D ( 'NONE', #114726, #194288, #174745 ) ;
#74011=VECTOR ( 'NONE', #250948, 1000.000000000000000 ) ;
#74027=CARTESIAN_POINT ( 'NONE',  ( 20.85000000000000142, 7.070967871798842452, -37.24656422186831151 ) ) ;
#74138=DIRECTION ( 'NONE',  ( 0.000000000000000000, 0.000000000000000000, -1.000000000000000000 ) ) ;
#74144=DIRECTION ( 'NONE',  ( 0.000000000000000000, -1.000000000000000000, 0.000000000000000000 ) ) ;
#74176=ORIENTED_EDGE ( 'NONE', *, *, #110289, .F. ) ;
#74178=CARTESIAN_POINT ( 'NONE',  ( 18.46932045258647648, -9.670685200265751291, -40.17386037299664991 ) ) ;
#74192=EDGE_CURVE ( 'NONE', #233652, #32887, #145032, .T. ) ;
#74204=AXIS2_PLACEMENT_3D ( 'NONE', #30663, #148021, #47607 ) ;
#74255=AXIS2_PLACEMENT_3D ( 'NONE', #224012, #24566, #244862 ) ;
#74275=CARTESIAN_POINT ( 'NONE',  ( 21.05000000000000071, 8.815452279197549146, -8.420392552614265114 ) ) ;
#74279=DIRECTION ( 'NONE',  ( -1.836970198721029934E-16, 1.000000000000000000, 0.000000000000000000 ) ) ;
#74282=AXIS2_PLACEMENT_3D ( 'NONE', #210374, #252053, #73450 ) ;
#74298=DIRECTION ( 'NONE',  ( 0.000000000000000000, -1.000000000000000000, 0.000000000000000000 ) ) ;
#74319=CARTESIAN_POINT ( 'NONE',  ( 20.94999999999999929, 0.000000000000000000, -33.50000000000000000 ) ) ;
#74329=CARTESIAN_POINT ( 'NONE',  ( 22.49806830649814060, 0.07746431632550720980, 11.64988965483908068 ) ) ;
#74339=VERTEX_POINT ( 'NONE', #149887 ) ;
#74350=DIRECTION ( 'NONE',  ( -3.469446951953635015E-14, -1.000000000000000000, 0.000000000000000000 ) ) ;
#74355=LINE ( 'NONE', #209989, #100113 ) ;
#74358=CARTESIAN_POINT ( 'NONE',  ( -22.49756042579671700, 0.07804633701718154126, 11.64986496110232572 ) ) ;
#74382=AXIS2_PLACEMENT_3D ( 'NONE', #20677, #100159, #81874 ) ;
#74412=DIRECTION ( 'NONE',  ( 0.000000000000000000, -6.308085367188393199E-16, -1.000000000000000000 ) ) ;
#74417=AXIS2_PLACEMENT_3D ( 'NONE', #55758, #91077, #93643 ) ;
#74465=CARTESIAN_POINT ( 'NONE',  ( -23.15000000000000213, 11.65000000000000036, -26.48519422934605672 ) ) ;
#74475=CIRCLE ( 'NONE', #70369, 0.09999999999999939493 ) ;
#74476=CARTESIAN_POINT ( 'NONE',  ( -20.94999999999999929, -11.48912529307605901, -3.100000000000000533 ) ) ;
#74509=ADVANCED_FACE ( 'NONE', ( #239672 ), #121035, .T. ) ;
#74565=LINE ( 'NONE', #75804, #39560 ) ;
#74587=VERTEX_POINT ( 'NONE', #27666 ) ;
#74593=ORIENTED_EDGE ( 'NONE', *, *, #97123, .T. ) ;
#74606=AXIS2_PLACEMENT_3D ( 'NONE', #133349, #79755, #135883 ) ;
#74620=DIRECTION ( 'NONE',  ( 1.000000000000000000, -0.000000000000000000, -0.000000000000000000 ) ) ;
#74624=CARTESIAN_POINT ( 'NONE',  ( -21.07928932188134041, 0.09889514565439468108, 6.328516656393293083 ) ) ;
#74646=EDGE_CURVE ( 'NONE', #191070, #44201, #232270, .T. ) ;
#74655=CARTESIAN_POINT ( 'NONE',  ( 21.00000000000000000, 9.749999999999998224, -12.35000000000000320 ) ) ;
#74688=CIRCLE ( 'NONE', #24799, 11.80000000000000426 ) ;
#74708=DIRECTION ( 'NONE',  ( 0.000000000000000000, 1.000000000000000000, 1.265107689135680095E-16 ) ) ;
#74713=AXIS2_PLACEMENT_3D ( 'NONE', #197079, #181407, #257016 ) ;
#74723=DIRECTION ( 'NONE',  ( 1.000000000000000000, 0.000000000000000000, 0.000000000000000000 ) ) ;
#74780=CARTESIAN_POINT ( 'NONE',  ( 22.59999999999999432, 11.74987124437650721, 0.06542959101367906705 ) ) ;
#74794=ADVANCED_FACE ( 'NONE', ( #139544 ), #176147, .F. ) ;
#74797=AXIS2_PLACEMENT_3D ( 'NONE', #39037, #55986, #135532 ) ;
#74819=CARTESIAN_POINT ( 'NONE',  ( -21.05000000000000071, -1.162701749938009677, -8.099999999999999645 ) ) ;
#74843=FACE_OUTER_BOUND ( 'NONE', #103609, .T. ) ;
#74853=CARTESIAN_POINT ( 'NONE',  ( 21.14999999999999858, 6.649999999999999467, -12.35000000000000142 ) ) ;
#74857=ORIENTED_EDGE ( 'NONE', *, *, #155728, .F. ) ;
#74891=DIRECTION ( 'NONE',  ( 0.000000000000000000, 0.000000000000000000, 1.000000000000000000 ) ) ;
#74895=SURFACE_SIDE_STYLE ('',( #248365 ) ) ;
#74908=ADVANCED_FACE ( 'NONE', ( #24783 ), #83406, .F. ) ;
#74929=PRESENTATION_STYLE_ASSIGNMENT (( #73645 ) ) ;
#74938=EDGE_CURVE ( 'NONE', #138502, #90335, #62211, .T. ) ;
#74954=DIRECTION ( 'NONE',  ( -1.000000000000000000, 0.000000000000000000, 0.000000000000000000 ) ) ;
#74955=AXIS2_PLACEMENT_3D ( 'NONE', #48921, #43803, #84145 ) ;
#75004=ORIENTED_EDGE ( 'NONE', *, *, #123407, .T. ) ;
#75012=CARTESIAN_POINT ( 'NONE',  ( 18.59999999999999076, 6.450000000000001066, -10.01702717044001822 ) ) ;
#75025=CYLINDRICAL_SURFACE ( 'NONE', #155950, 0.09999999999999939493 ) ;
#75030=CARTESIAN_POINT ( 'NONE',  ( -18.59999999999999787, 0.000000000000000000, -41.40000000000000568 ) ) ;
#75055=AXIS2_PLACEMENT_3D ( 'NONE', #3067, #6936, #185576 ) ;
#75094=CIRCLE ( 'NONE', #250037, 4.300000000000032685 ) ;
#75098=ORIENTED_EDGE ( 'NONE', *, *, #104562, .T. ) ;
#75123=EDGE_CURVE ( 'NONE', #97348, #20836, #78919, .T. ) ;
#75131=EDGE_CURVE ( 'NONE', #207350, #245627, #37468, .T. ) ;
#75158=ORIENTED_EDGE ( 'NONE', *, *, #92102, .T. ) ;
#75169=CARTESIAN_POINT ( 'NONE',  ( 20.95512820512820440, 8.876151316288115822, -21.25000000000000000 ) ) ;
#75174=CARTESIAN_POINT ( 'NONE',  ( -23.25000000000000000, 11.75000000000000000, 0.000000000000000000 ) ) ;
#75182=CYLINDRICAL_SURFACE ( 'NONE', #222802, 12.87499999999999822 ) ;
#75198=CARTESIAN_POINT ( 'NONE',  ( -23.25000000000000000, 1.910280373831780176, -12.63136785519894012 ) ) ;
#75239=ORIENTED_EDGE ( 'NONE', *, *, #49334, .F. ) ;
#75241=CARTESIAN_POINT ( 'NONE',  ( -18.54118089899632693, -9.463537631848099707, -7.048577597868117550 ) ) ;
#75264=VECTOR ( 'NONE', #30602, 1000.000000000000114 ) ;
#75274=DIRECTION ( 'NONE',  ( 1.000000000000000000, 0.000000000000000000, 0.000000000000000000 ) ) ;
#75275=ORIENTED_EDGE ( 'NONE', *, *, #131545, .F. ) ;
#75276=FACE_OUTER_BOUND ( 'NONE', #126520, .T. ) ;
#75316=ORIENTED_EDGE ( 'NONE', *, *, #14819, .T. ) ;
#75328=AXIS2_PLACEMENT_3D ( 'NONE', #216384, #37779, #195568 ) ;
#75349=DIRECTION ( 'NONE',  ( 0.000000000000000000, 0.000000000000000000, -1.000000000000000000 ) ) ;
#75360=VECTOR ( 'NONE', #99676, 1000.000000000000000 ) ;
#75383=EDGE_CURVE ( 'NONE', #160000, #241513, #87318, .T. ) ;
#75437=DIRECTION ( 'NONE',  ( -1.000000000000000000, 0.000000000000000000, 0.000000000000000000 ) ) ;
#75452=CARTESIAN_POINT ( 'NONE',  ( 18.36493879433275822, -9.500000806189802915, -40.42214866035106269 ) ) ;
#75465=CARTESIAN_POINT ( 'NONE',  ( -20.94999999999999929, 0.000000000000000000, -29.40000000000000213 ) ) ;
#75469=ORIENTED_EDGE ( 'NONE', *, *, #38397, .F. ) ;
#75474=VERTEX_POINT ( 'NONE', #219422 ) ;
#75484=DIRECTION ( 'NONE',  ( -1.000000000000000000, 0.000000000000000000, -0.000000000000000000 ) ) ;
#75499=CARTESIAN_POINT ( 'NONE',  ( 20.94999999999999929, 2.388061258337340615E-16, -31.59999999999999787 ) ) ;
#75518=EDGE_CURVE ( 'NONE', #54887, #72537, #87494, .T. ) ;
#75521=CARTESIAN_POINT ( 'NONE',  ( -18.50000000000000000, -1.637172712970379918, -11.58215336547201701 ) ) ;
#75563=VERTEX_POINT ( 'NONE', #42113 ) ;
#75575=LINE ( 'NONE', #192935, #250822 ) ;
#75582=CARTESIAN_POINT ( 'NONE',  ( -23.25000000000000000, -1.149570369575693807, -41.31591248450196474 ) ) ;
#75593=CIRCLE ( 'NONE', #204721, 0.1000000000000000472 ) ;
#75600=CARTESIAN_POINT ( 'NONE',  ( 22.43288208788031568, 0.004899854885382672054, 11.64965184371907192 ) ) ;
#75605=DIRECTION ( 'NONE',  ( 0.000000000000000000, 0.000000000000000000, -1.000000000000000000 ) ) ;
#75617=ADVANCED_FACE ( 'NONE', ( #223280 ), #6815, .T. ) ;
#75651=CARTESIAN_POINT ( 'NONE',  ( 18.50000000000046541, 10.44006789214481579, -24.76711774888623196 ) ) ;
#75659=DIRECTION ( 'NONE',  ( -1.000000000000000000, -0.000000000000000000, -0.000000000000000000 ) ) ;
#75706=CARTESIAN_POINT ( 'NONE',  ( 20.85000000000000142, 6.933893972126341509, -37.28564583437357527 ) ) ;
#75718=ORIENTED_EDGE ( 'NONE', *, *, #66151, .F. ) ;
#75722=LINE ( 'NONE', #135663, #123081 ) ;
#75775=CARTESIAN_POINT ( 'NONE',  ( 20.95520789717937404, 10.57693059938495672, -7.580232973874853286 ) ) ;
#75804=CARTESIAN_POINT ( 'NONE',  ( 22.50000000000000000, 7.750000000000007105, 0.09999999999999939493 ) ) ;
#75806=ORIENTED_EDGE ( 'NONE', *, *, #164273, .F. ) ;
#75807=EDGE_CURVE ( 'NONE', #183282, #132561, #62585, .T. ) ;
#75811=AXIS2_PLACEMENT_3D ( 'NONE', #185701, #244370, #124449 ) ;
#75813=ORIENTED_EDGE ( 'NONE', *, *, #27157, .F. ) ;
#75821=EDGE_CURVE ( 'NONE', #37010, #187076, #54915, .T. ) ;
#75829=EDGE_CURVE ( 'NONE', #115218, #243446, #232312, .T. ) ;
#75863=CARTESIAN_POINT ( 'NONE',  ( 21.05000000000000071, 6.450000000000001066, -10.01702717044001822 ) ) ;
#75882=CARTESIAN_POINT ( 'NONE',  ( -23.15000000000000213, 2.571758278209444422E-16, -31.39999999999999858 ) ) ;
#75892=CARTESIAN_POINT ( 'NONE',  ( 20.84999999999998721, -11.75000000000000000, -33.50000000000000000 ) ) ;
#75918=AXIS2_PLACEMENT_3D ( 'NONE', #103788, #256742, #178577 ) ;
#75922=AXIS2_PLACEMENT_3D ( 'NONE', #185964, #166435, #4732 ) ;
#75945=LINE ( 'NONE', #155514, #190231 ) ;
#75964=CARTESIAN_POINT ( 'NONE',  ( -21.55000000000000426, 7.708578643762696636, -21.25000000000000000 ) ) ;
#75978=CARTESIAN_POINT ( 'NONE',  ( 22.49999999999999645, 11.74956712348939014, 0.1008583690987083642 ) ) ;
#76027=ORIENTED_EDGE ( 'NONE', *, *, #82800, .F. ) ;
#76056=CARTESIAN_POINT ( 'NONE',  ( 18.59999999999999076, 10.20857864376269575, -24.65000000000000213 ) ) ;
#76057=DIRECTION ( 'NONE',  ( 1.000000000000000000, -0.000000000000000000, -0.000000000000000000 ) ) ;
#76093=DIRECTION ( 'NONE',  ( 0.000000000000000000, -0.1455152366551522025, -0.9893560106964505163 ) ) ;
#76096=ORIENTED_EDGE ( 'NONE', *, *, #34327, .F. ) ;
#76149=FACE_OUTER_BOUND ( 'NONE', #213550, .T. ) ;
#76153=CARTESIAN_POINT ( 'NONE',  ( 18.59999999999999076, 1.749999999999999778, -11.66951155790164485 ) ) ;
#76172=B_SPLINE_CURVE_WITH_KNOTS ( 'NONE', 3,
 ( #223464, #126950, #104780, #89098, #166115, #248186 ),
 .UNSPECIFIED., .F., .F.,
 ( 4, 2, 4 ),
 ( 0.000000000000000000, 0.0002113392456165982716, 0.0004226784912331965432 ),
 .UNSPECIFIED. ) ;
#76176=AXIS2_PLACEMENT_3D ( 'NONE', #231762, #130067, #150931 ) ;
#76210=AXIS2_PLACEMENT_3D ( 'NONE', #175047, #130723, #254498 ) ;
#76211=ORIENTED_EDGE ( 'NONE', *, *, #54991, .T. ) ;
#76226=ORIENTED_EDGE ( 'NONE', *, *, #29701, .T. ) ;
#76242=DIRECTION ( 'NONE',  ( 1.000000000000000000, -0.000000000000000000, -0.000000000000000000 ) ) ;
#76245=AXIS2_PLACEMENT_3D ( 'NONE', #155962, #95943, #20292 ) ;
#76297=ORIENTED_EDGE ( 'NONE', *, *, #149191, .T. ) ;
#76315=CARTESIAN_POINT ( 'NONE',  ( 21.05000000000000071, -11.48912529307605546, -30.59999999999999432 ) ) ;
#76316=DIRECTION ( 'NONE',  ( 1.000000000000000000, -0.000000000000000000, -0.000000000000000000 ) ) ;
#76327=CIRCLE ( 'NONE', #59754, 0.09999999999999999167 ) ;
#76331=ADVANCED_FACE ( 'NONE', ( #25765 ), #246106, .F. ) ;
#76338=ADVANCED_FACE ( 'NONE', ( #27080 ), #4884, .T. ) ;
#76390=EDGE_LOOP ( 'NONE', ( #79355, #102353, #87680, #249241 ) ) ;
#76415=CARTESIAN_POINT ( 'NONE',  ( 20.94999999999999574, 1.162701749938009677, -8.000000000000000000 ) ) ;
#76442=VECTOR ( 'NONE', #39928, 1000.000000000000000 ) ;
#76454=CARTESIAN_POINT ( 'NONE',  ( 18.50000000000000000, -9.499999999999998224, 11.75000000000000000 ) ) ;
#76482=DIRECTION ( 'NONE',  ( 6.938893903907222067E-15, -1.000000000000000000, -0.000000000000000000 ) ) ;
#76491=CARTESIAN_POINT ( 'NONE',  ( -18.50000000000000000, 11.64999999999999680, -12.15000000000000036 ) ) ;
#76495=ORIENTED_EDGE ( 'NONE', *, *, #64538, .T. ) ;
#76521=ORIENTED_EDGE ( 'NONE', *, *, #178313, .T. ) ;
#76558=ORIENTED_EDGE ( 'NONE', *, *, #66424, .T. ) ;
#76559=ORIENTED_EDGE ( 'NONE', *, *, #231985, .F. ) ;
#76571=CIRCLE ( 'NONE', #80835, 0.09999999999999939493 ) ;
#76579=DIRECTION ( 'NONE',  ( 0.000000000000000000, 0.008583690987128059571, -0.9999631594459056361 ) ) ;
#76609=CARTESIAN_POINT ( 'NONE',  ( 21.05000000000000071, 4.999999999999997335, -21.09473398108690390 ) ) ;
#76658=DIRECTION ( 'NONE',  ( 1.441126678808781001E-14, 0.9876197685951252359, 0.1568667991644863424 ) ) ;
#76679=LINE ( 'NONE', #96240, #27621 ) ;
#76698=DIRECTION ( 'NONE',  ( 1.000000000000000000, 0.000000000000000000, 3.523657060577910710E-15 ) ) ;
#76728=ADVANCED_FACE ( 'NONE', ( #62028 ), #221075, .F. ) ;
#76739=ADVANCED_FACE ( 'NONE', ( #3301 ), #142806, .T. ) ;
#76771=CARTESIAN_POINT ( 'NONE',  ( -21.05000000000000071, 6.257814610476114758, 0.09779029130879343668 ) ) ;
#76784=ORIENTED_EDGE ( 'NONE', *, *, #163953, .F. ) ;
#76796=ORIENTED_EDGE ( 'NONE', *, *, #168829, .F. ) ;
#76803=CARTESIAN_POINT ( 'NONE',  ( -20.94999999999999929, -11.65000000000000036, -2.900000000000003464 ) ) ;
#76849=CARTESIAN_POINT ( 'NONE',  ( 20.22894356738451194, 9.278498222838468479, -8.268522906243765291 ) ) ;
#76852=EDGE_LOOP ( 'NONE', ( #208307, #140348, #168278, #130345, #75275 ) ) ;
#76860=ADVANCED_FACE ( 'NONE', ( #172725 ), #9738, .F. ) ;
#76874=CARTESIAN_POINT ( 'NONE',  ( -22.47886152344871036, 0.03750093886169331148, 11.64998864304793003 ) ) ;
#76884=AXIS2_PLACEMENT_3D ( 'NONE', #242354, #79413, #256736 ) ;
#76911=DIRECTION ( 'NONE',  ( 0.000000000000000000, 0.000000000000000000, -1.000000000000000000 ) ) ;
#76939=CARTESIAN_POINT ( 'NONE',  ( -23.15000000000000213, -4.831324760622930370, -16.96969694219874825 ) ) ;
#76983=CARTESIAN_POINT ( 'NONE',  ( 20.94999999999999929, 0.000000000000000000, -41.30000000000000426 ) ) ;
#76989=DIRECTION ( 'NONE',  ( 1.000000000000000000, 0.000000000000000000, 0.000000000000000000 ) ) ;
#77003=ORIENTED_EDGE ( 'NONE', *, *, #124441, .F. ) ;
#77009=ORIENTED_EDGE ( 'NONE', *, *, #256879, .T. ) ;
#77025=ORIENTED_EDGE ( 'NONE', *, *, #146427, .T. ) ;
#77038=CARTESIAN_POINT ( 'NONE',  ( 20.95132126680579887, 10.48994987014678770, -7.570324538434519468 ) ) ;
#77042=EDGE_LOOP ( 'NONE', ( #120295, #137001, #145023, #206947 ) ) ;
#77055=ADVANCED_FACE ( 'NONE', ( #236490 ), #233459, .T. ) ;
#77082=CARTESIAN_POINT ( 'NONE',  ( 21.05000000000000071, -9.400000000000000355, -23.60603087734755690 ) ) ;
#77132=VERTEX_POINT ( 'NONE', #199957 ) ;
#77138=DIRECTION ( 'NONE',  ( 0.000000000000000000, 0.000000000000000000, -1.000000000000000000 ) ) ;
#77170=DIRECTION ( 'NONE',  ( 0.000000000000000000, 0.4999999999999994449, 0.8660254037844390407 ) ) ;
#77171=CIRCLE ( 'NONE', #222918, 0.2000000000000005107 ) ;
#77184=EDGE_CURVE ( 'NONE', #169096, #113211, #254257, .T. ) ;
#77190=AXIS2_PLACEMENT_3D ( 'NONE', #59292, #116740, #176737 ) ;
#77192=EDGE_CURVE ( 'NONE', #113369, #79663, #208507, .T. ) ;
#77208=FACE_OUTER_BOUND ( 'NONE', #42250, .T. ) ;
#77218=ORIENTED_EDGE ( 'NONE', *, *, #210132, .F. ) ;
#77225=FACE_OUTER_BOUND ( 'NONE', #181591, .T. ) ;
#77228=CARTESIAN_POINT ( 'NONE',  ( -20.64999999999999858, 4.349999999999999645, -12.25000000000000000 ) ) ;
#77235=CARTESIAN_POINT ( 'NONE',  ( -18.58735405345342784, -9.566478620336599903, -40.32271464626595758 ) ) ;
#77246=FACE_OUTER_BOUND ( 'NONE', #199573, .T. ) ;
#77352=AXIS2_PLACEMENT_3D ( 'NONE', #36140, #116942, #238156 ) ;
#77363=CARTESIAN_POINT ( 'NONE',  ( -18.59999999999999787, -1.835341550224411922, -11.55515129256297868 ) ) ;
#77368=EDGE_CURVE ( 'NONE', #106325, #59419, #104408, .T. ) ;
#77399=VERTEX_POINT ( 'NONE', #58491 ) ;
#77408=VERTEX_POINT ( 'NONE', #157662 ) ;
#77413=TOROIDAL_SURFACE ( 'NONE', #110749, 6.258578643762712446, 0.1000000000000000056 ) ;
#77439=ORIENTED_EDGE ( 'NONE', *, *, #50517, .T. ) ;
#77476=CIRCLE ( 'NONE', #48465, 11.80000000000000249 ) ;
#77485=CARTESIAN_POINT ( 'NONE',  ( -21.46681500597532022, -5.827586677109586333E-16, 6.857511159431289194 ) ) ;
#77516=EDGE_CURVE ( 'NONE', #205304, #11636, #112815, .T. ) ;
#77517=DIRECTION ( 'NONE',  ( -2.840903330521631775E-16, 0.8700118002898321601, -0.4930308989875230030 ) ) ;
#77538=CARTESIAN_POINT ( 'NONE',  ( -20.64999999999999858, 1.999999999999998224, -20.27537807723789953 ) ) ;
#77540=EDGE_CURVE ( 'NONE', #150108, #239317, #96225, .T. ) ;
#77551=ORIENTED_EDGE ( 'NONE', *, *, #25433, .T. ) ;
#77596=DIRECTION ( 'NONE',  ( 1.000000000000000000, 0.000000000000000000, 0.000000000000000000 ) ) ;
#77649=EDGE_LOOP ( 'NONE', ( #162799, #243729, #70476, #123716, #166917 ) ) ;
#77655=ADVANCED_FACE ( 'NONE', ( #113048 ), #117739, .F. ) ;
#77680=CARTESIAN_POINT ( 'NONE',  ( -18.50000000000000000, 7.120270961697591439, -37.15956304183932701 ) ) ;
#77684=EDGE_CURVE ( 'NONE', #166580, #177411, #206208, .T. ) ;
#77688=EDGE_CURVE ( 'NONE', #143019, #63983, #46807, .T. ) ;
#77694=ORIENTED_EDGE ( 'NONE', *, *, #20771, .T. ) ;
#77698=ORIENTED_EDGE ( 'NONE', *, *, #189081, .T. ) ;
#77709=ORIENTED_EDGE ( 'NONE', *, *, #229436, .T. ) ;
#77736=ADVANCED_FACE ( 'NONE', ( #77747 ), #200950, .T. ) ;
#77747=FACE_OUTER_BOUND ( 'NONE', #240138, .T. ) ;
#77758=CARTESIAN_POINT ( 'NONE',  ( -18.59999999999999787, -9.321008403361290107, -7.235938249077882745 ) ) ;
#77765=DIRECTION ( 'NONE',  ( 1.000000000000000000, -7.304098846218133681E-16, -2.111765289898285610E-31 ) ) ;
#77811=ADVANCED_FACE ( 'NONE', ( #154352 ), #175198, .T. ) ;
#77846=ORIENTED_EDGE ( 'NONE', *, *, #58529, .T. ) ;
#77859=CIRCLE ( 'NONE', #119590, 0.1000000000000028644 ) ;
#77866=AXIS2_PLACEMENT_3D ( 'NONE', #183984, #202270, #160603 ) ;
#77868=CARTESIAN_POINT ( 'NONE',  ( -22.59999970745345976, -0.009356377326984025716, 11.75051320766921314 ) ) ;
#77873=ORIENTED_EDGE ( 'NONE', *, *, #19103, .T. ) ;
#77937=CARTESIAN_POINT ( 'NONE',  ( 21.05000000000000071, -0.1000000000000011297, 6.540656951701244282 ) ) ;
#77955=DIRECTION ( 'NONE',  ( -1.000000000000000000, 0.000000000000000000, 0.000000000000000000 ) ) ;
#77956=CARTESIAN_POINT ( 'NONE',  ( 18.49999999999998579, -9.321008403361311423, -7.235938249077851658 ) ) ;
#77997=CARTESIAN_POINT ( 'NONE',  ( 18.59999999999999076, 14.05000000000000959, -5.513695070760984862 ) ) ;
#78018=ORIENTED_EDGE ( 'NONE', *, *, #188128, .T. ) ;
#78021=ORIENTED_EDGE ( 'NONE', *, *, #18501, .T. ) ;
#78027=FACE_OUTER_BOUND ( 'NONE', #213251, .T. ) ;
#78043=CARTESIAN_POINT ( 'NONE',  ( -21.07933241753356413, 0.09337959041926464920, 6.328645948379739039 ) ) ;
#78084=LINE ( 'NONE', #158948, #224046 ) ;
#78106=DIRECTION ( 'NONE',  ( -0.000000000000000000, -0.000000000000000000, 1.000000000000000000 ) ) ;
#78114=CARTESIAN_POINT ( 'NONE',  ( -18.59999999999999787, 9.250000000000001776, -12.25000000000000000 ) ) ;
#78126=CARTESIAN_POINT ( 'NONE',  ( 20.21567752745019320, 10.19811410123150353, -7.882620347651839943 ) ) ;
#78128=FACE_OUTER_BOUND ( 'NONE', #117791, .T. ) ;
#78132=EDGE_LOOP ( 'NONE', ( #171382, #173697, #193887, #181007 ) ) ;
#78151=CARTESIAN_POINT ( 'NONE',  ( -21.05000000000000426, -0.09999999999999968636, 6.477067021124752522 ) ) ;
#78158=DIRECTION ( 'NONE',  ( 1.000000000000000000, 0.000000000000000000, -0.000000000000000000 ) ) ;
#78160=CARTESIAN_POINT ( 'NONE',  ( 23.14999999999999858, 0.000000000000000000, -33.50000000000000000 ) ) ;
#78182=EDGE_CURVE ( 'NONE', #23701, #183417, #67856, .T. ) ;
#78197=ADVANCED_FACE ( 'NONE', ( #78738 ), #117875, .T. ) ;
#78199=CYLINDRICAL_SURFACE ( 'NONE', #208602, 0.1000000000000028644 ) ;
#78204=ADVANCED_FACE ( 'NONE', ( #222087 ), #17957, .T. ) ;
#78247=ORIENTED_EDGE ( 'NONE', *, *, #169395, .F. ) ;
#78255=DIRECTION ( 'NONE',  ( 0.000000000000000000, -0.000000000000000000, 1.000000000000000000 ) ) ;
#78268=ORIENTED_EDGE ( 'NONE', *, *, #150711, .T. ) ;
#78331=CARTESIAN_POINT ( 'NONE',  ( -18.50000000000000000, 11.64999999999999680, -12.25000000000000000 ) ) ;
#78348=ORIENTED_EDGE ( 'NONE', *, *, #52722, .F. ) ;
#78356=EDGE_CURVE ( 'NONE', #31598, #126171, #176208, .T. ) ;
#78361=CARTESIAN_POINT ( 'NONE',  ( -20.54999999999999716, 7.150000000000000355, -16.75000000000000000 ) ) ;
#78370=CARTESIAN_POINT ( 'NONE',  ( 21.14999999999999503, -0.09999999999999939493, 11.64957080754479968 ) ) ;
#78375=FACE_OUTER_BOUND ( 'NONE', #77649, .T. ) ;
#78389=CARTESIAN_POINT ( 'NONE',  ( -21.55000000000000426, 7.750000000000003553, -21.25000000000000000 ) ) ;
#78416=DIRECTION ( 'NONE',  ( -1.000000000000000000, 0.000000000000000000, 0.000000000000000000 ) ) ;
#78463=CARTESIAN_POINT ( 'NONE',  ( -20.00857864376270001, 9.250000000000001776, -12.34999999999999964 ) ) ;
#78499=VECTOR ( 'NONE', #171522, 1000.000000000000000 ) ;
#78502=AXIS2_PLACEMENT_3D ( 'NONE', #61383, #183901, #5230 ) ;
#78508=ORIENTED_EDGE ( 'NONE', *, *, #114447, .T. ) ;
#78530=CARTESIAN_POINT ( 'NONE',  ( 22.49544290803761015, 11.74987023785715756, 0.06531195925763526311 ) ) ;
#78587=VERTEX_POINT ( 'NONE', #82279 ) ;
#78604=AXIS2_PLACEMENT_3D ( 'NONE', #133049, #215139, #177333 ) ;
#78623=EDGE_CURVE ( 'NONE', #172615, #170111, #72335, .T. ) ;
#78648=ADVANCED_FACE ( 'NONE', ( #167023 ), #242994, .T. ) ;
#78692=ORIENTED_EDGE ( 'NONE', *, *, #57577, .F. ) ;
#78697=EDGE_CURVE ( 'NONE', #128006, #56398, #217700, .T. ) ;
#78700=EDGE_CURVE ( 'NONE', #20887, #109, #105603, .T. ) ;
#78733=FACE_OUTER_BOUND ( 'NONE', #213536, .T. ) ;
#78738=FACE_OUTER_BOUND ( 'NONE', #53350, .T. ) ;
#78745=CARTESIAN_POINT ( 'NONE',  ( -18.50000000000000000, 9.350000000000001421, -12.34999999999999964 ) ) ;
#78749=CARTESIAN_POINT ( 'NONE',  ( 21.07888907270776002, 10.72506921351522102, -12.22119358683319135 ) ) ;
#78808=CARTESIAN_POINT ( 'NONE',  ( -20.94999999999999929, 11.64999999999999680, -33.50000000000000000 ) ) ;
#78828=DIRECTION ( 'NONE',  ( 0.000000000000000000, 0.000000000000000000, -1.000000000000000000 ) ) ;
#78831=CARTESIAN_POINT ( 'NONE',  ( 23.14999999999999858, -3.899999999999999467, -33.50000000000000000 ) ) ;
#78871=DIRECTION ( 'NONE',  ( 0.000000000000000000, 1.224646799147353207E-16, 1.000000000000000000 ) ) ;
#78886=CIRCLE ( 'NONE', #124713, 0.1000000000000008799 ) ;
#78887=ORIENTED_EDGE ( 'NONE', *, *, #239545, .F. ) ;
#78897=CARTESIAN_POINT ( 'NONE',  ( 18.49999999999999289, 6.846123162352588665, -37.23772626684986164 ) ) ;
#78919=CIRCLE ( 'NONE', #233113, 0.4000000000000010214 ) ;
#78923=VECTOR ( 'NONE', #68640, 1000.000000000000000 ) ;
#78953=ORIENTED_EDGE ( 'NONE', *, *, #1009, .T. ) ;
#78990=ORIENTED_EDGE ( 'NONE', *, *, #27637, .T. ) ;
#79071=AXIS2_PLACEMENT_3D ( 'NONE', #13168, #112277, #176109 ) ;
#79078=VERTEX_POINT ( 'NONE', #191075 ) ;
#79159=DIRECTION ( 'NONE',  ( 0.000000000000000000, 0.000000000000000000, 1.000000000000000000 ) ) ;
#79187=CIRCLE ( 'NONE', #66748, 0.09999999999999939493 ) ;
#79194=CARTESIAN_POINT ( 'NONE',  ( 21.05000000000000071, 6.413978881488429984, -0.08579911627414654740 ) ) ;
#79202=CIRCLE ( 'NONE', #224945, 0.1999999999999987899 ) ;
#79211=CARTESIAN_POINT ( 'NONE',  ( 21.05000000000000071, -0.01454569056957751363, 6.497017786431992015 ) ) ;
#79250=DIRECTION ( 'NONE',  ( 0.000000000000000000, -1.000000000000000000, 0.000000000000000000 ) ) ;
#79304=CARTESIAN_POINT ( 'NONE',  ( 21.08489247129321242, 8.877675190870073507, -12.35000000000000142 ) ) ;
#79315=CARTESIAN_POINT ( 'NONE',  ( -21.08376601933334271, 0.06377601092987864040, 6.341947271275729214 ) ) ;
#79324=EDGE_CURVE ( 'NONE', #82580, #161077, #102180, .T. ) ;
#79347=TOROIDAL_SURFACE ( 'NONE', #141898, 12.97499999999999787, 0.1000000000000000056 ) ;
#79351=EDGE_LOOP ( 'NONE', ( #191932, #65993, #55079, #33986 ) ) ;
#79355=ORIENTED_EDGE ( 'NONE', *, *, #63368, .F. ) ;
#79365=EDGE_LOOP ( 'NONE', ( #220676, #14154, #104325, #220547 ) ) ;
#79391=AXIS2_PLACEMENT_3D ( 'NONE', #159356, #62806, #121525 ) ;
#79392=CARTESIAN_POINT ( 'NONE',  ( -20.54999999999999716, 4.349999999999999645, -21.15000000000000213 ) ) ;
#79394=ORIENTED_EDGE ( 'NONE', *, *, #237579, .T. ) ;
#79413=DIRECTION ( 'NONE',  ( 1.000000000000000000, 3.469446951953704435E-14, -2.003086131649669752E-14 ) ) ;
#79430=LINE ( 'NONE', #1175, #230001 ) ;
#79436=ADVANCED_FACE ( 'NONE', ( #225979 ), #126923, .T. ) ;
#79440=TOROIDAL_SURFACE ( 'NONE', #204338, 11.70000000000000107, 0.1000000000000000056 ) ;
#79465=ORIENTED_EDGE ( 'NONE', *, *, #41835, .T. ) ;
#79471=CYLINDRICAL_SURFACE ( 'NONE', #46302, 0.1000000000000028644 ) ;
#79494=EDGE_CURVE ( 'NONE', #18766, #180038, #23617, .T. ) ;
#79504=CARTESIAN_POINT ( 'NONE',  ( -22.39999999999999858, 7.790779598373403836, 0.000000000000000000 ) ) ;
#79515=CIRCLE ( 'NONE', #33789, 7.900000000000000355 ) ;
#79531=DIRECTION ( 'NONE',  ( 0.000000000000000000, 1.000000000000000000, -1.224646799147353207E-16 ) ) ;
#79535=CYLINDRICAL_SURFACE ( 'NONE', #197383, 7.900000000000003908 ) ;
#79554=CARTESIAN_POINT ( 'NONE',  ( 21.10320863425824811, 6.400277386459165996, 0.02502225122713586103 ) ) ;
#79598=CIRCLE ( 'NONE', #229646, 0.1000000000000017958 ) ;
#79606=CARTESIAN_POINT ( 'NONE',  ( -21.05000000000000071, 1.162701749938009677, -8.099999999999999645 ) ) ;
#79651=EDGE_CURVE ( 'NONE', #182491, #94835, #206916, .T. ) ;
#79663=VERTEX_POINT ( 'NONE', #52498 ) ;
#79666=ORIENTED_EDGE ( 'NONE', *, *, #194064, .T. ) ;
#79673=ORIENTED_EDGE ( 'NONE', *, *, #250234, .F. ) ;
#79725=CARTESIAN_POINT ( 'NONE',  ( 20.85000000000000142, 0.000000000000000000, -33.50000000000000000 ) ) ;
#79730=EDGE_CURVE ( 'NONE', #41537, #28425, #216198, .T. ) ;
#79745=CARTESIAN_POINT ( 'NONE',  ( 21.05000000000000071, -9.000000000000000000, -23.60603087734755690 ) ) ;
#79755=DIRECTION ( 'NONE',  ( 1.000000000000000000, 0.000000000000000000, 0.000000000000000000 ) ) ;
#79771=CYLINDRICAL_SURFACE ( 'NONE', #79391, 0.09999999999999939493 ) ;
#79799=CARTESIAN_POINT ( 'NONE',  ( 22.49999999999999645, 11.64957080754479968, 0.09999999999999595324 ) ) ;
#79815=ORIENTED_EDGE ( 'NONE', *, *, #161247, .T. ) ;
#79853=CARTESIAN_POINT ( 'NONE',  ( -20.94999999999999929, 10.29270135740183179, -38.95736188715193293 ) ) ;
#79867=ADVANCED_FACE ( 'NONE', ( #225677 ), #7965, .F. ) ;
#79872=ORIENTED_EDGE ( 'NONE', *, *, #160593, .T. ) ;
#79894=VERTEX_POINT ( 'NONE', #165765 ) ;
#79898=CARTESIAN_POINT ( 'NONE',  ( 23.14999999999999858, 5.599999999999996980, -12.40526601891309788 ) ) ;
#79928=ORIENTED_EDGE ( 'NONE', *, *, #169215, .T. ) ;
#79929=CARTESIAN_POINT ( 'NONE',  ( 20.94999999999999929, 5.499999999999998224, -12.40526601891309788 ) ) ;
#79936=AXIS2_PLACEMENT_3D ( 'NONE', #46729, #126268, #243657 ) ;
#79953=VERTEX_POINT ( 'NONE', #113465 ) ;
#79954=ORIENTED_EDGE ( 'NONE', *, *, #231477, .T. ) ;
#79979=EDGE_CURVE ( 'NONE', #156671, #180654, #229578, .T. ) ;
#79991=AXIS2_PLACEMENT_3D ( 'NONE', #76609, #253952, #117029 ) ;
#79994=CARTESIAN_POINT ( 'NONE',  ( -23.15000000000000213, 11.65000000000000036, -12.15000000000000036 ) ) ;
#80014=CARTESIAN_POINT ( 'NONE',  ( 21.14999999999999858, -11.75000000000000000, -12.25000000000000000 ) ) ;
#80017=ADVANCED_FACE ( 'NONE', ( #178610 ), #157240, .T. ) ;
#80020=FACE_OUTER_BOUND ( 'NONE', #80915, .T. ) ;
#80049=DIRECTION ( 'NONE',  ( 0.000000000000000000, -1.000000000000000000, 0.000000000000000000 ) ) ;
#80068=DIRECTION ( 'NONE',  ( 0.000000000000000000, 0.000000000000000000, -1.000000000000000000 ) ) ;
#80070=ADVANCED_FACE ( 'NONE', ( #119925 ), #7168, .T. ) ;
#80082=CARTESIAN_POINT ( 'NONE',  ( -21.07928932188134041, 6.328516656393293083, 0.09889514565439641580 ) ) ;
#80105=VERTEX_POINT ( 'NONE', #138147 ) ;
#80128=ORIENTED_EDGE ( 'NONE', *, *, #184766, .F. ) ;
#80131=CARTESIAN_POINT ( 'NONE',  ( 18.49999999999999645, -1.637172712970381694, -11.58215336547201701 ) ) ;
#80173=CARTESIAN_POINT ( 'NONE',  ( 20.04142135623730070, 11.75000000000000355, -24.65000000000000213 ) ) ;
#80178=FACE_OUTER_BOUND ( 'NONE', #13074, .T. ) ;
#80195=EDGE_CURVE ( 'NONE', #197965, #44715, #173837, .T. ) ;
#80205=DIRECTION ( 'NONE',  ( 0.000000000000000000, 0.000000000000000000, -1.000000000000000000 ) ) ;
#80224=CIRCLE ( 'NONE', #80415, 0.5000000000000004441 ) ;
#80236=EDGE_LOOP ( 'NONE', ( #14, #16423, #212161, #175309 ) ) ;
#80279=EDGE_CURVE ( 'NONE', #222808, #255460, #153163, .T. ) ;
#80284=CARTESIAN_POINT ( 'NONE',  ( -23.25000000000000000, 4.150000000000001243, -21.14999999999999858 ) ) ;
#80286=CARTESIAN_POINT ( 'NONE',  ( -22.59999999999999787, 11.74956712348939192, 0.1008583690987087389 ) ) ;
#80292=DIRECTION ( 'NONE',  ( 0.000000000000000000, 0.000000000000000000, -1.000000000000000000 ) ) ;
#80302=CARTESIAN_POINT ( 'NONE',  ( -23.15000000000000213, 0.000000000000000000, -12.87499999999999822 ) ) ;
#80328=ADVANCED_FACE ( 'NONE', ( #53187 ), #135273, .F. ) ;
#80337=ORIENTED_EDGE ( 'NONE', *, *, #204325, .T. ) ;
#80344=CARTESIAN_POINT ( 'NONE',  ( -20.54999999999999716, 0.000000000000000000, -12.97499999999999609 ) ) ;
#80406=CARTESIAN_POINT ( 'NONE',  ( -21.05000000000000071, 0.000000000000000000, -33.50000000000000000 ) ) ;
#80415=AXIS2_PLACEMENT_3D ( 'NONE', #79745, #120224, #180176 ) ;
#80436=CARTESIAN_POINT ( 'NONE',  ( -18.50000000000000000, 11.74999999999999645, -21.35000000000000142 ) ) ;
#80452=CARTESIAN_POINT ( 'NONE',  ( 21.09096482362060243, 6.363544365404417036, 0.03944827877412642597 ) ) ;
#80453=CARTESIAN_POINT ( 'NONE',  ( 20.85000000000000142, 11.75000000000000355, -26.71613433702190932 ) ) ;
#80463=CARTESIAN_POINT ( 'NONE',  ( 22.50000000000000000, 11.64957080754479968, 0.09999999999999592548 ) ) ;
#80474=CARTESIAN_POINT ( 'NONE',  ( 21.09107601085572981, 0.03930716471739142265, 6.363877975359904404 ) ) ;
#80491=CARTESIAN_POINT ( 'NONE',  ( -23.15000000000000213, 11.65000000000000036, -21.35000000000000142 ) ) ;
#80510=EDGE_LOOP ( 'NONE', ( #257681, #204566, #65053, #156321 ) ) ;
#80580=CARTESIAN_POINT ( 'NONE',  ( 18.59999999999999076, 10.20857864376269575, -21.35000000000000142 ) ) ;
#80587=DIRECTION ( 'NONE',  ( 1.000000000000000000, -0.000000000000000000, -0.000000000000000000 ) ) ;
#80640=DIRECTION ( 'NONE',  ( 1.000000000000000000, -0.000000000000000000, -0.000000000000000000 ) ) ;
#80655=ORIENTED_EDGE ( 'NONE', *, *, #124593, .T. ) ;
#80673=CARTESIAN_POINT ( 'NONE',  ( -20.54999999999999716, -9.500000000000003553, -9.893969122652444881 ) ) ;
#80675=AXIS2_PLACEMENT_3D ( 'NONE', #110666, #229343, #230626 ) ;
#80739=AXIS2_PLACEMENT_3D ( 'NONE', #125844, #25489, #183269 ) ;
#80742=DIRECTION ( 'NONE',  ( 0.000000000000000000, 0.000000000000000000, -1.000000000000000000 ) ) ;
#80750=DIRECTION ( 'NONE',  ( 0.000000000000000000, 0.000000000000000000, -1.000000000000000000 ) ) ;
#80778=ORIENTED_EDGE ( 'NONE', *, *, #55379, .F. ) ;
#80803=EDGE_LOOP ( 'NONE', ( #188115, #52673, #112458, #206472 ) ) ;
#80816=EDGE_LOOP ( 'NONE', ( #177778, #94865, #178710, #199031, #126055, #52480, #31051, #137957, #139862, #33453 ) ) ;
#80822=ORIENTED_EDGE ( 'NONE', *, *, #5826, .T. ) ;
#80835=AXIS2_PLACEMENT_3D ( 'NONE', #4187, #163286, #125440 ) ;
#80862=ORIENTED_EDGE ( 'NONE', *, *, #19103, .F. ) ;
#80888=ORIENTED_EDGE ( 'NONE', *, *, #11560, .F. ) ;
#80889=FACE_OUTER_BOUND ( 'NONE', #107759, .T. ) ;
#80915=EDGE_LOOP ( 'NONE', ( #133791, #114217, #38195, #152314 ) ) ;
#80933=ORIENTED_EDGE ( 'NONE', *, *, #174256, .T. ) ;
#80972=DIRECTION ( 'NONE',  ( 0.000000000000000000, 0.000000000000000000, -1.000000000000000000 ) ) ;
#80983=DIRECTION ( 'NONE',  ( -1.000000000000000000, 0.000000000000000000, 0.000000000000000000 ) ) ;
#81017=CARTESIAN_POINT ( 'NONE',  ( -20.64999999999999858, -8.730841121495325652, -23.90192528101566793 ) ) ;
#81029=ORIENTED_EDGE ( 'NONE', *, *, #134385, .T. ) ;
#81072=AXIS2_PLACEMENT_3D ( 'NONE', #16031, #56393, #159380 ) ;
#81085=TOROIDAL_SURFACE ( 'NONE', #106021, 0.9750000000000019762, 0.1000000000000000056 ) ;
#81167=AXIS2_PLACEMENT_3D ( 'NONE', #201527, #98529, #178142 ) ;
#81178=CIRCLE ( 'NONE', #10299, 0.09999999999999939493 ) ;
#81188=ORIENTED_EDGE ( 'NONE', *, *, #245725, .T. ) ;
#81190=DIRECTION ( 'NONE',  ( 0.000000000000000000, -0.3738317757009658182, 0.9274965247785366129 ) ) ;
#81194=EDGE_LOOP ( 'NONE', ( #195234, #113934, #50712, #254624 ) ) ;
#81221=EDGE_CURVE ( 'NONE', #138366, #62457, #191836, .T. ) ;
#81257=EDGE_LOOP ( 'NONE', ( #217785, #234641, #118639, #27196 ) ) ;
#81269=ADVANCED_FACE ( 'NONE', ( #25980 ), #66178, .T. ) ;
#81348=DIRECTION ( 'NONE',  ( 0.000000000000000000, 0.000000000000000000, 1.000000000000000000 ) ) ;
#81366=LINE ( 'NONE', #78808, #165989 ) ;
#81376=CARTESIAN_POINT ( 'NONE',  ( -20.64999999999999858, 0.000000000000000000, -12.97499999999999609 ) ) ;
#81398=DIRECTION ( 'NONE',  ( -1.000000000000000000, 0.000000000000000000, 0.000000000000000000 ) ) ;
#81403=EDGE_CURVE ( 'NONE', #210865, #255460, #41086, .T. ) ;
#81419=VERTEX_POINT ( 'NONE', #12846 ) ;
#81422=ORIENTED_EDGE ( 'NONE', *, *, #250234, .T. ) ;
#81431=EDGE_CURVE ( 'NONE', #130735, #220463, #54509, .T. ) ;
#81447=CARTESIAN_POINT ( 'NONE',  ( 20.94999999999999574, -1.736257131597395809, -11.56865232901749785 ) ) ;
#81456=CARTESIAN_POINT ( 'NONE',  ( 18.56579813702275317, 10.33025634371522194, -39.08709292826387838 ) ) ;
#81457=CARTESIAN_POINT ( 'NONE',  ( -20.64999999999999858, 4.250000000000000000, -12.25000000000000000 ) ) ;
#81503=CARTESIAN_POINT ( 'NONE',  ( 21.05000000000000071, 5.265981236333658899E-16, -4.300000000000032685 ) ) ;
#81527=EDGE_CURVE ( 'NONE', #137697, #177256, #158777, .T. ) ;
#81536=AXIS2_PLACEMENT_3D ( 'NONE', #27594, #186643, #203621 ) ;
#81567=DIRECTION ( 'NONE',  ( 0.000000000000000000, -1.000000000000000000, -2.891205793294679805E-16 ) ) ;
#81569=CIRCLE ( 'NONE', #198312, 0.09999999999999939493 ) ;
#81632=ORIENTED_EDGE ( 'NONE', *, *, #81403, .T. ) ;
#81664=EDGE_CURVE ( 'NONE', #17135, #113369, #157996, .T. ) ;
#81679=EDGE_LOOP ( 'NONE', ( #14569, #249554 ) ) ;
#81717=CIRCLE ( 'NONE', #164961, 0.1999999999999996503 ) ;
#81719=ORIENTED_EDGE ( 'NONE', *, *, #220050, .T. ) ;
#81731=CARTESIAN_POINT ( 'NONE',  ( -18.59999999999999787, 7.249999999999999112, -21.35000000000000142 ) ) ;
#81739=ORIENTED_EDGE ( 'NONE', *, *, #214664, .F. ) ;
#81750=ORIENTED_EDGE ( 'NONE', *, *, #67911, .T. ) ;
#81759=EDGE_CURVE ( 'NONE', #40685, #214000, #97994, .T. ) ;
#81766=AXIS2_PLACEMENT_3D ( 'NONE', #115402, #54140, #213208 ) ;
#81776=CARTESIAN_POINT ( 'NONE',  ( 22.59999999999999432, 0.1008583690987118475, 11.74956712348939547 ) ) ;
#81791=DIRECTION ( 'NONE',  ( 0.000000000000000000, 1.000000000000000000, 0.000000000000000000 ) ) ;
#81792=VECTOR ( 'NONE', #83893, 1000.000000000000000 ) ;
#81813=CIRCLE ( 'NONE', #36077, 0.09999999999999939493 ) ;
#81816=ORIENTED_EDGE ( 'NONE', *, *, #10764, .F. ) ;
#81829=DIRECTION ( 'NONE',  ( 1.000000000000000000, 0.000000000000000000, 0.000000000000000000 ) ) ;
#81852=DIRECTION ( 'NONE',  ( 0.000000000000000000, 0.000000000000000000, -1.000000000000000000 ) ) ;
#81855=VECTOR ( 'NONE', #159254, 1000.000000000000000 ) ;
#81858=ORIENTED_EDGE ( 'NONE', *, *, #158963, .F. ) ;
#81860=ADVANCED_FACE ( 'NONE', ( #232846 ), #136210, .F. ) ;
#81873=CARTESIAN_POINT ( 'NONE',  ( 23.14999999999999503, 11.65000000000000746, -12.15000000000000036 ) ) ;
#81874=DIRECTION ( 'NONE',  ( 0.000000000000000000, 0.000000000000000000, -1.000000000000000000 ) ) ;
#81890=DIRECTION ( 'NONE',  ( -1.000000000000000000, 0.000000000000000000, 0.000000000000000000 ) ) ;
#81905=ORIENTED_EDGE ( 'NONE', *, *, #234578, .F. ) ;
#81953=CARTESIAN_POINT ( 'NONE',  ( 20.50589344625226929, 10.48318793147603145, -7.572994978672304534 ) ) ;
#81966=DIRECTION ( 'NONE',  ( 0.000000000000000000, 0.000000000000000000, 1.000000000000000000 ) ) ;
#81985=DIRECTION ( 'NONE',  ( 0.000000000000000000, 0.9876197685951252359, -0.1568667991644863424 ) ) ;
#81993=VERTEX_POINT ( 'NONE', #80131 ) ;
#82019=ORIENTED_EDGE ( 'NONE', *, *, #164477, .F. ) ;
#82043=DIRECTION ( 'NONE',  ( 0.000000000000000000, 0.000000000000000000, -1.000000000000000000 ) ) ;
#82044=CARTESIAN_POINT ( 'NONE',  ( 23.14999999999999858, 0.000000000000000000, -33.50000000000000000 ) ) ;
#82066=ADVANCED_FACE ( 'NONE', ( #83973 ), #112355, .F. ) ;
#82113=ORIENTED_EDGE ( 'NONE', *, *, #226088, .T. ) ;
#82126=AXIS2_PLACEMENT_3D ( 'NONE', #36380, #37658, #257908 ) ;
#82144=DIRECTION ( 'NONE',  ( 0.000000000000000000, 0.000000000000000000, 1.000000000000000000 ) ) ;
#82154=B_SPLINE_CURVE_WITH_KNOTS ( 'NONE', 3,
 ( #226854, #69087, #209874, #49508, #243847, #206016, #48216, #130309, #26105, #105594 ),
 .UNSPECIFIED., .F., .F.,
 ( 4, 3, 3, 4 ),
 ( 0.000000000000000000, 0.0002000000000008585893, 0.001000000000082977483, 0.001967863649483336721 ),
 .UNSPECIFIED. ) ;
#82159=ORIENTED_EDGE ( 'NONE', *, *, #130853, .F. ) ;
#82175=( BOUNDED_SURFACE ( )  B_SPLINE_SURFACE ( 3, 2, ( 
 ( #158813, #19273, #81776 ),
 ( #98766, #178374, #238311 ),
 ( #239613, #59650, #218734 ),
 ( #179648, #953, #140486 ) ),
 .UNSPECIFIED., .F., .F., .F. ) 
 B_SPLINE_SURFACE_WITH_KNOTS ( ( 4, 4 ),
 ( 3, 3 ),
 ( -2.710505431213761085E-20, 0.0003124336600439507920 ),
 ( 0.000000000000000000, 1.000000000000000000 ),
 .UNSPECIFIED. ) 
 GEOMETRIC_REPRESENTATION_ITEM ( )  RATIONAL_B_SPLINE_SURFACE ( (
 ( 1.000000000000000000, 0.7071067811865536790, 1.000000000000000000),
 ( 1.000000000000000000, 0.7089187706049598914, 1.000000000000000000),
 ( 1.000000000000000000, 0.7039288185052290370, 1.000000000000000000),
 ( 1.000000000000000000, 0.7040654476015686392, 1.000000000000000000) ) ) 
 REPRESENTATION_ITEM ( '' )  SURFACE ( )  );
#82177=EDGE_CURVE ( 'NONE', #81993, #250275, #199667, .T. ) ;
#82183=EDGE_LOOP ( 'NONE', ( #18324, #218962 ) ) ;
#82202=DIRECTION ( 'NONE',  ( 1.000000000000000000, -0.000000000000000000, 0.000000000000000000 ) ) ;
#82212=ORIENTED_EDGE ( 'NONE', *, *, #150686, .F. ) ;
#82224=AXIS2_PLACEMENT_3D ( 'NONE', #200787, #78255, #221604 ) ;
#82227=ORIENTED_EDGE ( 'NONE', *, *, #193579, .F. ) ;
#82233=ORIENTED_EDGE ( 'NONE', *, *, #45262, .T. ) ;
#82236=CIRCLE ( 'NONE', #103098, 0.09999999999999982514 ) ;
#82238=DIRECTION ( 'NONE',  ( 0.000000000000000000, 0.000000000000000000, -1.000000000000000000 ) ) ;
#82257=ORIENTED_EDGE ( 'NONE', *, *, #23368, .F. ) ;
#82277=AXIS2_PLACEMENT_3D ( 'NONE', #34016, #69265, #130495 ) ;
#82279=CARTESIAN_POINT ( 'NONE',  ( 20.94999999999999574, -11.39257802170567224, -3.073949579831933843 ) ) ;
#82310=EDGE_CURVE ( 'NONE', #69230, #167893, #54240, .T. ) ;
#82315=CIRCLE ( 'NONE', #7512, 0.1000000000000028644 ) ;
#82324=CARTESIAN_POINT ( 'NONE',  ( 21.14999999999999858, 0.000000000000000000, 6.540656951701244282 ) ) ;
#82329=EDGE_CURVE ( 'NONE', #37872, #152840, #129100, .T. ) ;
#82350=CARTESIAN_POINT ( 'NONE',  ( -18.47140463609786920, -9.671474685220882606, -40.17276045827407671 ) ) ;
#82367=FACE_OUTER_BOUND ( 'NONE', #239029, .T. ) ;
#82416=CARTESIAN_POINT ( 'NONE',  ( -20.86777300164945004, 10.33200063079656417, -39.09316749566428939 ) ) ;
#82435=CIRCLE ( 'NONE', #32439, 6.258578643762700899 ) ;
#82463=CARTESIAN_POINT ( 'NONE',  ( 23.15000000000000213, -9.600000000000001421, -9.893969122652443104 ) ) ;
#82488=DIRECTION ( 'NONE',  ( 0.000000000000000000, -1.000000000000000000, 0.000000000000000000 ) ) ;
#82492=VERTEX_POINT ( 'NONE', #105829 ) ;
#82516=ORIENTED_EDGE ( 'NONE', *, *, #77688, .T. ) ;
#82571=DIRECTION ( 'NONE',  ( 1.000000000000000000, 0.000000000000000000, 0.000000000000000000 ) ) ;
#82580=VERTEX_POINT ( 'NONE', #129275 ) ;
#82599=CARTESIAN_POINT ( 'NONE',  ( -20.94999999999999929, 11.74999999999999289, -26.71613433702190576 ) ) ;
#82617=CARTESIAN_POINT ( 'NONE',  ( -23.25000000000000000, 0.000000000000000000, -41.40000000000000568 ) ) ;
#82637=CIRCLE ( 'NONE', #24442, 1.900000000000005906 ) ;
#82641=FACE_OUTER_BOUND ( 'NONE', #132933, .T. ) ;
#82649=FACE_OUTER_BOUND ( 'NONE', #103718, .T. ) ;
#82662=DIRECTION ( 'NONE',  ( 0.000000000000000000, 0.000000000000000000, 1.000000000000000000 ) ) ;
#82736=CARTESIAN_POINT ( 'NONE',  ( 18.50211644919734866, 10.30207779524869061, -38.98955207167824000 ) ) ;
#82750=CARTESIAN_POINT ( 'NONE',  ( 20.85000000000000142, 0.000000000000000000, -33.50000000000000000 ) ) ;
#82777=EDGE_CURVE ( 'NONE', #166638, #43854, #57416, .T. ) ;
#82782=CARTESIAN_POINT ( 'NONE',  ( 23.24999999999999645, 0.000000000000000000, -33.50000000000000000 ) ) ;
#82796=AXIS2_PLACEMENT_3D ( 'NONE', #213102, #216942, #215656 ) ;
#82800=EDGE_CURVE ( 'NONE', #163039, #17816, #100204, .T. ) ;
#82867=DIRECTION ( 'NONE',  ( 0.000000000000000000, 0.000000000000000000, 1.000000000000000000 ) ) ;
#82870=EDGE_LOOP ( 'NONE', ( #81029, #207852, #51414 ) ) ;
#82874=ORIENTED_EDGE ( 'NONE', *, *, #186790, .F. ) ;
#82882=CARTESIAN_POINT ( 'NONE',  ( 21.05000000000000071, 4.999999999999997335, -12.40526601891309788 ) ) ;
#82899=DIRECTION ( 'NONE',  ( 0.000000000000000000, 0.008583690987124399305, -0.9999631594459055250 ) ) ;
#82915=AXIS2_PLACEMENT_3D ( 'NONE', #112191, #255475, #212567 ) ;
#82922=EDGE_LOOP ( 'NONE', ( #78953, #130223, #8185, #187541, #38093 ) ) ;
#82931=LINE ( 'NONE', #119545, #170139 ) ;
#82963=EDGE_CURVE ( 'NONE', #214167, #127799, #104479, .T. ) ;
#82966=EDGE_CURVE ( 'NONE', #55509, #26533, #231589, .T. ) ;
#82969=DIRECTION ( 'NONE',  ( 0.000000000000000000, 0.000000000000000000, -1.000000000000000000 ) ) ;
#82996=ADVANCED_FACE ( 'NONE', ( #153373 ), #174216, .F. ) ;
#83011=FACE_OUTER_BOUND ( 'NONE', #85420, .T. ) ;
#83025=CARTESIAN_POINT ( 'NONE',  ( 21.07954763557440359, 6.329290990037726772, 0.06587591861843060392 ) ) ;
#83037=ORIENTED_EDGE ( 'NONE', *, *, #230464, .T. ) ;
#83042=CARTESIAN_POINT ( 'NONE',  ( 21.07928932188134041, 0.09889514565463336515, 6.328516656398708307 ) ) ;
#83054=DIRECTION ( 'NONE',  ( 0.000000000000000000, 0.000000000000000000, 1.000000000000000000 ) ) ;
#83055=CARTESIAN_POINT ( 'NONE',  ( -20.64999999999999858, 4.349999999999999645, -21.15000000000000213 ) ) ;
#83057=ORIENTED_EDGE ( 'NONE', *, *, #183956, .T. ) ;
#83059=CARTESIAN_POINT ( 'NONE',  ( 20.94999999999999574, -1.835341550224411922, -11.65515129256297833 ) ) ;
#83064=DIRECTION ( 'NONE',  ( 0.000000000000000000, -0.1455152366551522025, -0.9893560106964505163 ) ) ;
#83065=AXIS2_PLACEMENT_3D ( 'NONE', #4477, #206544, #27943 ) ;
#83068=VERTEX_POINT ( 'NONE', #52933 ) ;
#83072=CIRCLE ( 'NONE', #74797, 0.1000000000000028644 ) ;
#83091=TOROIDAL_SURFACE ( 'NONE', #208055, 0.2000000000000000111, 0.1000000000000000056 ) ;
#83092=DIRECTION ( 'NONE',  ( 1.000000000000000000, -0.000000000000000000, -0.000000000000000000 ) ) ;
#83098=EDGE_LOOP ( 'NONE', ( #25438, #48912, #9554, #253137 ) ) ;
#83118=ORIENTED_EDGE ( 'NONE', *, *, #57836, .T. ) ;
#83141=ORIENTED_EDGE ( 'NONE', *, *, #163657, .F. ) ;
#83153=DIRECTION ( 'NONE',  ( -3.265361837132813093E-16, 1.000000000000000000, 0.000000000000000000 ) ) ;
#83165=ORIENTED_EDGE ( 'NONE', *, *, #106189, .F. ) ;
#83181=EDGE_CURVE ( 'NONE', #179010, #38660, #180598, .T. ) ;
#83260=CARTESIAN_POINT ( 'NONE',  ( -18.59999999999999787, 1.851028230140860487, -11.65391326942249250 ) ) ;
#83267=LINE ( 'NONE', #162861, #107141 ) ;
#83273=CARTESIAN_POINT ( 'NONE',  ( 18.59999999999999076, 10.20857864376269575, -24.75000000000000000 ) ) ;
#83311=FACE_OUTER_BOUND ( 'NONE', #188611, .T. ) ;
#83327=CARTESIAN_POINT ( 'NONE',  ( 22.00411653962170533, 7.253442868370061802, 0.09903810578604116399 ) ) ;
#83355=CARTESIAN_POINT ( 'NONE',  ( -20.54999999999999716, 1.940186915887848196, -20.67088078894667547 ) ) ;
#83363=ADVANCED_FACE ( 'NONE', ( #113900 ), #170822, .T. ) ;
#83369=CARTESIAN_POINT ( 'NONE',  ( 23.15000000000000213, -11.64999999999999147, -30.39999999999999503 ) ) ;
#83384=EDGE_LOOP ( 'NONE', ( #79815, #57929, #146947, #20563 ) ) ;
#83400=ORIENTED_EDGE ( 'NONE', *, *, #111425, .F. ) ;
#83406=PLANE ( 'NONE',  #120497 ) ;
#83417=DIRECTION ( 'NONE',  ( 0.000000000000000000, 2.891205793294679805E-16, -1.000000000000000000 ) ) ;
#83432=DIRECTION ( 'NONE',  ( 2.342056488767301376E-15, -0.1350103645451904977, -0.9908441862701596881 ) ) ;
#83451=ORIENTED_EDGE ( 'NONE', *, *, #166967, .T. ) ;
#83454=CIRCLE ( 'NONE', #8481, 12.87499999999999822 ) ;
#83477=EDGE_CURVE ( 'NONE', #183242, #210699, #116597, .T. ) ;
#83492=FACE_OUTER_BOUND ( 'NONE', #204746, .T. ) ;
#83509=EDGE_LOOP ( 'NONE', ( #139433, #146226, #9403, #7720 ) ) ;
#83525=ORIENTED_EDGE ( 'NONE', *, *, #144375, .T. ) ;
#83571=DIRECTION ( 'NONE',  ( -0.000000000000000000, -0.000000000000000000, -1.000000000000000000 ) ) ;
#83627=CIRCLE ( 'NONE', #225292, 0.1000000000000001582 ) ;
#83650=TOROIDAL_SURFACE ( 'NONE', #112907, 0.2000000000000000111, 0.1000000000000000056 ) ;
#83652=CYLINDRICAL_SURFACE ( 'NONE', #67831, 0.09999999999999939493 ) ;
#83683=ORIENTED_EDGE ( 'NONE', *, *, #13825, .F. ) ;
#83687=CARTESIAN_POINT ( 'NONE',  ( -20.94999999999999929, 10.29288807858821109, -38.95800201601217339 ) ) ;
#83709=AXIS2_PLACEMENT_3D ( 'NONE', #167710, #124709, #42599 ) ;
#83800=ADVANCED_FACE ( 'NONE', ( #10653 ), #249270, .T. ) ;
#83832=ORIENTED_EDGE ( 'NONE', *, *, #105148, .T. ) ;
#83833=DIRECTION ( 'NONE',  ( -1.000000000000000000, 0.000000000000000000, 0.000000000000000000 ) ) ;
#83859=EDGE_LOOP ( 'NONE', ( #150168, #194654, #122948, #6514 ) ) ;
#83887=ORIENTED_EDGE ( 'NONE', *, *, #34187, .F. ) ;
#83893=DIRECTION ( 'NONE',  ( 1.000000000000000000, -0.000000000000000000, -0.000000000000000000 ) ) ;
#83925=ORIENTED_EDGE ( 'NONE', *, *, #3645, .T. ) ;
#83928=FACE_OUTER_BOUND ( 'NONE', #21888, .T. ) ;
#83937=DIRECTION ( 'NONE',  ( -1.000000000000000000, -1.836970198721029934E-16, -3.186635328391151676E-31 ) ) ;
#83957=ORIENTED_EDGE ( 'NONE', *, *, #147089, .F. ) ;
#83973=FACE_OUTER_BOUND ( 'NONE', #189589, .T. ) ;
#83974=VERTEX_POINT ( 'NONE', #101702 ) ;
#83984=FACE_OUTER_BOUND ( 'NONE', #65235, .T. ) ;
#83993=EDGE_LOOP ( 'NONE', ( #114946, #169694, #122828 ) ) ;
#83999=ADVANCED_FACE ( 'NONE', ( #26068 ), #142143, .F. ) ;
#84003=CARTESIAN_POINT ( 'NONE',  ( 18.49999999999999289, 10.29270135740183179, -38.95736188715193293 ) ) ;
#84040=CIRCLE ( 'NONE', #155050, 0.09999999999999939493 ) ;
#84043=DIRECTION ( 'NONE',  ( -1.000000000000000000, -0.000000000000000000, -0.000000000000000000 ) ) ;
#84057=DIRECTION ( 'NONE',  ( -0.000000000000000000, -0.000000000000000000, 1.000000000000000000 ) ) ;
#84065=VERTEX_POINT ( 'NONE', #151150 ) ;
#84075=DIRECTION ( 'NONE',  ( 0.000000000000000000, 0.9908441862701596881, -0.1350103645451904977 ) ) ;
#84088=EDGE_LOOP ( 'NONE', ( #120273, #23612, #197410 ) ) ;
#84118=ADVANCED_FACE ( 'NONE', ( #130275 ), #79347, .F. ) ;
#84127=ORIENTED_EDGE ( 'NONE', *, *, #30268, .F. ) ;
#84133=CARTESIAN_POINT ( 'NONE',  ( -20.94999999999999929, 1.851028230140860487, -11.65391326942249250 ) ) ;
#84145=DIRECTION ( 'NONE',  ( 0.000000000000000000, 0.000000000000000000, -1.000000000000000000 ) ) ;
#84155=EDGE_CURVE ( 'NONE', #114284, #177411, #166896, .T. ) ;
#84157=CYLINDRICAL_SURFACE ( 'NONE', #215948, 0.09999999999999939493 ) ;
#84201=CARTESIAN_POINT ( 'NONE',  ( -22.59999999999999787, 0.09999999999999939493, 11.64957080754479968 ) ) ;
#84244=AXIS2_PLACEMENT_3D ( 'NONE', #89806, #208509, #130215 ) ;
#84271=PLANE ( 'NONE',  #93684 ) ;
#84272=CARTESIAN_POINT ( 'NONE',  ( -18.46946985241261174, -9.509317228711573478, -6.986662565499634603 ) ) ;
#84294=AXIS2_PLACEMENT_3D ( 'NONE', #183800, #23478, #104239 ) ;
#84303=CARTESIAN_POINT ( 'NONE',  ( 18.49999999999999289, 11.65000000000000391, -24.85000000000000142 ) ) ;
#84310=DIRECTION ( 'NONE',  ( -1.000000000000000000, 0.000000000000000000, 0.000000000000000000 ) ) ;
#84353=CARTESIAN_POINT ( 'NONE',  ( -20.95613430942416144, 11.75000000000000000, -6.857162648220172407 ) ) ;
#84387=CARTESIAN_POINT ( 'NONE',  ( 23.14999999999999858, 0.000000000000000000, -33.50000000000000000 ) ) ;
#84393=CARTESIAN_POINT ( 'NONE',  ( -20.94999999999999929, -11.29603075033528548, -3.047899159663867152 ) ) ;
#84414=EDGE_CURVE ( 'NONE', #37010, #77399, #108590, .T. ) ;
#84418=ORIENTED_EDGE ( 'NONE', *, *, #48926, .F. ) ;
#84439=DIRECTION ( 'NONE',  ( 0.000000000000000000, 0.000000000000000000, -1.000000000000000000 ) ) ;
#84448=DIRECTION ( 'NONE',  ( -0.000000000000000000, -0.000000000000000000, -1.000000000000000000 ) ) ;
#84457=DIRECTION ( 'NONE',  ( -0.000000000000000000, 0.000000000000000000, 1.000000000000000000 ) ) ;
#84481=DIRECTION ( 'NONE',  ( 1.000000000000000000, 0.000000000000000000, 0.000000000000000000 ) ) ;
#84499=EDGE_LOOP ( 'NONE', ( #192764, #59955, #104590 ) ) ;
#84504=FACE_BOUND ( 'NONE', #82183, .T. ) ;
#84538=DIRECTION ( 'NONE',  ( 0.000000000000000000, 0.000000000000000000, -1.000000000000000000 ) ) ;
#84581=PRODUCT_DEFINITION_SHAPE ( 'NONE', 'NONE',  #163264 ) ;
#84602=DIRECTION ( 'NONE',  ( -1.000000000000000000, -0.000000000000000000, -0.000000000000000000 ) ) ;
#84612=CIRCLE ( 'NONE', #167888, 4.049999999999998934 ) ;
#84624=VECTOR ( 'NONE', #251176, 1000.000000000000114 ) ;
#84634=EDGE_CURVE ( 'NONE', #138502, #191355, #137332, .T. ) ;
#84645=CARTESIAN_POINT ( 'NONE',  ( 21.05000000000000071, -0.09999999999999939493, 6.540656951701244282 ) ) ;
#84666=ORIENTED_EDGE ( 'NONE', *, *, #123595, .F. ) ;
#84692=VERTEX_POINT ( 'NONE', #218148 ) ;
#84700=DIRECTION ( 'NONE',  ( 0.000000000000000000, 0.000000000000000000, -1.000000000000000000 ) ) ;
#84707=CARTESIAN_POINT ( 'NONE',  ( 21.22070241538126467, 0.09891903053502529297, 6.469946272869620429 ) ) ;
#84716=ORIENTED_EDGE ( 'NONE', *, *, #16135, .F. ) ;
#84757=AXIS2_PLACEMENT_3D ( 'NONE', #99250, #161840, #238789 ) ;
#84773=DIRECTION ( 'NONE',  ( 0.000000000000000000, 0.000000000000000000, 1.000000000000000000 ) ) ;
#84803=CARTESIAN_POINT ( 'NONE',  ( -20.54999999999999716, -8.730841121495329205, -9.598074718984332065 ) ) ;
#84822=CIRCLE ( 'NONE', #80739, 0.09999999999999939493 ) ;
#84826=CARTESIAN_POINT ( 'NONE',  ( -22.39999999999999858, 0.000000000000000000, 6.249999999999998224 ) ) ;
#84832=ORIENTED_EDGE ( 'NONE', *, *, #75807, .F. ) ;
#84849=ORIENTED_EDGE ( 'NONE', *, *, #114190, .F. ) ;
#84903=ORIENTED_EDGE ( 'NONE', *, *, #257091, .T. ) ;
#84940=DIRECTION ( 'NONE',  ( 0.000000000000000000, 0.000000000000000000, -1.000000000000000000 ) ) ;
#84943=CARTESIAN_POINT ( 'NONE',  ( -21.05000000000000071, 1.835341550224411922, -11.65515129256298010 ) ) ;
#84969=VERTEX_POINT ( 'NONE', #49368 ) ;
#84973=CARTESIAN_POINT ( 'NONE',  ( -23.15000000000000213, -9.000000000000003553, -9.393969122652443104 ) ) ;
#84981=CARTESIAN_POINT ( 'NONE',  ( -20.85000000000000142, 10.33248238082518711, -39.09484654391314962 ) ) ;
#84984=CARTESIAN_POINT ( 'NONE',  ( -21.29999999999995808, 0.000000000000000000, -4.049999999999998934 ) ) ;
#85001=EDGE_CURVE ( 'NONE', #43854, #3631, #250598, .T. ) ;
#85003=AXIS2_PLACEMENT_3D ( 'NONE', #181302, #83432, #196978 ) ;
#85004=CYLINDRICAL_SURFACE ( 'NONE', #105611, 0.09999999999999939493 ) ;
#85023=B_SPLINE_CURVE_WITH_KNOTS ( 'NONE', 3,
 ( #148417, #106692, #150980, #149718 ),
 .UNSPECIFIED., .F., .F.,
 ( 4, 4 ),
 ( 0.000000000000000000, 0.001767853679387110157 ),
 .UNSPECIFIED. ) ;
#85074=ORIENTED_EDGE ( 'NONE', *, *, #105692, .T. ) ;
#85094=EDGE_CURVE ( 'NONE', #199662, #191690, #764, .T. ) ;
#85116=ADVANCED_FACE ( 'NONE', ( #71520, #209726 ), #92336, .T. ) ;
#85125=DIRECTION ( 'NONE',  ( 1.000000000000000000, 0.000000000000000000, 0.000000000000000000 ) ) ;
#85126=EDGE_CURVE ( 'NONE', #130475, #240172, #246330, .T. ) ;
#85136=ORIENTED_EDGE ( 'NONE', *, *, #92670, .F. ) ;
#85183=AXIS2_PLACEMENT_3D ( 'NONE', #198173, #142047, #221564 ) ;
#85211=ADVANCED_FACE ( 'NONE', ( #51903 ), #191476, .F. ) ;
#85219=CIRCLE ( 'NONE', #151924, 0.09999999999999939493 ) ;
#85246=ORIENTED_EDGE ( 'NONE', *, *, #90372, .T. ) ;
#85258=EDGE_CURVE ( 'NONE', #199652, #183080, #54783, .T. ) ;
#85282=DIRECTION ( 'NONE',  ( 0.000000000000000000, -1.000000000000000000, 0.000000000000000000 ) ) ;
#85329=DIRECTION ( 'NONE',  ( 1.000000000000000000, 7.304098846218134667E-16, 0.000000000000000000 ) ) ;
#85343=VERTEX_POINT ( 'NONE', #118335 ) ;
#85346=AXIS2_PLACEMENT_3D ( 'NONE', #69288, #127968, #87530 ) ;
#85356=ORIENTED_EDGE ( 'NONE', *, *, #129430, .F. ) ;
#85368=CARTESIAN_POINT ( 'NONE',  ( -20.54999999999999716, 7.150000000000000355, -12.34999999999999964 ) ) ;
#85371=DIRECTION ( 'NONE',  ( 0.000000000000000000, 1.000000000000000000, 0.000000000000000000 ) ) ;
#85391=CARTESIAN_POINT ( 'NONE',  ( -20.54999999999999716, 1.999999999999998224, -20.27537807723789953 ) ) ;
#85408=ORIENTED_EDGE ( 'NONE', *, *, #145237, .F. ) ;
#85420=EDGE_LOOP ( 'NONE', ( #46642, #2656, #13949, #209618, #238159 ) ) ;
#85446=ORIENTED_EDGE ( 'NONE', *, *, #95479, .T. ) ;
#85466=EDGE_CURVE ( 'NONE', #75563, #160332, #147008, .T. ) ;
#85469=DIRECTION ( 'NONE',  ( -0.000000000000000000, -0.1350103645451876666, 0.9908441862701600211 ) ) ;
#85472=DIRECTION ( 'NONE',  ( 0.000000000000000000, 0.000000000000000000, -1.000000000000000000 ) ) ;
#85482=AXIS2_PLACEMENT_3D ( 'NONE', #234866, #36694, #56198 ) ;
#85511=ORIENTED_EDGE ( 'NONE', *, *, #226088, .F. ) ;
#85513=FACE_OUTER_BOUND ( 'NONE', #156121, .T. ) ;
#85517=AXIS2_PLACEMENT_3D ( 'NONE', #95675, #134787, #99508 ) ;
#85522=EDGE_CURVE ( 'NONE', #241513, #251180, #213403, .T. ) ;
#85526=EDGE_LOOP ( 'NONE', ( #167870, #196296, #230606, #183637, #16996 ) ) ;
#85528=CARTESIAN_POINT ( 'NONE',  ( 20.94999675878240808, 10.29307482167955357, -38.95864214669402514 ) ) ;
#85545=DIRECTION ( 'NONE',  ( 0.000000000000000000, 0.000000000000000000, -1.000000000000000000 ) ) ;
#85572=CARTESIAN_POINT ( 'NONE',  ( -18.42609945526394455, -9.499999710490698135, -6.999362490248241642 ) ) ;
#85573=CARTESIAN_POINT ( 'NONE',  ( 18.59999999999999076, -1.851617760468904805, -45.10318971960366241 ) ) ;
#85576=EDGE_CURVE ( 'NONE', #41617, #13199, #111755, .T. ) ;
#85583=CARTESIAN_POINT ( 'NONE',  ( -20.94999999999999929, -11.65000000000000036, -2.900000000000003464 ) ) ;
#85665=ORIENTED_EDGE ( 'NONE', *, *, #169308, .F. ) ;
#85707=PLANE ( 'NONE',  #87682 ) ;
#85769=DIRECTION ( 'NONE',  ( 0.000000000000000000, -6.217248937900876626E-15, -1.000000000000000000 ) ) ;
#85773=DIRECTION ( 'NONE',  ( 0.000000000000000000, -0.8660254037844383745, 0.5000000000000003331 ) ) ;
#85797=DIRECTION ( 'NONE',  ( 0.000000000000000000, 0.000000000000000000, -1.000000000000000000 ) ) ;
#85804=DIRECTION ( 'NONE',  ( -0.000000000000000000, 0.000000000000000000, -1.000000000000000000 ) ) ;
#85838=LINE ( 'NONE', #165422, #46002 ) ;
#85841=TOROIDAL_SURFACE ( 'NONE', #60913, 4.149999999999999467, 0.1000000000000000056 ) ;
#85886=ORIENTED_EDGE ( 'NONE', *, *, #201299, .F. ) ;
#85893=CARTESIAN_POINT ( 'NONE',  ( 21.05000000000000071, -11.64999999999999147, 3.469446951953614189E-15 ) ) ;
#85904=AXIS2_PLACEMENT_3D ( 'NONE', #208526, #31199, #186391 ) ;
#85943=ORIENTED_EDGE ( 'NONE', *, *, #130853, .T. ) ;
#85950=DIRECTION ( 'NONE',  ( -0.4999999999999799050, 0.000000000000000000, -0.8660254037844502539 ) ) ;
#85952=DIRECTION ( 'NONE',  ( 0.000000000000000000, 0.000000000000000000, -1.000000000000000000 ) ) ;
#85955=ORIENTED_EDGE ( 'NONE', *, *, #184169, .T. ) ;
#85958=AXIS2_PLACEMENT_3D ( 'NONE', #18257, #97760, #177365 ) ;
#85959=EDGE_CURVE ( 'NONE', #70460, #239230, #46942, .T. ) ;
#85982=DIRECTION ( 'NONE',  ( 2.952720810173289112E-16, -1.000000000000000000, 0.000000000000000000 ) ) ;
#85988=ORIENTED_EDGE ( 'NONE', *, *, #143454, .T. ) ;
#86000=CARTESIAN_POINT ( 'NONE',  ( -20.54999999999999716, -11.75000000000000000, -16.75000000000000000 ) ) ;
#86028=CIRCLE ( 'NONE', #56803, 0.1000000000000002554 ) ;
#86045=DIRECTION ( 'NONE',  ( 0.000000000000000000, 0.000000000000000000, -1.000000000000000000 ) ) ;
#86062=ORIENTED_EDGE ( 'NONE', *, *, #134759, .T. ) ;
#86087=ORIENTED_EDGE ( 'NONE', *, *, #117039, .F. ) ;
#86104=AXIS2_PLACEMENT_3D ( 'NONE', #195567, #252936, #16920 ) ;
#86121=CARTESIAN_POINT ( 'NONE',  ( 18.39999999999999858, -9.399999999999998579, 11.75000000000000000 ) ) ;
#86130=CARTESIAN_POINT ( 'NONE',  ( 18.45068634130096896, -9.486506073342757972, -7.068778431168105669 ) ) ;
#86140=CARTESIAN_POINT ( 'NONE',  ( -21.07928932188134041, 6.328516656398702978, 0.09889514565463444762 ) ) ;
#86144=ADVANCED_FACE ( 'NONE', ( #209938 ), #241661, .T. ) ;
#86231=AXIS2_PLACEMENT_3D ( 'NONE', #236252, #17227, #116325 ) ;
#86274=ADVANCED_FACE ( 'NONE', ( #153854 ), #221906, .F. ) ;
#86278=AXIS2_PLACEMENT_3D ( 'NONE', #59034, #214304, #255937 ) ;
#86297=LINE ( 'NONE', #246674, #238856 ) ;
#86303=ORIENTED_EDGE ( 'NONE', *, *, #22087, .F. ) ;
#86308=ORIENTED_EDGE ( 'NONE', *, *, #163616, .T. ) ;
#86350=TOROIDAL_SURFACE ( 'NONE', #19774, 11.65000000000000036, 0.1000000000000000056 ) ;
#86352=CARTESIAN_POINT ( 'NONE',  ( -18.39999999999999858, -9.500000000000005329, -7.032069396699667685 ) ) ;
#86354=CARTESIAN_POINT ( 'NONE',  ( -20.94999999999999929, 7.021664781900089913, -37.13356540189729316 ) ) ;
#86361=ORIENTED_EDGE ( 'NONE', *, *, #244142, .T. ) ;
#86375=EDGE_CURVE ( 'NONE', #180038, #18766, #117866, .T. ) ;
#86391=DIRECTION ( 'NONE',  ( 0.000000000000000000, 1.000000000000000000, 0.000000000000000000 ) ) ;
#86405=DIRECTION ( 'NONE',  ( -3.265361837132813093E-16, 1.000000000000000000, 0.000000000000000000 ) ) ;
#86406=AXIS2_PLACEMENT_3D ( 'NONE', #43957, #230291, #112923 ) ;
#86450=DIRECTION ( 'NONE',  ( 0.000000000000000000, 0.000000000000000000, -1.000000000000000000 ) ) ;
#86461=ORIENTED_EDGE ( 'NONE', *, *, #14819, .F. ) ;
#86465=AXIS2_PLACEMENT_3D ( 'NONE', #173308, #254059, #93713 ) ;
#86468=ORIENTED_EDGE ( 'NONE', *, *, #234238, .F. ) ;
#86472=DIRECTION ( 'NONE',  ( 0.000000000000000000, -0.1350103645451876666, 0.9908441862701600211 ) ) ;
#86491=VERTEX_POINT ( 'NONE', #105334 ) ;
#86495=DIRECTION ( 'NONE',  ( 0.000000000000000000, -0.9915357197604882655, 0.1298341882519791490 ) ) ;
#86520=ADVANCED_FACE ( 'NONE', ( #7559 ), #166668, .F. ) ;
#86535=EDGE_LOOP ( 'NONE', ( #235490, #232342, #73854, #153059, #47439, #235187, #162390, #189748, #212237, #187725, #207508, #172841, #254869, #112469, #183044, #23200, #251541, #210494, #15332, #192049, #203669, #53660, #114485, #125490, #113147 ) ) ;
#86545=DIRECTION ( 'NONE',  ( -1.000000000000000000, 0.000000000000000000, 0.000000000000000000 ) ) ;
#86556=VECTOR ( 'NONE', #124694, 1000.000000000000000 ) ;
#86582=CARTESIAN_POINT ( 'NONE',  ( -21.05000000000000071, 0.000000000000000000, 0.000000000000000000 ) ) ;
#86595=AXIS2_PLACEMENT_3D ( 'NONE', #35685, #76057, #257213 ) ;
#86647=DIRECTION ( 'NONE',  ( -0.000000000000000000, 0.000000000000000000, -1.000000000000000000 ) ) ;
#86677=( BOUNDED_CURVE ( )  B_SPLINE_CURVE ( 3, ( #14298, #251597, #232054, #18118 ),
 .UNSPECIFIED., .F., .F. ) 
 B_SPLINE_CURVE_WITH_KNOTS ( ( 4, 4 ),
 ( 1.570796326794896558, 3.141592653589793116 ),
 .UNSPECIFIED. ) 
 CURVE ( )  GEOMETRIC_REPRESENTATION_ITEM ( )  RATIONAL_B_SPLINE_CURVE ( ( 1.000000000000000000, 0.8047378541243649375, 0.8047378541243649375, 1.000000000000000000 ) ) 
 REPRESENTATION_ITEM ( '' )  );
#86680=EDGE_CURVE ( 'NONE', #60900, #147515, #197163, .T. ) ;
#86692=EDGE_LOOP ( 'NONE', ( #120829, #122108, #334, #49214, #225896, #131006 ) ) ;
#86698=ORIENTED_EDGE ( 'NONE', *, *, #195095, .T. ) ;
#86783=EDGE_CURVE ( 'NONE', #55133, #213315, #109673, .T. ) ;
#86796=DIRECTION ( 'NONE',  ( 0.000000000000000000, 1.000000000000000000, 0.000000000000000000 ) ) ;
#86817=CARTESIAN_POINT ( 'NONE',  ( 20.94999999999999929, 0.000000000000000000, -33.50000000000000000 ) ) ;
#86854=DIRECTION ( 'NONE',  ( 1.000000000000000000, 0.000000000000000000, 0.000000000000000000 ) ) ;
#86859=CARTESIAN_POINT ( 'NONE',  ( -21.05000000000000071, -1.249999999999999334, -8.000000000000000000 ) ) ;
#86879=CARTESIAN_POINT ( 'NONE',  ( 18.46905048506369695, -9.473744257382394451, -40.17598629225540208 ) ) ;
#86894=CIRCLE ( 'NONE', #75055, 0.09999999999999939493 ) ;
#86903=AXIS2_PLACEMENT_3D ( 'NONE', #132964, #149964, #228206 ) ;
#86957=VERTEX_POINT ( 'NONE', #98603 ) ;
#86973=EDGE_CURVE ( 'NONE', #244742, #127799, #97367, .T. ) ;
#86981=ORIENTED_EDGE ( 'NONE', *, *, #116517, .F. ) ;
#87012=DIRECTION ( 'NONE',  ( 0.000000000000000000, -6.308085367188393199E-16, -1.000000000000000000 ) ) ;
#87027=ORIENTED_EDGE ( 'NONE', *, *, #226142, .T. ) ;
#87030=CYLINDRICAL_SURFACE ( 'NONE', #16185, 0.09999999999999939493 ) ;
#87037=EDGE_LOOP ( 'NONE', ( #14618, #89137, #139610, #174531 ) ) ;
#87042=VECTOR ( 'NONE', #238621, 1000.000000000000000 ) ;
#87050=CARTESIAN_POINT ( 'NONE',  ( -20.64999999999999858, 2.399999999999999467, -20.27537807723789953 ) ) ;
#87081=DIRECTION ( 'NONE',  ( 0.000000000000000000, -0.01283462868041981321, -0.9999176327611367654 ) ) ;
#87124=DIRECTION ( 'NONE',  ( 0.000000000000000000, 0.3738317757009225195, 0.9274965247785541544 ) ) ;
#87127=ORIENTED_EDGE ( 'NONE', *, *, #34723, .T. ) ;
#87205=CARTESIAN_POINT ( 'NONE',  ( 20.85000000000000142, 0.000000000000000000, -33.50000000000000000 ) ) ;
#87217=AXIS2_PLACEMENT_3D ( 'NONE', #90780, #171659, #29576 ) ;
#87221=AXIS2_PLACEMENT_3D ( 'NONE', #181436, #200984, #43199 ) ;
#87286=AXIS2_PLACEMENT_3D ( 'NONE', #250999, #192339, #252288 ) ;
#87300=CARTESIAN_POINT ( 'NONE',  ( -22.57320508075687115, 11.75000000000000000, -3.083226800830041490E-14 ) ) ;
#87318=CIRCLE ( 'NONE', #195698, 4.049999999999998934 ) ;
#87328=EDGE_LOOP ( 'NONE', ( #130833, #171601, #257495, #115169 ) ) ;
#87330=EDGE_CURVE ( 'NONE', #210865, #127472, #89199, .T. ) ;
#87338=EDGE_LOOP ( 'NONE', ( #121675, #683, #232743, #204093 ) ) ;
#87343=LINE ( 'NONE', #26117, #26201 ) ;
#87351=EDGE_LOOP ( 'NONE', ( #27021, #228580, #55356, #108581 ) ) ;
#87367=EDGE_LOOP ( 'NONE', ( #247677, #112783, #101825, #19045 ) ) ;
#87370=ORIENTED_EDGE ( 'NONE', *, *, #121316, .T. ) ;
#87390=CARTESIAN_POINT ( 'NONE',  ( 18.59999999999999787, -1.249999999999999334, -41.30048075441506938 ) ) ;
#87425=ORIENTED_EDGE ( 'NONE', *, *, #113552, .T. ) ;
#87427=CARTESIAN_POINT ( 'NONE',  ( -21.13422380239050824, -7.589415207398531038E-16, 6.493326514805533911 ) ) ;
#87494=CIRCLE ( 'NONE', #195874, 0.09999999999999939493 ) ;
#87513=( BOUNDED_CURVE ( )  B_SPLINE_CURVE ( 3, ( #179146, #236509, #57860, #117846 ),
 .UNSPECIFIED., .F., .F. ) 
 B_SPLINE_CURVE_WITH_KNOTS ( ( 4, 4 ),
 ( 3.192897208853993085, 4.712388980384689674 ),
 .UNSPECIFIED. ) 
 CURVE ( )  GEOMETRIC_REPRESENTATION_ITEM ( )  RATIONAL_B_SPLINE_CURVE ( ( 1.000000000000000000, 0.8166740347213228279, 0.8166740347213228279, 1.000000000000000000 ) ) 
 REPRESENTATION_ITEM ( '' )  );
#87530=DIRECTION ( 'NONE',  ( 1.000000000000000000, 0.000000000000000000, 0.000000000000000000 ) ) ;
#87532=ADVANCED_FACE ( 'NONE', ( #95469 ), #251976, .T. ) ;
#87567=CARTESIAN_POINT ( 'NONE',  ( 18.59999999999999787, -10.35479209692539548, -27.25654098307376216 ) ) ;
#87594=VERTEX_POINT ( 'NONE', #91625 ) ;
#87595=CARTESIAN_POINT ( 'NONE',  ( -20.94999999999999929, 7.070967871798842452, -37.24656422186831151 ) ) ;
#87604=VECTOR ( 'NONE', #25395, 1000.000000000000000 ) ;
#87609=ORIENTED_EDGE ( 'NONE', *, *, #124061, .T. ) ;
#87610=DIRECTION ( 'NONE',  ( 1.000000000000000000, 0.000000000000000000, 0.000000000000000000 ) ) ;
#87629=CIRCLE ( 'NONE', #250157, 11.75000000000000000 ) ;
#87654=ORIENTED_EDGE ( 'NONE', *, *, #53357, .T. ) ;
#87657=DIRECTION ( 'NONE',  ( 0.000000000000000000, 1.734723475976817507E-14, -1.000000000000000000 ) ) ;
#87665=AXIS2_PLACEMENT_3D ( 'NONE', #146052, #100791, #66535 ) ;
#87680=ORIENTED_EDGE ( 'NONE', *, *, #25799, .F. ) ;
#87682=AXIS2_PLACEMENT_3D ( 'NONE', #66190, #246119, #165287 ) ;
#87697=FACE_OUTER_BOUND ( 'NONE', #183816, .T. ) ;
#87711=DIRECTION ( 'NONE',  ( 0.000000000000000000, -1.000000000000000000, 0.000000000000000000 ) ) ;
#87743=DIRECTION ( 'NONE',  ( -2.952720810173289112E-16, 1.000000000000000000, 0.000000000000000000 ) ) ;
#87744=AXIS2_PLACEMENT_3D ( 'NONE', #148420, #183696, #186264 ) ;
#87788=CARTESIAN_POINT ( 'NONE',  ( 21.00000000000000000, 9.749999999999998224, -21.25000000000000000 ) ) ;
#87829=ORIENTED_EDGE ( 'NONE', *, *, #149191, .F. ) ;
#87841=CARTESIAN_POINT ( 'NONE',  ( 22.57856590037848932, -0.004128330064331048668, 11.75005846267545273 ) ) ;
#87866=VECTOR ( 'NONE', #40885, 999.9999999999998863 ) ;
#87876=CIRCLE ( 'NONE', #50461, 0.1999999999999987899 ) ;
#87991=EDGE_CURVE ( 'NONE', #143019, #143516, #52625, .T. ) ;
#88124=CARTESIAN_POINT ( 'NONE',  ( 23.14999999999999858, 4.999999999999997335, -21.59473398108690390 ) ) ;
#88156=EDGE_CURVE ( 'NONE', #50839, #251180, #98549, .T. ) ;
#88176=AXIS2_PLACEMENT_3D ( 'NONE', #194337, #37829, #153948 ) ;
#88182=CYLINDRICAL_SURFACE ( 'NONE', #9912, 0.09999999999999982514 ) ;
#88204=AXIS2_PLACEMENT_3D ( 'NONE', #110178, #150608, #135838 ) ;
#88249=AXIS2_PLACEMENT_3D ( 'NONE', #65438, #201101, #62874 ) ;
#88270=VERTEX_POINT ( 'NONE', #176659 ) ;
#88274=AXIS2_PLACEMENT_3D ( 'NONE', #206517, #226040, #121854 ) ;
#88289=CARTESIAN_POINT ( 'NONE',  ( -18.59999999999999787, 0.000000000000000000, -33.50000000000000000 ) ) ;
#88315=AXIS2_PLACEMENT_3D ( 'NONE', #71925, #172348, #223576 ) ;
#88343=LINE ( 'NONE', #71400, #103848 ) ;
#88348=DIRECTION ( 'NONE',  ( -1.000000000000000000, -0.000000000000000000, -0.000000000000000000 ) ) ;
#88360=DIRECTION ( 'NONE',  ( 0.000000000000000000, -0.9999176327611369874, 0.01283462868041984617 ) ) ;
#88413=CARTESIAN_POINT ( 'NONE',  ( -18.50000000000000000, 10.29270135740182823, -38.95736188715194714 ) ) ;
#88427=LINE ( 'NONE', #109288, #73379 ) ;
#88445=EDGE_CURVE ( 'NONE', #91362, #1674, #48673, .T. ) ;
#88451=DIRECTION ( 'NONE',  ( 1.000000000000000000, 3.265361837132813093E-16, -0.000000000000000000 ) ) ;
#88467=AXIS2_PLACEMENT_3D ( 'NONE', #31460, #110958, #254299 ) ;
#88478=CARTESIAN_POINT ( 'NONE',  ( -18.40904629823847216, -9.500000000000007105, -40.10018956248171662 ) ) ;
#88494=DIRECTION ( 'NONE',  ( 0.000000000000000000, 0.000000000000000000, 1.000000000000000000 ) ) ;
#88499=ORIENTED_EDGE ( 'NONE', *, *, #146802, .F. ) ;
#88531=CARTESIAN_POINT ( 'NONE',  ( -23.25000000000000000, 4.349999999999999645, -12.15000000000000391 ) ) ;
#88541=ADVANCED_FACE ( 'NONE', ( #235035 ), #233754, .T. ) ;
#88555=ORIENTED_EDGE ( 'NONE', *, *, #191298, .T. ) ;
#88635=CYLINDRICAL_SURFACE ( 'NONE', #6961, 12.87499999999999822 ) ;
#88664=DIRECTION ( 'NONE',  ( 1.000000000000000000, -0.000000000000000000, -0.000000000000000000 ) ) ;
#88671=CARTESIAN_POINT ( 'NONE',  ( -20.54999999999999716, 1.999999999999998224, -20.27537807723789953 ) ) ;
#88687=AXIS2_PLACEMENT_3D ( 'NONE', #17185, #72018, #253199 ) ;
#88715=CARTESIAN_POINT ( 'NONE',  ( -21.05000000000000071, 6.258842723537645369, 0.03201369318776357137 ) ) ;
#88750=DIRECTION ( 'NONE',  ( -0.000000000000000000, 1.000000000000000000, -1.224646799147352961E-16 ) ) ;
#88765=CARTESIAN_POINT ( 'NONE',  ( 21.14999999999999858, 6.257814610476124528, 0.09779029130879343668 ) ) ;
#88777=LINE ( 'NONE', #227021, #211832 ) ;
#88787=FACE_OUTER_BOUND ( 'NONE', #221418, .T. ) ;
#88822=ADVANCED_FACE ( 'NONE', ( #131617 ), #97227, .T. ) ;
#88877=EDGE_LOOP ( 'NONE', ( #173124, #77439 ) ) ;
#88891=AXIS2_PLACEMENT_3D ( 'NONE', #172444, #254471, #154166 ) ;
#88900=DIRECTION ( 'NONE',  ( 0.000000000000000000, 1.000000000000000000, 0.000000000000000000 ) ) ;
#88908=CARTESIAN_POINT ( 'NONE',  ( 23.14999999999999503, 11.65000000000000746, -21.25000000000000000 ) ) ;
#88918=EDGE_LOOP ( 'NONE', ( #196373, #8542, #82159 ) ) ;
#88924=ORIENTED_EDGE ( 'NONE', *, *, #132063, .T. ) ;
#88935=CIRCLE ( 'NONE', #51319, 0.09999999999999939493 ) ;
#88943=VERTEX_POINT ( 'NONE', #201863 ) ;
#88975=FACE_OUTER_BOUND ( 'NONE', #163102, .T. ) ;
#88978=DIRECTION ( 'NONE',  ( 0.000000000000000000, 0.7397360091702755991, -0.6728971962616832059 ) ) ;
#89018=FACE_OUTER_BOUND ( 'NONE', #184187, .T. ) ;
#89057=ORIENTED_EDGE ( 'NONE', *, *, #78356, .T. ) ;
#89079=EDGE_CURVE ( 'NONE', #136601, #134956, #209718, .T. ) ;
#89085=CARTESIAN_POINT ( 'NONE',  ( -20.54999999999999716, 2.399999999999999467, -23.60603087734756045 ) ) ;
#89089=DIRECTION ( 'NONE',  ( 1.000000000000000000, 0.000000000000000000, 0.000000000000000000 ) ) ;
#89092=DIRECTION ( 'NONE',  ( 1.000000000000000000, 0.000000000000000000, 0.000000000000000000 ) ) ;
#89098=CARTESIAN_POINT ( 'NONE',  ( 21.04999999999999716, 10.68430915748508347, -7.526696790326847797 ) ) ;
#89112=FACE_OUTER_BOUND ( 'NONE', #79351, .T. ) ;
#89116=DIRECTION ( 'NONE',  ( 0.000000000000000000, 0.000000000000000000, -1.000000000000000000 ) ) ;
#89137=ORIENTED_EDGE ( 'NONE', *, *, #222477, .F. ) ;
#89142=DIRECTION ( 'NONE',  ( -1.000000000000000000, 0.000000000000000000, 0.000000000000000000 ) ) ;
#89180=AXIS2_PLACEMENT_3D ( 'NONE', #5463, #141162, #21240 ) ;
#89199=CIRCLE ( 'NONE', #47679, 0.4000000000000010214 ) ;
#89207=CARTESIAN_POINT ( 'NONE',  ( -21.05000000000000071, 11.59999999999999964, -26.57179676972449656 ) ) ;
#89220=CARTESIAN_POINT ( 'NONE',  ( 23.14999999999999858, 2.000000000000002665, -33.50000000000000000 ) ) ;
#89244=TOROIDAL_SURFACE ( 'NONE', #235016, 0.6000000000000009770, 0.1000000000000000056 ) ;
#89258=AXIS2_PLACEMENT_3D ( 'NONE', #239139, #194893, #100858 ) ;
#89275=FILL_AREA_STYLE_COLOUR ( '', #106246 ) ;
#89284=AXIS2_PLACEMENT_3D ( 'NONE', #254611, #5413, #161980 ) ;
#89297=DIRECTION ( 'NONE',  ( 0.000000000000000000, 0.01562500000001058528, 0.9998779222360095753 ) ) ;
#89322=DIRECTION ( 'NONE',  ( -1.000000000000000000, -0.000000000000000000, -0.000000000000000000 ) ) ;
#89328=CARTESIAN_POINT ( 'NONE',  ( 18.49999999999998934, 10.24999999999999822, -24.65000000000000213 ) ) ;
#89408=CARTESIAN_POINT ( 'NONE',  ( 20.89192007715127986, 10.32898536000685574, -39.08266832227643306 ) ) ;
#89426=CIRCLE ( 'NONE', #93711, 0.1000000000000000333 ) ;
#89435=VECTOR ( 'NONE', #21092, 1000.000000000000000 ) ;
#89442=CIRCLE ( 'NONE', #235210, 0.09999999999999939493 ) ;
#89452=CARTESIAN_POINT ( 'NONE',  ( -22.50000000000000000, 11.64957080754479968, 0.09999999999999592548 ) ) ;
#89455=DIRECTION ( 'NONE',  ( -0.000000000000000000, -0.1350103645451876666, -0.9908441862701600211 ) ) ;
#89476=ORIENTED_EDGE ( 'NONE', *, *, #73537, .T. ) ;
#89522=CARTESIAN_POINT ( 'NONE',  ( 19.99999999999998934, 11.75000000000000000, -21.35000000000000142 ) ) ;
#89529=CARTESIAN_POINT ( 'NONE',  ( 20.94999999999997442, -1.263275465217258198, -41.40186466674640542 ) ) ;
#89530=EDGE_LOOP ( 'NONE', ( #234268, #84127, #37835, #113989 ) ) ;
#89534=CARTESIAN_POINT ( 'NONE',  ( -20.64999999999999858, 4.349999999999999645, -12.35000000000000142 ) ) ;
#89541=DIRECTION ( 'NONE',  ( 0.000000000000000000, 0.000000000000000000, 1.000000000000000000 ) ) ;
#89570=CARTESIAN_POINT ( 'NONE',  ( -20.00857864376270001, 9.150000000000002132, -12.34999999999999964 ) ) ;
#89575=CIRCLE ( 'NONE', #251901, 11.79999999999999716 ) ;
#89606=VECTOR ( 'NONE', #212740, 1000.000000000000000 ) ;
#89613=EDGE_CURVE ( 'NONE', #122037, #115921, #205547, .T. ) ;
#89616=CARTESIAN_POINT ( 'NONE',  ( 21.05000000000000071, 0.000000000000000000, 0.000000000000000000 ) ) ;
#89621=VERTEX_POINT ( 'NONE', #85573 ) ;
#89637=CARTESIAN_POINT ( 'NONE',  ( -23.25000000000000000, 0.000000000000000000, 0.000000000000000000 ) ) ;
#89639=CARTESIAN_POINT ( 'NONE',  ( -23.15000000000000213, -11.65000000000000036, -30.39999999999999858 ) ) ;
#89676=CARTESIAN_POINT ( 'NONE',  ( 21.10710606213542206, 8.776894023893211383, -12.24099652639942271 ) ) ;
#89686=LINE ( 'NONE', #47999, #407 ) ;
#89696=DIRECTION ( 'NONE',  ( 0.000000000000000000, 0.000000000000000000, -1.000000000000000000 ) ) ;
#89702=CARTESIAN_POINT ( 'NONE',  ( -23.25000000000000000, 7.021664781900089913, -37.33356540189728889 ) ) ;
#89735=CARTESIAN_POINT ( 'NONE',  ( -20.94999999999999929, -0.2561057920922211739, 0.03489644167229202787 ) ) ;
#89762=DIRECTION ( 'NONE',  ( 0.000000000000000000, -1.000000000000000000, 0.000000000000000000 ) ) ;
#89776=CARTESIAN_POINT ( 'NONE',  ( -18.40000000000000213, -9.500000000000007105, -40.42214984933044519 ) ) ;
#89806=CARTESIAN_POINT ( 'NONE',  ( -20.00857864376270001, 9.150000000000002132, -12.25000000000000000 ) ) ;
#89811=DIRECTION ( 'NONE',  ( 0.000000000000000000, 0.000000000000000000, 1.000000000000000000 ) ) ;
#89840=CARTESIAN_POINT ( 'NONE',  ( 20.00000000000000355, 11.75000000000000711, -24.65000000000000213 ) ) ;
#89876=CARTESIAN_POINT ( 'NONE',  ( -20.54999999999999716, -8.730841121495325652, -23.90192528101566793 ) ) ;
#89888=CARTESIAN_POINT ( 'NONE',  ( 18.59999999999999787, -1.851028230140860487, -11.65391326942249250 ) ) ;
#89922=CARTESIAN_POINT ( 'NONE',  ( -20.94999999999999929, 1.162701749938009677, -8.099999999999999645 ) ) ;
#89926=ORIENTED_EDGE ( 'NONE', *, *, #151323, .T. ) ;
#89944=FACE_OUTER_BOUND ( 'NONE', #78132, .T. ) ;
#89948=EDGE_CURVE ( 'NONE', #210671, #138899, #97209, .T. ) ;
#89950=AXIS2_PLACEMENT_3D ( 'NONE', #153947, #35273, #155214 ) ;
#89957=DIRECTION ( 'NONE',  ( 0.000000000000000000, 0.000000000000000000, 1.000000000000000000 ) ) ;
#89960=CARTESIAN_POINT ( 'NONE',  ( 20.94999999999999574, 8.926614585087095932, -8.471683019223121391 ) ) ;
#90002=ORIENTED_EDGE ( 'NONE', *, *, #196554, .T. ) ;
#90012=DIRECTION ( 'NONE',  ( 0.000000000000000000, 0.000000000000000000, -1.000000000000000000 ) ) ;
#90013=DIRECTION ( 'NONE',  ( 0.000000000000000000, 0.000000000000000000, -1.000000000000000000 ) ) ;
#90015=ORIENTED_EDGE ( 'NONE', *, *, #256879, .F. ) ;
#90036=DIRECTION ( 'NONE',  ( -1.000000000000000000, -7.304098846218133681E-16, 4.217023435051677994E-16 ) ) ;
#90064=DIRECTION ( 'NONE',  ( 2.952720810173289112E-16, -1.000000000000000000, 0.000000000000000000 ) ) ;
#90125=CARTESIAN_POINT ( 'NONE',  ( 21.05000000000000071, 5.849999999999949019, -10.13249722427796762 ) ) ;
#90172=AXIS2_PLACEMENT_3D ( 'NONE', #180213, #98052, #2824 ) ;
#90181=DIRECTION ( 'NONE',  ( 0.000000000000000000, -1.000000000000000000, -0.000000000000000000 ) ) ;
#90204=ORIENTED_EDGE ( 'NONE', *, *, #191196, .F. ) ;
#90206=FACE_OUTER_BOUND ( 'NONE', #62372, .T. ) ;
#90208=ADVANCED_FACE ( 'NONE', ( #202071 ), #161679, .T. ) ;
#90238=ORIENTED_EDGE ( 'NONE', *, *, #184356, .T. ) ;
#90245=AXIS2_PLACEMENT_3D ( 'NONE', #51207, #173816, #72105 ) ;
#90250=DIRECTION ( 'NONE',  ( 1.000000000000000000, 3.265361837132813093E-16, -0.000000000000000000 ) ) ;
#90285=AXIS2_PLACEMENT_3D ( 'NONE', #34215, #233680, #253220 ) ;
#90292=DIRECTION ( 'NONE',  ( 0.000000000000000000, 0.000000000000000000, 1.000000000000000000 ) ) ;
#90305=ORIENTED_EDGE ( 'NONE', *, *, #237096, .T. ) ;
#90307=DIRECTION ( 'NONE',  ( 0.000000000000000000, 0.000000000000000000, -1.000000000000000000 ) ) ;
#90310=DIRECTION ( 'NONE',  ( -1.000000000000000000, -0.000000000000000000, -0.000000000000000000 ) ) ;
#90313=CARTESIAN_POINT ( 'NONE',  ( 20.94999999999999929, 1.835341550224413698, -11.55515129256298401 ) ) ;
#90335=VERTEX_POINT ( 'NONE', #250182 ) ;
#90347=EDGE_CURVE ( 'NONE', #10818, #199162, #1578, .T. ) ;
#90369=AXIS2_PLACEMENT_3D ( 'NONE', #96830, #194712, #235103 ) ;
#90372=EDGE_CURVE ( 'NONE', #192073, #175406, #106801, .T. ) ;
#90376=ADVANCED_FACE ( 'NONE', ( #109361 ), #248906, .T. ) ;
#90407=ORIENTED_EDGE ( 'NONE', *, *, #105872, .F. ) ;
#90441=CARTESIAN_POINT ( 'NONE',  ( -20.94999999999999929, -1.162701749938009677, -8.000000000000000000 ) ) ;
#90445=DIRECTION ( 'NONE',  ( 0.000000000000000000, 0.000000000000000000, -1.000000000000000000 ) ) ;
#90483=DIRECTION ( 'NONE',  ( -1.000000000000000000, 0.000000000000000000, 0.000000000000000000 ) ) ;
#90509=ORIENTED_EDGE ( 'NONE', *, *, #156896, .F. ) ;
#90524=VECTOR ( 'NONE', #84448, 1000.000000000000000 ) ;
#90525=EDGE_CURVE ( 'NONE', #68538, #127360, #233207, .T. ) ;
#90550=DIRECTION ( 'NONE',  ( 1.000000000000000000, 0.000000000000000000, 0.000000000000000000 ) ) ;
#90552=ORIENTED_EDGE ( 'NONE', *, *, #100240, .T. ) ;
#90558=SURFACE_STYLE_USAGE ( .BOTH. , #74895 ) ;
#90579=DIRECTION ( 'NONE',  ( -0.000000000000000000, 0.8660254037844411501, 0.4999999999999956701 ) ) ;
#90591=ORIENTED_EDGE ( 'NONE', *, *, #15585, .T. ) ;
#90637=CIRCLE ( 'NONE', #44877, 0.09999999999999939493 ) ;
#90681=ORIENTED_EDGE ( 'NONE', *, *, #250917, .T. ) ;
#90685=AXIS2_PLACEMENT_3D ( 'NONE', #175971, #33921, #113406 ) ;
#90699=DIRECTION ( 'NONE',  ( -1.000000000000000000, 0.000000000000000000, 0.000000000000000000 ) ) ;
#90701=CARTESIAN_POINT ( 'NONE',  ( 21.14999999999999858, 8.786607556600111835, -12.25000000000000000 ) ) ;
#90721=CARTESIAN_POINT ( 'NONE',  ( 22.47071067811865319, 7.720074744498043096, 0.09909245470260744093 ) ) ;
#90755=AXIS2_PLACEMENT_3D ( 'NONE', #146938, #83092, #225187 ) ;
#90758=TOROIDAL_SURFACE ( 'NONE', #128201, 0.2000000000000000111, 0.1000000000000000056 ) ;
#90771=EDGE_CURVE ( 'NONE', #130496, #24262, #122593, .T. ) ;
#90773=DIRECTION ( 'NONE',  ( 0.000000000000000000, -0.8777080977375132376, 0.4791956752371582251 ) ) ;
#90777=DIRECTION ( 'NONE',  ( -0.000000000000000000, 0.01283462868039629209, -0.9999176327611372095 ) ) ;
#90780=CARTESIAN_POINT ( 'NONE',  ( -21.45000000000000284, 7.708578643762696636, -21.15000000000000213 ) ) ;
#90788=AXIS2_PLACEMENT_3D ( 'NONE', #148950, #129367, #208901 ) ;
#90791=ADVANCED_FACE ( 'NONE', ( #26995 ), #249865, .F. ) ;
#90826=TOROIDAL_SURFACE ( 'NONE', #236569, 0.6000000000000017542, 0.1000000000000000056 ) ;
#90850=ORIENTED_EDGE ( 'NONE', *, *, #163109, .T. ) ;
#90902=CARTESIAN_POINT ( 'NONE',  ( 21.05000000000000071, 0.000000000000000000, 0.000000000000000000 ) ) ;
#90915=ORIENTED_EDGE ( 'NONE', *, *, #193075, .T. ) ;
#90948=B_SPLINE_CURVE_WITH_KNOTS ( 'NONE', 3,
 ( #42643, #186008, #7364, #123470, #86879, #103877, #3504, #183451, #166477, #245989 ),
 .UNSPECIFIED., .F., .F.,
 ( 4, 2, 2, 2, 4 ),
 ( 0.000000000000000000, 0.0001660831991682258321, 0.0002491247987523387752, 0.0002906455985443952197, 0.0003321663983364516641 ),
 .UNSPECIFIED. ) ;
#90953=EDGE_LOOP ( 'NONE', ( #82516, #95895, #102744, #167968, #133903, #167596, #57451, #241078 ) ) ;
#90989=VERTEX_POINT ( 'NONE', #102307 ) ;
#91006=EDGE_CURVE ( 'NONE', #239652, #96700, #22825, .T. ) ;
#91008=DIRECTION ( 'NONE',  ( 0.000000000000000000, 0.000000000000000000, -1.000000000000000000 ) ) ;
#91075=CARTESIAN_POINT ( 'NONE',  ( -18.31331870001055862, -9.536294719180791191, -40.36857869098546558 ) ) ;
#91077=DIRECTION ( 'NONE',  ( 0.000000000000000000, 0.7397360091702755991, -0.6728971962616832059 ) ) ;
#91097=CARTESIAN_POINT ( 'NONE',  ( -18.59999999999999787, 11.64999999999999680, -12.25000000000000000 ) ) ;
#91102=DIRECTION ( 'NONE',  ( 1.000000000000000000, 0.000000000000000000, 0.000000000000000000 ) ) ;
#91111=CARTESIAN_POINT ( 'NONE',  ( -23.25000000000000000, 2.600000000000000089, -13.22462192276210224 ) ) ;
#91201=LINE ( 'NONE', #63617, #166852 ) ;
#91204=ORIENTED_EDGE ( 'NONE', *, *, #142740, .F. ) ;
#91279=CARTESIAN_POINT ( 'NONE',  ( -21.55000000000000071, 7.349999999999998757, -12.34999999999999964 ) ) ;
#91288=DIRECTION ( 'NONE',  ( 1.000000000000000000, 0.000000000000000000, 0.000000000000000000 ) ) ;
#91299=ORIENTED_EDGE ( 'NONE', *, *, #104138, .F. ) ;
#91314=CARTESIAN_POINT ( 'NONE',  ( 23.14999999999999858, 0.000000000000000000, -37.50000000000000000 ) ) ;
#91333=AXIS2_PLACEMENT_3D ( 'NONE', #128468, #89322, #210575 ) ;
#91362=VERTEX_POINT ( 'NONE', #96870 ) ;
#91366=DIRECTION ( 'NONE',  ( 0.5000000000001141309, 0.000000000000000000, -0.8660254037843729824 ) ) ;
#91411=AXIS2_PLACEMENT_3D ( 'NONE', #193595, #124964, #204478 ) ;
#91419=LINE ( 'NONE', #249210, #24411 ) ;
#91523=EDGE_CURVE ( 'NONE', #112086, #56955, #6411, .T. ) ;
#91546=ORIENTED_EDGE ( 'NONE', *, *, #59474, .T. ) ;
#91559=VERTEX_POINT ( 'NONE', #75465 ) ;
#91599=DIRECTION ( 'NONE',  ( 0.000000000000000000, -1.734723475976811630E-15, 1.000000000000000000 ) ) ;
#91614=VECTOR ( 'NONE', #189316, 1000.000000000000000 ) ;
#91625=CARTESIAN_POINT ( 'NONE',  ( 18.49999999999999645, 1.162701749938009677, -8.099999999999999645 ) ) ;
#91636=ORIENTED_EDGE ( 'NONE', *, *, #183118, .T. ) ;
#91649=CARTESIAN_POINT ( 'NONE',  ( 23.24999999999999645, 4.775700934579435675, -21.65123189595403375 ) ) ;
#91667=ORIENTED_EDGE ( 'NONE', *, *, #100010, .F. ) ;
#91694=EDGE_LOOP ( 'NONE', ( #73902, #129315, #96217, #221451 ) ) ;
#91713=PLANE ( 'NONE',  #158303 ) ;
#91721=CYLINDRICAL_SURFACE ( 'NONE', #224751, 0.1000000000000010741 ) ;
#91731=ORIENTED_EDGE ( 'NONE', *, *, #110604, .F. ) ;
#91746=CARTESIAN_POINT ( 'NONE',  ( 21.05000000000000071, 5.850000000000001421, -23.36750277572207679 ) ) ;
#91804=PLANE ( 'NONE',  #22297 ) ;
#91815=ORIENTED_EDGE ( 'NONE', *, *, #41500, .T. ) ;
#91816=ORIENTED_EDGE ( 'NONE', *, *, #35266, .T. ) ;
#91822=CARTESIAN_POINT ( 'NONE',  ( 20.94999999999999574, 1.736257131597397585, -11.56865232901749962 ) ) ;
#91823=VECTOR ( 'NONE', #93859, 1000.000000000000000 ) ;
#91828=ORIENTED_EDGE ( 'NONE', *, *, #173945, .T. ) ;
#91831=EDGE_LOOP ( 'NONE', ( #96308, #124167, #3959, #69893, #40642 ) ) ;
#91886=FILL_AREA_STYLE_COLOUR ( '', #189328 ) ;
#91911=DIRECTION ( 'NONE',  ( -1.000000000000000000, -0.000000000000000000, -0.000000000000000000 ) ) ;
#91956=DIRECTION ( 'NONE',  ( 0.000000000000000000, 0.000000000000000000, -1.000000000000000000 ) ) ;
#91965=SPHERICAL_SURFACE ( 'NONE', #57566, 0.1000000000000000056 ) ;
#91984=DIRECTION ( 'NONE',  ( 1.000000000000000000, 3.265361837132813093E-16, -0.000000000000000000 ) ) ;
#91988=CARTESIAN_POINT ( 'NONE',  ( 21.13461538461538325, 8.885417037974457699, -12.25000000000000178 ) ) ;
#92091=CARTESIAN_POINT ( 'NONE',  ( -21.05000000000000071, -1.835341550224411922, -11.55515129256297868 ) ) ;
#92099=DIRECTION ( 'NONE',  ( 1.000000000000000000, 0.000000000000000000, 0.000000000000000000 ) ) ;
#92102=EDGE_CURVE ( 'NONE', #144164, #39469, #201473, .T. ) ;
#92123=EDGE_CURVE ( 'NONE', #185054, #34317, #240613, .T. ) ;
#92153=VERTEX_POINT ( 'NONE', #81503 ) ;
#92159=FACE_OUTER_BOUND ( 'NONE', #112362, .T. ) ;
#92199=DIRECTION ( 'NONE',  ( 0.000000000000000000, 0.1350103645451876666, -0.9908441862701600211 ) ) ;
#92216=AXIS2_PLACEMENT_3D ( 'NONE', #248503, #12480, #211960 ) ;
#92225=FACE_OUTER_BOUND ( 'NONE', #55678, .T. ) ;
#92252=ORIENTED_EDGE ( 'NONE', *, *, #129217, .T. ) ;
#92282=CARTESIAN_POINT ( 'NONE',  ( 20.94999999999999929, 1.360870587192041681, -8.072997927090961312 ) ) ;
#92318=ADVANCED_FACE ( 'NONE', ( #130937 ), #248216, .T. ) ;
#92327=EDGE_CURVE ( 'NONE', #105990, #201752, #244099, .T. ) ;
#92333=EDGE_CURVE ( 'NONE', #74587, #39052, #164994, .T. ) ;
#92336=PLANE ( 'NONE',  #179706 ) ;
#92389=DIRECTION ( 'NONE',  ( 1.224646799147353207E-16, 1.000000000000000000, 0.000000000000000000 ) ) ;
#92390=DIRECTION ( 'NONE',  ( -1.000000000000000000, -2.952720810173289112E-16, 0.000000000000000000 ) ) ;
#92391=CARTESIAN_POINT ( 'NONE',  ( 18.45036689428341603, -9.490184143328932009, -7.012695827486270517 ) ) ;
#92395=EDGE_CURVE ( 'NONE', #8515, #218249, #81569, .T. ) ;
#92470=ORIENTED_EDGE ( 'NONE', *, *, #182763, .T. ) ;
#92487=CARTESIAN_POINT ( 'NONE',  ( -20.85000000000000142, 0.000000000000000000, -33.50000000000000000 ) ) ;
#92507=DIRECTION ( 'NONE',  ( -1.000000000000000000, 0.000000000000000000, 0.000000000000000000 ) ) ;
#92517=FACE_OUTER_BOUND ( 'NONE', #129434, .T. ) ;
#92519=ORIENTED_EDGE ( 'NONE', *, *, #157772, .F. ) ;
#92555=CARTESIAN_POINT ( 'NONE',  ( 22.45301702632625762, 0.01521087971018478258, 11.64979222426039129 ) ) ;
#92655=PLANE ( 'NONE',  #36561 ) ;
#92657=DIRECTION ( 'NONE',  ( 0.000000000000000000, 0.000000000000000000, 1.000000000000000000 ) ) ;
#92664=CYLINDRICAL_SURFACE ( 'NONE', #2055, 0.09999999999999939493 ) ;
#92670=EDGE_CURVE ( 'NONE', #176398, #207698, #111016, .T. ) ;
#92682=CARTESIAN_POINT ( 'NONE',  ( -21.37071067811865532, 8.070710678118656389, -12.25000000000000000 ) ) ;
#92698=CARTESIAN_POINT ( 'NONE',  ( 21.05000000000000071, 1.162701749938009677, -7.900000000000000355 ) ) ;
#92712=ORIENTED_EDGE ( 'NONE', *, *, #140603, .F. ) ;
#92736=CARTESIAN_POINT ( 'NONE',  ( -21.07928932188134041, 6.328516656393293083, 0.09889514565439641580 ) ) ;
#92749=EDGE_CURVE ( 'NONE', #193752, #241011, #215071, .T. ) ;
#92767=AXIS2_PLACEMENT_3D ( 'NONE', #71167, #230218, #169008 ) ;
#92782=ORIENTED_EDGE ( 'NONE', *, *, #82966, .F. ) ;
#92792=EDGE_CURVE ( 'NONE', #97347, #187076, #244460, .T. ) ;
#92793=CIRCLE ( 'NONE', #134478, 0.09999999999999939493 ) ;
#92811=ORIENTED_EDGE ( 'NONE', *, *, #166741, .F. ) ;
#92825=VECTOR ( 'NONE', #238060, 1000.000000000000000 ) ;
#92858=ORIENTED_EDGE ( 'NONE', *, *, #253602, .F. ) ;
#92904=EDGE_CURVE ( 'NONE', #235552, #157226, #184939, .T. ) ;
#92921=CARTESIAN_POINT ( 'NONE',  ( 20.95512820512820440, 10.62384868371188062, -7.664913569087605794 ) ) ;
#92941=ORIENTED_EDGE ( 'NONE', *, *, #125791, .F. ) ;
#92952=LINE ( 'NONE', #154267, #2913 ) ;
#92976=VERTEX_POINT ( 'NONE', #29754 ) ;
#92983=AXIS2_PLACEMENT_3D ( 'NONE', #39665, #61763, #119178 ) ;
#93007=ORIENTED_EDGE ( 'NONE', *, *, #119588, .F. ) ;
#93018=CARTESIAN_POINT ( 'NONE',  ( -20.64999999999999858, -8.663551401869156621, -23.97589888193269658 ) ) ;
#93099=AXIS2_PLACEMENT_3D ( 'NONE', #239685, #101398, #23228 ) ;
#93125=CARTESIAN_POINT ( 'NONE',  ( -21.05000000000000071, 0.000000000000000000, 0.000000000000000000 ) ) ;
#93166=CARTESIAN_POINT ( 'NONE',  ( -23.15000000000000213, 4.250000000000000000, -21.25000000000000000 ) ) ;
#93175=VERTEX_POINT ( 'NONE', #239479 ) ;
#93178=ADVANCED_FACE ( 'NONE', ( #19136 ), #94618, .T. ) ;
#93225=CARTESIAN_POINT ( 'NONE',  ( -1.739115166359751801E-14, 11.64999999999998970, -21.35000000000000142 ) ) ;
#93251=ORIENTED_EDGE ( 'NONE', *, *, #220287, .T. ) ;
#93276=DIRECTION ( 'NONE',  ( 1.000000000000000000, 0.000000000000000000, 0.000000000000000000 ) ) ;
#93277=DIRECTION ( 'NONE',  ( 0.000000000000000000, 0.000000000000000000, 1.000000000000000000 ) ) ;
#93287=ORIENTED_EDGE ( 'NONE', *, *, #167746, .F. ) ;
#93288=CIRCLE ( 'NONE', #239042, 0.09999999999999939493 ) ;
#93300=DIRECTION ( 'NONE',  ( -1.000000000000000000, -0.000000000000000000, -0.000000000000000000 ) ) ;
#93325=DIRECTION ( 'NONE',  ( 1.000000000000000000, 0.000000000000000000, 0.000000000000000000 ) ) ;
#93344=DIRECTION ( 'NONE',  ( 0.000000000000000000, 0.000000000000000000, -1.000000000000000000 ) ) ;
#93350=DIRECTION ( 'NONE',  ( 0.000000000000000000, 0.000000000000000000, -1.000000000000000000 ) ) ;
#93352=DIRECTION ( 'NONE',  ( 0.000000000000000000, 0.000000000000000000, 1.000000000000000000 ) ) ;
#93382=CIRCLE ( 'NONE', #168469, 0.1000000000000028644 ) ;
#93404=CARTESIAN_POINT ( 'NONE',  ( 22.00411653889210584, 0.09903810578593504055, 7.253442867640402802 ) ) ;
#93420=EDGE_LOOP ( 'NONE', ( #9048, #232682, #63696, #103771 ) ) ;
#93430=ORIENTED_EDGE ( 'NONE', *, *, #47518, .T. ) ;
#93444=EDGE_LOOP ( 'NONE', ( #11407, #131800, #222728, #161763 ) ) ;
#93448=VECTOR ( 'NONE', #212691, 1000.000000000000000 ) ;
#93449=CARTESIAN_POINT ( 'NONE',  ( 21.05000000000000071, -9.500000000000000000, -23.60603087734755690 ) ) ;
#93491=FACE_OUTER_BOUND ( 'NONE', #154633, .T. ) ;
#93492=CARTESIAN_POINT ( 'NONE',  ( -21.56666275994539816, 0.000000000000000000, 6.957368406893326807 ) ) ;
#93564=ORIENTED_EDGE ( 'NONE', *, *, #67140, .T. ) ;
#93565=FACE_OUTER_BOUND ( 'NONE', #178822, .T. ) ;
#93584=EDGE_CURVE ( 'NONE', #158172, #97122, #223973, .T. ) ;
#93595=FACE_OUTER_BOUND ( 'NONE', #140760, .T. ) ;
#93612=ADVANCED_FACE ( 'NONE', ( #39707 ), #99067, .F. ) ;
#93619=CIRCLE ( 'NONE', #251834, 11.65000000000000036 ) ;
#93636=CIRCLE ( 'NONE', #231209, 0.09999999999999939493 ) ;
#93638=ORIENTED_EDGE ( 'NONE', *, *, #115804, .T. ) ;
#93643=DIRECTION ( 'NONE',  ( 0.000000000000000000, 0.6728971962616783209, 0.7397360091702797069 ) ) ;
#93679=ORIENTED_EDGE ( 'NONE', *, *, #9599, .T. ) ;
#93684=AXIS2_PLACEMENT_3D ( 'NONE', #204262, #166469, #6065 ) ;
#93694=ORIENTED_EDGE ( 'NONE', *, *, #20771, .F. ) ;
#93700=CARTESIAN_POINT ( 'NONE',  ( 18.43630871534870508, -9.679800874802955590, -40.16063206798408913 ) ) ;
#93711=AXIS2_PLACEMENT_3D ( 'NONE', #114576, #35077, #234510 ) ;
#93713=DIRECTION ( 'NONE',  ( 0.000000000000000000, 0.000000000000000000, 1.000000000000000000 ) ) ;
#93745=CIRCLE ( 'NONE', #23044, 0.09999999999999954758 ) ;
#93784=LINE ( 'NONE', #155088, #239593 ) ;
#93785=CARTESIAN_POINT ( 'NONE',  ( -20.54999999999999716, -8.663551401869156621, -23.97589888193269658 ) ) ;
#93798=ORIENTED_EDGE ( 'NONE', *, *, #252388, .F. ) ;
#93817=CARTESIAN_POINT ( 'NONE',  ( 23.24999999999999645, 0.000000000000000000, 0.000000000000000000 ) ) ;
#93847=FACE_OUTER_BOUND ( 'NONE', #60520, .T. ) ;
#93859=DIRECTION ( 'NONE',  ( 0.000000000000000000, 0.000000000000000000, -1.000000000000000000 ) ) ;
#93875=FACE_OUTER_BOUND ( 'NONE', #38910, .T. ) ;
#93888=EDGE_CURVE ( 'NONE', #78587, #253474, #65774, .T. ) ;
#93899=ADVANCED_FACE ( 'NONE', ( #167357 ), #246851, .T. ) ;
#93940=EDGE_LOOP ( 'NONE', ( #206748, #79394, #127450, #186183 ) ) ;
#93976=CIRCLE ( 'NONE', #173149, 11.65000000000000036 ) ;
#93984=CYLINDRICAL_SURFACE ( 'NONE', #155819, 0.09999999999999976963 ) ;
#94047=DIRECTION ( 'NONE',  ( 0.000000000000000000, 0.000000000000000000, -1.000000000000000000 ) ) ;
#94064=CARTESIAN_POINT ( 'NONE',  ( -20.85000000000000142, 7.021664781900089913, -37.33356540189728889 ) ) ;
#94088=DIRECTION ( 'NONE',  ( 0.000000000000000000, 0.000000000000000000, 1.000000000000000000 ) ) ;
#94108=DIRECTION ( 'NONE',  ( 1.000000000000000000, -0.000000000000000000, -0.000000000000000000 ) ) ;
#94126=ADVANCED_FACE ( 'NONE', ( #141051 ), #62789, .T. ) ;
#94132=DIRECTION ( 'NONE',  ( 0.000000000000000000, 1.000000000000000000, 2.891205793294679805E-16 ) ) ;
#94145=ORIENTED_EDGE ( 'NONE', *, *, #229525, .F. ) ;
#94176=PLANE ( 'NONE',  #1514 ) ;
#94181=VERTEX_POINT ( 'NONE', #228294 ) ;
#94186=VERTEX_POINT ( 'NONE', #70527 ) ;
#94247=DIRECTION ( 'NONE',  ( 0.000000000000000000, 0.000000000000000000, -1.000000000000000000 ) ) ;
#94271=( BOUNDED_SURFACE ( )  B_SPLINE_SURFACE ( 3, 2, ( 
 ( #101514, #98954, #16900 ),
 ( #97677, #37757, #57270 ),
 ( #58557, #39034, #121156 ),
 ( #156435, #76849, #96402 ),
 ( #136824, #177276, #237223 ),
 ( #36479, #216361, #238496 ),
 ( #198085, #181114, #78126 ),
 ( #217624, #2438, #116004 ),
 ( #118573, #81953, #258009 ),
 ( #59834, #139376, #218920 ),
 ( #40343, #20756, #100241 ),
 ( #179829, #1147, #160279 ) ),
 .UNSPECIFIED., .F., .F., .T. ) 
 B_SPLINE_SURFACE_WITH_KNOTS ( ( 4, 2, 2, 2, 2, 4 ),
 ( 3, 3 ),
 ( 3.174653483277205090, 3.943930578431714018, 4.713207673586222946, 5.482484768740731873, 5.867123316317986337, 6.251761863895240801 ),
 ( 0.000000000000000000, 1.000000000000000000 ),
 .UNSPECIFIED. ) 
 GEOMETRIC_REPRESENTATION_ITEM ( )  RATIONAL_B_SPLINE_SURFACE ( (
 ( 1.000000000000000000, 0.8659465255642357917, 1.000000000000000000),
 ( 1.000000000000000000, 0.8648614068488756912, 1.000000000000000000),
 ( 1.000000000000000000, 0.8489031841323320116, 1.000000000000000000),
 ( 1.000000000000000000, 0.7927507630162191621, 1.000000000000000000),
 ( 1.000000000000000000, 0.7523013859014273663, 1.000000000000000000),
 ( 1.000000000000000000, 0.6616226951191639394, 1.000000000000000000),
 ( 1.000000000000000000, 0.6112214368730266578, 1.000000000000000000),
 ( 1.000000000000000000, 0.5507684314495190359, 1.000000000000000000),
 ( 1.000000000000000000, 0.5333267243157234772, 1.000000000000000000),
 ( 1.000000000000000000, 0.5084565446475229900, 1.000000000000000000),
 ( 1.000000000000000000, 0.5010722703454241200, 1.000000000000000000),
 ( 1.000000000000000000, 0.5001234037138393429, 1.000000000000000000) ) ) 
 REPRESENTATION_ITEM ( '' )  SURFACE ( )  );
#94272=CARTESIAN_POINT ( 'NONE',  ( 23.24999999999999289, 11.65000000000000746, 11.75000000000000000 ) ) ;
#94310=FACE_OUTER_BOUND ( 'NONE', #167639, .T. ) ;
#94330=DIRECTION ( 'NONE',  ( 0.000000000000000000, 0.000000000000000000, -1.000000000000000000 ) ) ;
#94338=DIRECTION ( 'NONE',  ( 0.000000000000000000, 0.000000000000000000, -1.000000000000000000 ) ) ;
#94341=DIRECTION ( 'NONE',  ( -1.000000000000000000, -0.000000000000000000, -0.000000000000000000 ) ) ;
#94357=ORIENTED_EDGE ( 'NONE', *, *, #157521, .T. ) ;
#94363=EDGE_CURVE ( 'NONE', #247150, #244468, #141166, .T. ) ;
#94374=VERTEX_POINT ( 'NONE', #194322 ) ;
#94377=ADVANCED_FACE ( 'NONE', ( #33980 ), #124826, .T. ) ;
#94378=AXIS2_PLACEMENT_3D ( 'NONE', #185573, #4353, #106009 ) ;
#94395=DIRECTION ( 'NONE',  ( 0.000000000000000000, 3.552713678800500535E-15, -1.000000000000000000 ) ) ;
#94402=AXIS2_PLACEMENT_3D ( 'NONE', #55276, #174024, #38332 ) ;
#94407=ORIENTED_EDGE ( 'NONE', *, *, #147678, .F. ) ;
#94429=CARTESIAN_POINT ( 'NONE',  ( 20.85000000000000142, 0.000000000000000000, -33.50000000000000000 ) ) ;
#94445=B_SPLINE_CURVE_WITH_KNOTS ( 'NONE', 3,
 ( #252867, #153831, #74275, #36425 ),
 .UNSPECIFIED., .F., .F.,
 ( 4, 4 ),
 ( 0.000000000000000000, 0.0002118541922231894411 ),
 .UNSPECIFIED. ) ;
#94514=SPHERICAL_SURFACE ( 'NONE', #154523, 0.1000000000000000056 ) ;
#94529=ADVANCED_FACE ( 'NONE', ( #252331 ), #35890, .T. ) ;
#94531=DIRECTION ( 'NONE',  ( 0.000000000000000000, 0.000000000000000000, 1.000000000000000000 ) ) ;
#94543=CIRCLE ( 'NONE', #207571, 4.000000000000000000 ) ;
#94576=DIRECTION ( 'NONE',  ( 0.000000000000000000, 0.4999999999999863998, -0.8660254037844464792 ) ) ;
#94582=ORIENTED_EDGE ( 'NONE', *, *, #172204, .T. ) ;
#94613=ORIENTED_EDGE ( 'NONE', *, *, #128000, .F. ) ;
#94618=TOROIDAL_SURFACE ( 'NONE', #127962, 0.2000000000000000111, 0.1000000000000000056 ) ;
#94655=CARTESIAN_POINT ( 'NONE',  ( -18.50000000000000000, 9.250000000000001776, -21.25000000000000000 ) ) ;
#94704=VERTEX_POINT ( 'NONE', #41027 ) ;
#94771=CARTESIAN_POINT ( 'NONE',  ( -20.94999999999999929, 0.2561057920922211739, 0.03489644167229202787 ) ) ;
#94835=VERTEX_POINT ( 'NONE', #3137 ) ;
#94840=DIRECTION ( 'NONE',  ( -1.000000000000000000, 7.304098846218134667E-16, 4.217023435051625732E-16 ) ) ;
#94842=DIRECTION ( 'NONE',  ( 0.000000000000000000, 0.000000000000000000, -1.000000000000000000 ) ) ;
#94865=ORIENTED_EDGE ( 'NONE', *, *, #236139, .T. ) ;
#94868=VECTOR ( 'NONE', #177132, 1000.000000000000000 ) ;
#94873=CARTESIAN_POINT ( 'NONE',  ( 21.05000000000000071, -9.000000000000001776, -9.893969122652443104 ) ) ;
#94879=CARTESIAN_POINT ( 'NONE',  ( 18.60000000000000497, -9.523946312317709939, -40.38202799533822684 ) ) ;
#94894=DIRECTION ( 'NONE',  ( 1.000000000000000000, 0.000000000000000000, 0.000000000000000000 ) ) ;
#94918=EDGE_CURVE ( 'NONE', #50852, #44809, #11613, .T. ) ;
#94933=CIRCLE ( 'NONE', #161622, 4.049999999999998934 ) ;
#94943=CARTESIAN_POINT ( 'NONE',  ( -20.54999999999999716, 0.000000000000000000, -31.50000000000000000 ) ) ;
#94947=CARTESIAN_POINT ( 'NONE',  ( -21.05000000000000426, 6.270085863689140560, 0.03486800301310564315 ) ) ;
#94948=DIRECTION ( 'NONE',  ( 0.000000000000000000, -0.4999999999999929501, -0.8660254037844427044 ) ) ;
#94964=ADVANCED_FACE ( 'NONE', ( #55095 ), #248199, .T. ) ;
#94974=ORIENTED_EDGE ( 'NONE', *, *, #29329, .T. ) ;
#94989=AXIS2_PLACEMENT_3D ( 'NONE', #132703, #33642, #234348 ) ;
#95023=EDGE_CURVE ( 'NONE', #180003, #234900, #148985, .T. ) ;
#95034=AXIS2_PLACEMENT_3D ( 'NONE', #47591, #170175, #147999 ) ;
#95075=DIRECTION ( 'NONE',  ( -1.000000000000000000, 0.000000000000000000, 0.000000000000000000 ) ) ;
#95079=AXIS2_PLACEMENT_3D ( 'NONE', #8954, #134024, #108062 ) ;
#95083=CARTESIAN_POINT ( 'NONE',  ( -21.05000000000000071, 0.000000000000000000, -33.50000000000000000 ) ) ;
#95133=AXIS2_PLACEMENT_3D ( 'NONE', #97969, #257020, #177576 ) ;
#95136=DIRECTION ( 'NONE',  ( 0.000000000000000000, 0.000000000000000000, -1.000000000000000000 ) ) ;
#95149=DIRECTION ( 'NONE',  ( 1.000000000000000000, 2.952720810173289112E-16, -0.000000000000000000 ) ) ;
#95163=CARTESIAN_POINT ( 'NONE',  ( -23.25000000000000000, 6.982009704856444898, -37.19615211825629331 ) ) ;
#95195=ORIENTED_EDGE ( 'NONE', *, *, #75829, .F. ) ;
#95204=CARTESIAN_POINT ( 'NONE',  ( -21.00857864376268935, 11.59999999999999787, -6.928203230275555846 ) ) ;
#95224=CARTESIAN_POINT ( 'NONE',  ( 23.25000000000000000, 11.75000000000000711, -21.35000000000000142 ) ) ;
#95225=DIRECTION ( 'NONE',  ( 0.000000000000000000, 0.8660254037844385966, -0.5000000000000003331 ) ) ;
#95236=DIRECTION ( 'NONE',  ( -1.836970198721029934E-16, 1.000000000000000000, 0.000000000000000000 ) ) ;
#95265=AXIS2_PLACEMENT_3D ( 'NONE', #149385, #50237, #46388 ) ;
#95279=ORIENTED_EDGE ( 'NONE', *, *, #77540, .T. ) ;
#95285=CARTESIAN_POINT ( 'NONE',  ( 21.08078803292165659, 6.333012964437116921, 0.07918598715778434050 ) ) ;
#95325=ORIENTED_EDGE ( 'NONE', *, *, #3023, .F. ) ;
#95346=CIRCLE ( 'NONE', #12160, 0.09999999999999939493 ) ;
#95354=EDGE_LOOP ( 'NONE', ( #214465, #256853, #50569 ) ) ;
#95385=CARTESIAN_POINT ( 'NONE',  ( 20.94999999999999574, -1.835341550224411922, -11.55515129256297868 ) ) ;
#95403=ORIENTED_EDGE ( 'NONE', *, *, #236335, .T. ) ;
#95418=CARTESIAN_POINT ( 'NONE',  ( -23.15000000000000213, -9.600000000000001421, -23.60603087734756045 ) ) ;
#95456=DIRECTION ( 'NONE',  ( 1.000000000000000000, 1.836970198721029934E-16, 3.186635328391151676E-31 ) ) ;
#95461=FACE_OUTER_BOUND ( 'NONE', #122963, .T. ) ;
#95469=FACE_OUTER_BOUND ( 'NONE', #53255, .T. ) ;
#95479=EDGE_CURVE ( 'NONE', #148838, #84065, #16093, .T. ) ;
#95498=DIRECTION ( 'NONE',  ( -0.000000000000000000, 0.000000000000000000, 1.000000000000000000 ) ) ;
#95501=EDGE_CURVE ( 'NONE', #103887, #237621, #19560, .T. ) ;
#95517=AXIS2_PLACEMENT_3D ( 'NONE', #42, #57440, #239960 ) ;
#95521=CARTESIAN_POINT ( 'NONE',  ( -20.94999999999999929, -11.64999999999999858, -30.39999999999999503 ) ) ;
#95558=DIRECTION ( 'NONE',  ( 0.7071067811865475727, -0.7071067811865475727, 0.000000000000000000 ) ) ;
#95582=EDGE_LOOP ( 'NONE', ( #224705, #240071, #84832 ) ) ;
#95630=VERTEX_POINT ( 'NONE', #2536 ) ;
#95634=DIRECTION ( 'NONE',  ( -1.000000000000000000, 0.000000000000000000, 0.000000000000000000 ) ) ;
#95671=DIRECTION ( 'NONE',  ( 0.000000000000000000, -0.8660254037844411501, -0.4999999999999956701 ) ) ;
#95675=CARTESIAN_POINT ( 'NONE',  ( 20.94999999999999574, -1.835341550224411922, -11.55515129256297868 ) ) ;
#95708=FACE_OUTER_BOUND ( 'NONE', #197230, .T. ) ;
#95712=AXIS2_PLACEMENT_3D ( 'NONE', #204728, #207332, #206032 ) ;
#95735=DIRECTION ( 'NONE',  ( -1.000000000000000000, 0.000000000000000000, 0.000000000000000000 ) ) ;
#95757=CIRCLE ( 'NONE', #37534, 0.1000000000000028644 ) ;
#95762=CARTESIAN_POINT ( 'NONE',  ( 18.59999999999999076, 7.120270961697594103, -37.15956304183931991 ) ) ;
#95806=EDGE_CURVE ( 'NONE', #29061, #26218, #99590, .T. ) ;
#95839=CIRCLE ( 'NONE', #241607, 0.09999999999999971412 ) ;
#95875=EDGE_CURVE ( 'NONE', #163200, #56536, #24655, .T. ) ;
#95895=ORIENTED_EDGE ( 'NONE', *, *, #217400, .T. ) ;
#95904=CARTESIAN_POINT ( 'NONE',  ( 20.94999999999999929, -11.48912529307605546, -30.50000000000000000 ) ) ;
#95910=CARTESIAN_POINT ( 'NONE',  ( -18.59999999999999787, 11.64999999999999680, -7.014805770654001016 ) ) ;
#95928=DIRECTION ( 'NONE',  ( 0.000000000000000000, -1.000000000000000000, -0.000000000000000000 ) ) ;
#95941=DIRECTION ( 'NONE',  ( -1.000000000000000000, 0.000000000000000000, 0.000000000000000000 ) ) ;
#95943=DIRECTION ( 'NONE',  ( 1.000000000000000000, -0.000000000000000000, -0.000000000000000000 ) ) ;
#95949=DIRECTION ( 'NONE',  ( 0.000000000000000000, -0.9893560106964500722, 0.1455152366551550613 ) ) ;
#95966=CARTESIAN_POINT ( 'NONE',  ( -20.85000000000000142, -1.835859311443637010, -45.00443916879852679 ) ) ;
#95983=CARTESIAN_POINT ( 'NONE',  ( -20.54999999999999716, 0.000000000000000000, -33.50000000000000000 ) ) ;
#96010=ORIENTED_EDGE ( 'NONE', *, *, #216186, .F. ) ;
#96011=CARTESIAN_POINT ( 'NONE',  ( 21.30000000000002558, 4.959819536546777642E-16, 4.049999999999998934 ) ) ;
#96030=ORIENTED_EDGE ( 'NONE', *, *, #211457, .F. ) ;
#96038=DIRECTION ( 'NONE',  ( 1.000000000000000000, -0.000000000000000000, 0.000000000000000000 ) ) ;
#96042=EDGE_LOOP ( 'NONE', ( #77025, #151784, #232653, #73293 ) ) ;
#96067=CARTESIAN_POINT ( 'NONE',  ( 21.05000000000000071, 8.776282895292473185, -8.558628995140949769 ) ) ;
#96091=EDGE_CURVE ( 'NONE', #4416, #141605, #170350, .T. ) ;
#96097=ORIENTED_EDGE ( 'NONE', *, *, #220287, .F. ) ;
#96123=CIRCLE ( 'NONE', #104481, 0.1999999999999987899 ) ;
#96151=ADVANCED_FACE ( 'NONE', ( #66055 ), #103875, .T. ) ;
#96217=ORIENTED_EDGE ( 'NONE', *, *, #85001, .T. ) ;
#96225=CIRCLE ( 'NONE', #133656, 0.09999999999999939493 ) ;
#96240=CARTESIAN_POINT ( 'NONE',  ( 23.15000000000000213, -12.41227409414968363, -30.50000000000000000 ) ) ;
#96279=DIRECTION ( 'NONE',  ( 0.000000000000000000, 0.000000000000000000, 1.000000000000000000 ) ) ;
#96285=DIRECTION ( 'NONE',  ( 0.000000000000000000, 0.000000000000000000, -1.000000000000000000 ) ) ;
#96290=CARTESIAN_POINT ( 'NONE',  ( -18.50000000000000000, 9.350000000000001421, -21.15000000000000213 ) ) ;
#96308=ORIENTED_EDGE ( 'NONE', *, *, #186775, .T. ) ;
#96335=CARTESIAN_POINT ( 'NONE',  ( -21.14999999999999858, 11.65000000000000036, -0.1000000000000028644 ) ) ;
#96340=CIRCLE ( 'NONE', #246220, 0.2000000000000000944 ) ;
#96352=ORIENTED_EDGE ( 'NONE', *, *, #116565, .T. ) ;
#96359=ORIENTED_EDGE ( 'NONE', *, *, #160580, .F. ) ;
#96374=CARTESIAN_POINT ( 'NONE',  ( 18.59999999999997655, 11.75000000000000000, -33.50000000000000000 ) ) ;
#96402=CARTESIAN_POINT ( 'NONE',  ( 20.21494484322224849, 9.303170737868777351, -8.340265191770429354 ) ) ;
#96423=ADVANCED_FACE ( 'NONE', ( #89018 ), #186869, .T. ) ;
#96466=EDGE_LOOP ( 'NONE', ( #40028, #110743, #205847, #25988 ) ) ;
#96469=CARTESIAN_POINT ( 'NONE',  ( 18.59999999999999076, 11.65000000000000391, 11.75000000000000000 ) ) ;
#96486=LINE ( 'NONE', #156522, #122845 ) ;
#96487=CARTESIAN_POINT ( 'NONE',  ( 23.24999999999999289, 5.950000000000007283, -23.19429769496518645 ) ) ;
#96551=ORIENTED_EDGE ( 'NONE', *, *, #211986, .F. ) ;
#96585=ORIENTED_EDGE ( 'NONE', *, *, #154513, .T. ) ;
#96619=DIRECTION ( 'NONE',  ( -0.000000000000000000, -0.000000000000000000, -1.000000000000000000 ) ) ;
#96622=VERTEX_POINT ( 'NONE', #146025 ) ;
#96624=CARTESIAN_POINT ( 'NONE',  ( 23.14999999999999503, 11.65000000000000746, -21.35000000000000142 ) ) ;
#96626=DIRECTION ( 'NONE',  ( 1.000000000000000000, 0.000000000000000000, -0.000000000000000000 ) ) ;
#96643=ORIENTED_EDGE ( 'NONE', *, *, #194959, .F. ) ;
#96674=DIRECTION ( 'NONE',  ( 2.715809747126116508E-16, -1.000000000000000000, -1.629485848275670102E-15 ) ) ;
#96700=VERTEX_POINT ( 'NONE', #126469 ) ;
#96749=ORIENTED_EDGE ( 'NONE', *, *, #103639, .F. ) ;
#96752=DIRECTION ( 'NONE',  ( -1.000000000000000000, -0.000000000000000000, -0.000000000000000000 ) ) ;
#96803=CARTESIAN_POINT ( 'NONE',  ( -18.44448725179914206, -9.490081715483329461, -40.12896029406248033 ) ) ;
#96820=CARTESIAN_POINT ( 'NONE',  ( -23.15000000000000213, -11.48912529307605368, -30.39999999999999503 ) ) ;
#96821=TOROIDAL_SURFACE ( 'NONE', #117698, 2.100000000000002309, 0.1000000000000000056 ) ;
#96828=ORIENTED_EDGE ( 'NONE', *, *, #92904, .T. ) ;
#96830=CARTESIAN_POINT ( 'NONE',  ( 23.24999999999999645, 0.000000000000000000, 0.000000000000000000 ) ) ;
#96836=EDGE_CURVE ( 'NONE', #251327, #234302, #91201, .T. ) ;
#96870=CARTESIAN_POINT ( 'NONE',  ( -20.54999999999999716, 2.399999999999999467, -13.22462192276210224 ) ) ;
#96926=DIRECTION ( 'NONE',  ( 1.000000000000000000, -0.000000000000000000, -0.000000000000000000 ) ) ;
#96963=CARTESIAN_POINT ( 'NONE',  ( 20.94999999999999929, 6.550000000000000711, -12.15000000000000036 ) ) ;
#96979=CARTESIAN_POINT ( 'NONE',  ( 21.00000000000000000, 9.749999999999998224, -21.15000000000000213 ) ) ;
#96981=ORIENTED_EDGE ( 'NONE', *, *, #179744, .F. ) ;
#96994=CARTESIAN_POINT ( 'NONE',  ( -20.64999999999999858, 7.150000000000000355, -12.34999999999999964 ) ) ;
#97009=VECTOR ( 'NONE', #197500, 1000.000000000000000 ) ;
#97032=DIRECTION ( 'NONE',  ( 0.7070776581708965169, 0.000000000000000000, 0.7071359030027827286 ) ) ;
#97049=ADVANCED_FACE ( 'NONE', ( #222673 ), #85707, .F. ) ;
#97059=DIRECTION ( 'NONE',  ( 1.000000000000000000, 0.000000000000000000, 0.000000000000000000 ) ) ;
#97098=CARTESIAN_POINT ( 'NONE',  ( -23.25000000000000000, 0.000000000000000000, -33.50000000000000000 ) ) ;
#97122=VERTEX_POINT ( 'NONE', #75198 ) ;
#97123=EDGE_CURVE ( 'NONE', #115218, #248248, #104248, .T. ) ;
#97154=ORIENTED_EDGE ( 'NONE', *, *, #129430, .T. ) ;
#97156=DIRECTION ( 'NONE',  ( 0.000000000000000000, 1.000000000000000000, 0.000000000000000000 ) ) ;
#97161=DIRECTION ( 'NONE',  ( 1.000000000000000000, -0.000000000000000000, -0.000000000000000000 ) ) ;
#97169=LINE ( 'NONE', #132497, #247341 ) ;
#97197=CARTESIAN_POINT ( 'NONE',  ( -18.59999999999999787, -1.135018845910178431, -41.21697688343231647 ) ) ;
#97209=CIRCLE ( 'NONE', #235207, 0.09999999999999939493 ) ;
#97227=TOROIDAL_SURFACE ( 'NONE', #151477, 7.800000000000000711, 0.1000000000000000056 ) ;
#97244=ORIENTED_EDGE ( 'NONE', *, *, #251905, .T. ) ;
#97267=DIRECTION ( 'NONE',  ( 1.000000000000000000, 1.875376730785737719E-16, 0.000000000000000000 ) ) ;
#97273=DIRECTION ( 'NONE',  ( -2.342056488767301376E-15, -0.1350103645451904977, 0.9908441862701596881 ) ) ;
#97282=DIRECTION ( 'NONE',  ( -1.000000000000000000, -0.000000000000000000, -0.000000000000000000 ) ) ;
#97313=EDGE_LOOP ( 'NONE', ( #160704, #105916, #127264, #153517 ) ) ;
#97320=ORIENTED_EDGE ( 'NONE', *, *, #250917, .F. ) ;
#97338=ORIENTED_EDGE ( 'NONE', *, *, #99381, .T. ) ;
#97340=CARTESIAN_POINT ( 'NONE',  ( -21.55000000000000426, 7.708578643762696636, -21.15000000000000213 ) ) ;
#97347=VERTEX_POINT ( 'NONE', #9436 ) ;
#97348=VERTEX_POINT ( 'NONE', #250609 ) ;
#97367=CIRCLE ( 'NONE', #239053, 0.09999999999999939493 ) ;
#97373=EDGE_LOOP ( 'NONE', ( #20133, #10870, #60979, #207704 ) ) ;
#97395=CARTESIAN_POINT ( 'NONE',  ( -21.05000000000000071, -11.64999999999999858, -30.59999999999999432 ) ) ;
#97407=CARTESIAN_POINT ( 'NONE',  ( -22.50047199487840999, 0.04490605192048083977, 11.75004741891856597 ) ) ;
#97424=CARTESIAN_POINT ( 'NONE',  ( -20.54999999999999716, -9.000000000000003553, -9.893969122652444881 ) ) ;
#97438=ORIENTED_EDGE ( 'NONE', *, *, #147191, .F. ) ;
#97457=CIRCLE ( 'NONE', #243217, 0.1000000000000001721 ) ;
#97493=FACE_OUTER_BOUND ( 'NONE', #47590, .T. ) ;
#97496=ORIENTED_EDGE ( 'NONE', *, *, #172646, .T. ) ;
#97501=CARTESIAN_POINT ( 'NONE',  ( 18.49351773456751857, -9.443025695145427889, -7.185325526027306786 ) ) ;
#97544=ADVANCED_FACE ( 'NONE', ( #216623 ), #256984, .F. ) ;
#97575=DIRECTION ( 'NONE',  ( -0.000000000000000000, -1.000000000000000000, 0.000000000000000000 ) ) ;
#97590=DIRECTION ( 'NONE',  ( 0.000000000000000000, 1.000000000000000000, 2.891205793294679805E-16 ) ) ;
#97598=CIRCLE ( 'NONE', #168604, 0.09999999999999939493 ) ;
#97613=VECTOR ( 'NONE', #257636, 1000.000000000000000 ) ;
#97616=VECTOR ( 'NONE', #187192, 1000.000000000000000 ) ;
#97618=DIRECTION ( 'NONE',  ( -1.000000000000000000, 0.000000000000000000, 0.000000000000000000 ) ) ;
#97627=CARTESIAN_POINT ( 'NONE',  ( -21.37071067811865532, 8.070710678118656389, -21.15000000000000213 ) ) ;
#97645=EDGE_CURVE ( 'NONE', #210716, #227165, #55187, .T. ) ;
#97649=DIRECTION ( 'NONE',  ( 0.000000000000000000, -0.8700118002898359348, 0.4930308989875165082 ) ) ;
#97659=DIRECTION ( 'NONE',  ( -1.000000000000000000, -0.000000000000000000, 0.000000000000000000 ) ) ;
#97677=CARTESIAN_POINT ( 'NONE',  ( 20.77526135991778133, 8.932009016622666664, -8.468568542723934556 ) ) ;
#97693=CARTESIAN_POINT ( 'NONE',  ( 21.14999999999999503, 11.65000000000000746, -0.1000000000000028644 ) ) ;
#97727=EDGE_LOOP ( 'NONE', ( #161802, #86087, #206215, #138639 ) ) ;
#97744=CIRCLE ( 'NONE', #243511, 2.100000000000004530 ) ;
#97755=LINE ( 'NONE', #172236, #219453 ) ;
#97760=DIRECTION ( 'NONE',  ( -0.000000000000000000, -1.000000000000000000, -0.000000000000000000 ) ) ;
#97773=EDGE_CURVE ( 'NONE', #135192, #95630, #6561, .T. ) ;
#97777=CIRCLE ( 'NONE', #231108, 0.09999999999999939493 ) ;
#97839=CARTESIAN_POINT ( 'NONE',  ( -22.39999999999999858, 11.75000000000000000, 0.09999999999999592548 ) ) ;
#97844=ORIENTED_EDGE ( 'NONE', *, *, #67270, .F. ) ;
#97851=DIRECTION ( 'NONE',  ( -3.265361837132813586E-16, 1.000000000000000000, 0.000000000000000000 ) ) ;
#97858=EDGE_CURVE ( 'NONE', #92976, #33536, #9140, .T. ) ;
#97899=AXIS2_PLACEMENT_3D ( 'NONE', #96290, #16797, #218809 ) ;
#97901=AXIS2_PLACEMENT_3D ( 'NONE', #192906, #255379, #114642 ) ;
#97924=ADVANCED_FACE ( 'NONE', ( #55935 ), #172103, .F. ) ;
#97950=ORIENTED_EDGE ( 'NONE', *, *, #172783, .F. ) ;
#97963=CIRCLE ( 'NONE', #64664, 0.09999999999999939493 ) ;
#97969=CARTESIAN_POINT ( 'NONE',  ( 21.97500000000000497, 9.749999999999998224, -12.35000000000000320 ) ) ;
#97976=ORIENTED_EDGE ( 'NONE', *, *, #194523, .T. ) ;
#97994=B_SPLINE_CURVE_WITH_KNOTS ( 'NONE', 3,
 ( #68623, #128594, #208148, #102573, #182154, #162595, #242109, #142990 ),
 .UNSPECIFIED., .F., .F.,
 ( 4, 2, 2, 4 ),
 ( 0.000000000000000000, 0.0001881495939909221806, 0.0002822243909863843552, 0.0003762991879818465297 ),
 .UNSPECIFIED. ) ;
#98001=DIRECTION ( 'NONE',  ( -1.000000000000000000, 0.000000000000000000, 0.000000000000000000 ) ) ;
#98016=AXIS2_PLACEMENT_3D ( 'NONE', #29536, #188570, #50324 ) ;
#98017=EDGE_LOOP ( 'NONE', ( #70089, #167987, #44297, #138991 ) ) ;
#98019=ORIENTED_EDGE ( 'NONE', *, *, #57836, .F. ) ;
#98044=VECTOR ( 'NONE', #187130, 1000.000000000000000 ) ;
#98048=CARTESIAN_POINT ( 'NONE',  ( 20.94999999999999929, 0.000000000000000000, -33.50000000000000000 ) ) ;
#98052=DIRECTION ( 'NONE',  ( 0.000000000000000000, -0.000000000000000000, 1.000000000000000000 ) ) ;
#98138=TOROIDAL_SURFACE ( 'NONE', #44001, 2.100000000000002309, 0.1000000000000000056 ) ;
#98182=ADVANCED_FACE ( 'NONE', ( #45380 ), #67507, .F. ) ;
#98193=ORIENTED_EDGE ( 'NONE', *, *, #234035, .F. ) ;
#98200=AXIS2_PLACEMENT_3D ( 'NONE', #244383, #163583, #29247 ) ;
#98230=VERTEX_POINT ( 'NONE', #205730 ) ;
#98237=ORIENTED_EDGE ( 'NONE', *, *, #143252, .F. ) ;
#98247=FACE_OUTER_BOUND ( 'NONE', #139699, .T. ) ;
#98258=CIRCLE ( 'NONE', #198253, 4.299999999999956302 ) ;
#98277=DIRECTION ( 'NONE',  ( 0.000000000000000000, 0.000000000000000000, -1.000000000000000000 ) ) ;
#98289=CARTESIAN_POINT ( 'NONE',  ( 21.05000000000000071, 10.72371710470752149, -12.16119029412744545 ) ) ;
#98311=ORIENTED_EDGE ( 'NONE', *, *, #22064, .F. ) ;
#98313=AXIS2_PLACEMENT_3D ( 'NONE', #125790, #205314, #224882 ) ;
#98331=DIRECTION ( 'NONE',  ( 1.000000000000000000, 0.000000000000000000, 0.000000000000000000 ) ) ;
#98340=CARTESIAN_POINT ( 'NONE',  ( 21.14999999999999858, 6.649999999999999467, -12.25000000000000000 ) ) ;
#98344=DIRECTION ( 'NONE',  ( 0.000000000000000000, -1.000000000000000000, 0.000000000000000000 ) ) ;
#98367=EDGE_CURVE ( 'NONE', #107823, #117400, #212173, .T. ) ;
#98384=EDGE_CURVE ( 'NONE', #242875, #71337, #131664, .T. ) ;
#98438=EDGE_LOOP ( 'NONE', ( #6543, #97244, #2897, #23546 ) ) ;
#98446=ADVANCED_FACE ( 'NONE', ( #240707 ), #254476, .F. ) ;
#98448=EDGE_CURVE ( 'NONE', #131148, #187669, #229574, .T. ) ;
#98467=ORIENTED_EDGE ( 'NONE', *, *, #256157, .T. ) ;
#98469=CARTESIAN_POINT ( 'NONE',  ( 20.94999999999999929, 5.849999999999949019, -10.13249722427797117 ) ) ;
#98471=ORIENTED_EDGE ( 'NONE', *, *, #120101, .T. ) ;
#98509=CARTESIAN_POINT ( 'NONE',  ( -21.14999999999999858, -0.09999999999999939493, 11.64957080754480323 ) ) ;
#98514=CARTESIAN_POINT ( 'NONE',  ( 20.94999999999999574, -11.74999999999999112, -2.900000000000003464 ) ) ;
#98529=DIRECTION ( 'NONE',  ( 0.000000000000000000, 1.000000000000000000, 0.000000000000000000 ) ) ;
#98536=AXIS2_PLACEMENT_3D ( 'NONE', #252272, #117901, #59179 ) ;
#98539=ORIENTED_EDGE ( 'NONE', *, *, #25189, .F. ) ;
#98541=CYLINDRICAL_SURFACE ( 'NONE', #22320, 11.79999999999999716 ) ;
#98549=CIRCLE ( 'NONE', #15227, 4.049999999999998934 ) ;
#98555=AXIS2_PLACEMENT_3D ( 'NONE', #2622, #204670, #82144 ) ;
#98569=EDGE_CURVE ( 'NONE', #130475, #32767, #223687, .T. ) ;
#98603=CARTESIAN_POINT ( 'NONE',  ( -18.50000000000000000, 5.949999999999945111, -10.30570230503485796 ) ) ;
#98607=ORIENTED_EDGE ( 'NONE', *, *, #53381, .F. ) ;
#98635=CARTESIAN_POINT ( 'NONE',  ( 20.94999999999999574, 6.400000000000003020, -9.930424630061574831 ) ) ;
#98639=VECTOR ( 'NONE', #151788, 1000.000000000000000 ) ;
#98753=CARTESIAN_POINT ( 'NONE',  ( 21.14999999999999858, -1.124859753953710850E-15, 6.540656951701244282 ) ) ;
#98762=DIRECTION ( 'NONE',  ( 0.000000000000000000, 1.000000000000000000, -0.000000000000000000 ) ) ;
#98766=CARTESIAN_POINT ( 'NONE',  ( 22.49999999999999645, 0.04562336059637162045, 11.65050433855055978 ) ) ;
#98805=DIRECTION ( 'NONE',  ( 0.000000000000000000, 0.000000000000000000, -1.000000000000000000 ) ) ;
#98818=AXIS2_PLACEMENT_3D ( 'NONE', #189064, #54676, #152538 ) ;
#98881=EDGE_LOOP ( 'NONE', ( #86308, #242243, #137274, #218070 ) ) ;
#98895=CARTESIAN_POINT ( 'NONE',  ( -23.25000000000000000, -11.65000000000000036, 11.75000000000000000 ) ) ;
#98922=AXIS2_PLACEMENT_3D ( 'NONE', #123102, #240468, #86495 ) ;
#98930=LINE ( 'NONE', #162808, #234293 ) ;
#98931=CARTESIAN_POINT ( 'NONE',  ( -23.25000000000000000, 6.933893972126341509, -37.28564583437357527 ) ) ;
#98933=DIRECTION ( 'NONE',  ( -1.000000000000000000, -0.000000000000000000, 0.000000000000000000 ) ) ;
#98945=DIRECTION ( 'NONE',  ( -1.000000000000000000, -0.000000000000000000, -0.000000000000000000 ) ) ;
#98954=CARTESIAN_POINT ( 'NONE',  ( 20.97217846901852312, 8.875441724709672187, -8.501227683937228718 ) ) ;
#98989=VECTOR ( 'NONE', #191045, 1000.000000000000000 ) ;
#98992=CIRCLE ( 'NONE', #244746, 0.09999999999999939493 ) ;
#99017=DIRECTION ( 'NONE',  ( 0.000000000000000000, 0.000000000000000000, -1.000000000000000000 ) ) ;
#99042=VECTOR ( 'NONE', #105680, 1000.000000000000000 ) ;
#99055=DIRECTION ( 'NONE',  ( 0.000000000000000000, 0.000000000000000000, 1.000000000000000000 ) ) ;
#99064=CARTESIAN_POINT ( 'NONE',  ( 18.59999999999999076, 1.835341550224411922, -11.55515129256298046 ) ) ;
#99067=TOROIDAL_SURFACE ( 'NONE', #24110, 0.2000000000000000111, 0.1000000000000000056 ) ;
#99110=ADVANCED_FACE ( 'NONE', ( #217618 ), #35202, .F. ) ;
#99111=CARTESIAN_POINT ( 'NONE',  ( 21.08621493067296271, 6.349294291171669435, 0.05619483947610788566 ) ) ;
#99193=FACE_OUTER_BOUND ( 'NONE', #257201, .T. ) ;
#99229=CARTESIAN_POINT ( 'NONE',  ( -21.05000000000000071, -1.835341550224413698, -11.55515129256298046 ) ) ;
#99250=CARTESIAN_POINT ( 'NONE',  ( -20.64999999999999858, 1.940186915887848196, -20.67088078894667547 ) ) ;
#99273=LINE ( 'NONE', #217934, #145295 ) ;
#99298=AXIS2_PLACEMENT_3D ( 'NONE', #87205, #245013, #6399 ) ;
#99301=AXIS2_PLACEMENT_3D ( 'NONE', #231506, #110255, #13729 ) ;
#99308=ADVANCED_FACE ( 'NONE', ( #6283 ), #126236, .T. ) ;
#99309=AXIS2_PLACEMENT_3D ( 'NONE', #242896, #25163, #108524 ) ;
#99322=ORIENTED_EDGE ( 'NONE', *, *, #200462, .T. ) ;
#99327=DIRECTION ( 'NONE',  ( 0.000000000000000000, -1.000000000000000000, 0.000000000000000000 ) ) ;
#99333=CARTESIAN_POINT ( 'NONE',  ( -20.54999999999999716, -9.500000000000001776, -23.60603087734756045 ) ) ;
#99350=DIRECTION ( 'NONE',  ( 1.836970198721029934E-16, -1.000000000000000000, -0.000000000000000000 ) ) ;
#99351=LINE ( 'NONE', #215465, #182737 ) ;
#99380=ORIENTED_EDGE ( 'NONE', *, *, #223064, .T. ) ;
#99381=EDGE_CURVE ( 'NONE', #186188, #157226, #246497, .T. ) ;
#99459=DIRECTION ( 'NONE',  ( -1.000000000000000000, -0.000000000000000000, -0.000000000000000000 ) ) ;
#99462=ORIENTED_EDGE ( 'NONE', *, *, #113638, .F. ) ;
#99467=DIRECTION ( 'NONE',  ( -1.000000000000000000, 0.000000000000000000, 0.000000000000000000 ) ) ;
#99504=LINE ( 'NONE', #79929, #202203 ) ;
#99508=DIRECTION ( 'NONE',  ( 0.000000000000000000, 0.000000000000000000, 1.000000000000000000 ) ) ;
#99511=CARTESIAN_POINT ( 'NONE',  ( -23.25000000000000000, 0.000000000000000000, 0.000000000000000000 ) ) ;
#99541=CARTESIAN_POINT ( 'NONE',  ( -23.15000000000000213, 0.000000000000000000, 0.000000000000000000 ) ) ;
#99564=DIRECTION ( 'NONE',  ( 1.000000000000000000, 0.000000000000000000, 0.000000000000000000 ) ) ;
#99573=DIRECTION ( 'NONE',  ( 0.000000000000000000, -0.1350103645451904977, -0.9908441862701596881 ) ) ;
#99590=CIRCLE ( 'NONE', #124579, 11.70000000000000284 ) ;
#99614=CARTESIAN_POINT ( 'NONE',  ( -21.00023020733502932, -5.827586677109586333E-16, 6.390869245268355314 ) ) ;
#99676=DIRECTION ( 'NONE',  ( 1.000000000000000000, 0.000000000000000000, 0.000000000000000000 ) ) ;
#99688=ORIENTED_EDGE ( 'NONE', *, *, #194198, .F. ) ;
#99700=ORIENTED_EDGE ( 'NONE', *, *, #202221, .T. ) ;
#99721=ADVANCED_FACE ( 'NONE', ( #9839 ), #65964, .T. ) ;
#99726=ORIENTED_EDGE ( 'NONE', *, *, #10498, .T. ) ;
#99734=ORIENTED_EDGE ( 'NONE', *, *, #161146, .F. ) ;
#99748=CARTESIAN_POINT ( 'NONE',  ( 20.04142135623731136, 11.75000000000000711, -24.76715728752538226 ) ) ;
#99754=DIRECTION ( 'NONE',  ( 0.000000000000000000, 0.4999999999999966693, -0.8660254037844405950 ) ) ;
#99784=VERTEX_POINT ( 'NONE', #247153 ) ;
#99798=DIRECTION ( 'NONE',  ( 1.000000000000000000, 0.000000000000000000, 0.000000000000000000 ) ) ;
#99800=DIRECTION ( 'NONE',  ( 1.000000000000000000, 0.000000000000000000, -1.734723475976817507E-14 ) ) ;
#99823=ADVANCED_FACE ( 'NONE', ( #225012 ), #46380, .F. ) ;
#99835=ORIENTED_EDGE ( 'NONE', *, *, #116517, .T. ) ;
#99859=CARTESIAN_POINT ( 'NONE',  ( -23.25000000000000000, 0.000000000000000000, 0.000000000000000000 ) ) ;
#99861=DIRECTION ( 'NONE',  ( 0.000000000000000000, 0.000000000000000000, -1.000000000000000000 ) ) ;
#99907=ORIENTED_EDGE ( 'NONE', *, *, #5406, .F. ) ;
#99955=ORIENTED_EDGE ( 'NONE', *, *, #183333, .F. ) ;
#100010=EDGE_CURVE ( 'NONE', #143109, #19453, #250395, .T. ) ;
#100035=DIRECTION ( 'NONE',  ( 0.000000000000000000, 0.000000000000000000, -1.000000000000000000 ) ) ;
#100047=CARTESIAN_POINT ( 'NONE',  ( 21.11825140030076753, 0.007203620632672789147, 6.445407565420044449 ) ) ;
#100062=DIRECTION ( 'NONE',  ( 3.616040088954497272E-32, -1.224646799147352961E-16, 1.000000000000000000 ) ) ;
#100110=AXIS2_PLACEMENT_3D ( 'NONE', #186727, #5473, #122897 ) ;
#100113=VECTOR ( 'NONE', #33959, 1000.000000000000000 ) ;
#100133=ORIENTED_EDGE ( 'NONE', *, *, #38106, .F. ) ;
#100141=DIRECTION ( 'NONE',  ( -1.836970198721029934E-16, 1.000000000000000000, 0.000000000000000000 ) ) ;
#100159=DIRECTION ( 'NONE',  ( -1.000000000000000000, -0.000000000000000000, 0.000000000000000000 ) ) ;
#100187=DIRECTION ( 'NONE',  ( 0.000000000000000000, 0.000000000000000000, -1.000000000000000000 ) ) ;
#100188=ADVANCED_FACE ( 'NONE', ( #143900 ), #246849, .T. ) ;
#100204=CIRCLE ( 'NONE', #108435, 0.09999999999999832634 ) ;
#100227=FACE_OUTER_BOUND ( 'NONE', #229831, .T. ) ;
#100240=EDGE_CURVE ( 'NONE', #116906, #67614, #5650, .T. ) ;
#100241=CARTESIAN_POINT ( 'NONE',  ( 20.86036036209909383, 10.62104277657096318, -7.666348418505070761 ) ) ;
#100245=ORIENTED_EDGE ( 'NONE', *, *, #234238, .T. ) ;
#100250=AXIS2_PLACEMENT_3D ( 'NONE', #163833, #187258, #105093 ) ;
#100272=CARTESIAN_POINT ( 'NONE',  ( 18.59999999999999076, 0.000000000000000000, -33.50000000000000000 ) ) ;
#100274=FACE_OUTER_BOUND ( 'NONE', #46810, .T. ) ;
#100290=DIRECTION ( 'NONE',  ( 0.000000000000000000, 0.000000000000000000, 1.000000000000000000 ) ) ;
#100296=CIRCLE ( 'NONE', #146109, 0.09999999999999939493 ) ;
#100308=CARTESIAN_POINT ( 'NONE',  ( 21.05000000000000071, 0.000000000000000000, -33.50000000000000000 ) ) ;
#100314=AXIS2_PLACEMENT_3D ( 'NONE', #96335, #118510, #81890 ) ;
#100315=CARTESIAN_POINT ( 'NONE',  ( 23.24999999999997513, 11.75000000000000711, -26.48519422934605672 ) ) ;
#100365=CARTESIAN_POINT ( 'NONE',  ( -21.29999999999995808, 4.959819536546777642E-16, 4.049999999999998934 ) ) ;
#100371=PLANE ( 'NONE',  #236386 ) ;
#100408=ADVANCED_FACE ( 'NONE', ( #176061 ), #212604, .T. ) ;
#100422=ORIENTED_EDGE ( 'NONE', *, *, #6203, .T. ) ;
#100425=DIRECTION ( 'NONE',  ( 0.000000000000000000, -1.000000000000000000, 0.000000000000000000 ) ) ;
#100426=ORIENTED_EDGE ( 'NONE', *, *, #210634, .F. ) ;
#100437=DIRECTION ( 'NONE',  ( -6.938893903907222856E-15, 1.000000000000000000, 0.000000000000000000 ) ) ;
#100438=AXIS2_PLACEMENT_3D ( 'NONE', #134601, #35557, #12142 ) ;
#100458=ORIENTED_EDGE ( 'NONE', *, *, #85258, .T. ) ;
#100466=DIRECTION ( 'NONE',  ( 0.000000000000000000, 0.000000000000000000, -1.000000000000000000 ) ) ;
#100482=CARTESIAN_POINT ( 'NONE',  ( -20.85000000000000142, -11.65000000000000036, -30.59999999999999432 ) ) ;
#100572=CIRCLE ( 'NONE', #192201, 0.1000000000000028644 ) ;
#100601=CIRCLE ( 'NONE', #29940, 0.09999999999999939493 ) ;
#100625=CARTESIAN_POINT ( 'NONE',  ( 20.97224591636398827, 10.62515341616362363, -12.24992590466357534 ) ) ;
#100627=CARTESIAN_POINT ( 'NONE',  ( -18.54270223418606633, -9.624105502882903451, -40.24093505040743679 ) ) ;
#100675=DIRECTION ( 'NONE',  ( 1.000000000000000000, 0.000000000000000000, 0.000000000000000000 ) ) ;
#100713=ORIENTED_EDGE ( 'NONE', *, *, #189155, .T. ) ;
#100747=ADVANCED_FACE ( 'NONE', ( #157140 ), #16347, .T. ) ;
#100749=ORIENTED_EDGE ( 'NONE', *, *, #56439, .T. ) ;
#100763=ORIENTED_EDGE ( 'NONE', *, *, #49642, .T. ) ;
#100785=AXIS2_PLACEMENT_3D ( 'NONE', #100308, #221534, #99017 ) ;
#100791=DIRECTION ( 'NONE',  ( -0.000000000000000000, -0.000000000000000000, 1.000000000000000000 ) ) ;
#100836=AXIS2_PLACEMENT_3D ( 'NONE', #86817, #165094, #46414 ) ;
#100845=EDGE_LOOP ( 'NONE', ( #51361, #14307, #90238 ) ) ;
#100857=CARTESIAN_POINT ( 'NONE',  ( -18.53317502108577131, 10.32263460346243811, -39.06059579686719729 ) ) ;
#100858=DIRECTION ( 'NONE',  ( 0.000000000000000000, 0.000000000000000000, -1.000000000000000000 ) ) ;
#100861=EDGE_CURVE ( 'NONE', #156221, #138899, #225790, .T. ) ;
#100868=CARTESIAN_POINT ( 'NONE',  ( -20.96077737575330957, 11.62390063400468776, -26.64079195710655412 ) ) ;
#100876=VECTOR ( 'NONE', #57001, 1000.000000000000000 ) ;
#100888=DIRECTION ( 'NONE',  ( 0.000000000000000000, 0.000000000000000000, 1.000000000000000000 ) ) ;
#100957=AXIS2_PLACEMENT_3D ( 'NONE', #8632, #206824, #28224 ) ;
#101015=ORIENTED_EDGE ( 'NONE', *, *, #140603, .T. ) ;
#101032=DIRECTION ( 'NONE',  ( 0.000000000000000000, 1.000000000000000000, 0.000000000000000000 ) ) ;
#101044=EDGE_CURVE ( 'NONE', #160000, #50839, #229935, .T. ) ;
#101047=ORIENTED_EDGE ( 'NONE', *, *, #183769, .F. ) ;
#101069=LINE ( 'NONE', #45005, #256712 ) ;
#101085=DIRECTION ( 'NONE',  ( 0.000000000000000000, 0.000000000000000000, -1.000000000000000000 ) ) ;
#101091=VECTOR ( 'NONE', #211039, 1000.000000000000000 ) ;
#101170=VERTEX_POINT ( 'NONE', #216781 ) ;
#101174=FACE_OUTER_BOUND ( 'NONE', #158375, .T. ) ;
#101175=EDGE_LOOP ( 'NONE', ( #243499, #34829, #213936, #230347 ) ) ;
#101181=CARTESIAN_POINT ( 'NONE',  ( 20.94999999999999929, 4.999999999999997335, -21.09473398108690390 ) ) ;
#101216=ORIENTED_EDGE ( 'NONE', *, *, #221183, .F. ) ;
#101221=ORIENTED_EDGE ( 'NONE', *, *, #17947, .T. ) ;
#101229=EDGE_CURVE ( 'NONE', #101170, #94186, #61572, .T. ) ;
#101239=CARTESIAN_POINT ( 'NONE',  ( -20.64999999999999858, -9.000000000000001776, -23.60603087734756045 ) ) ;
#101242=AXIS2_PLACEMENT_3D ( 'NONE', #51257, #175144, #112563 ) ;
#101291=TOROIDAL_SURFACE ( 'NONE', #117905, 0.4000000000000009104, 0.1000000000000000056 ) ;
#101292=ORIENTED_EDGE ( 'NONE', *, *, #195968, .F. ) ;
#101313=DIRECTION ( 'NONE',  ( -0.000000000000000000, -1.000000000000000000, 0.000000000000000000 ) ) ;
#101351=CARTESIAN_POINT ( 'NONE',  ( -20.94999999999999929, 1.162701749938009677, -8.099999999999999645 ) ) ;
#101376=DIRECTION ( 'NONE',  ( 0.000000000000000000, 0.000000000000000000, -1.000000000000000000 ) ) ;
#101390=EDGE_CURVE ( 'NONE', #168114, #233652, #150113, .T. ) ;
#101398=DIRECTION ( 'NONE',  ( -1.000000000000000000, 0.000000000000000000, 0.000000000000000000 ) ) ;
#101486=ORIENTED_EDGE ( 'NONE', *, *, #177704, .F. ) ;
#101500=EDGE_CURVE ( 'NONE', #212474, #68538, #38934, .T. ) ;
#101510=CIRCLE ( 'NONE', #205780, 0.1000000000000002970 ) ;
#101514=CARTESIAN_POINT ( 'NONE',  ( 20.97438252431638972, 8.925423506075993885, -8.472370689010807254 ) ) ;
#101585=CARTESIAN_POINT ( 'NONE',  ( 22.50000000000000000, 0.000000000000000000, 0.000000000000000000 ) ) ;
#101587=DIRECTION ( 'NONE',  ( -1.000000000000000000, 9.012599976028471648E-15, 6.882867235861662930E-14 ) ) ;
#101616=ADVANCED_FACE ( 'NONE', ( #174838 ), #147053, .T. ) ;
#101618=ORIENTED_EDGE ( 'NONE', *, *, #130095, .F. ) ;
#101702=CARTESIAN_POINT ( 'NONE',  ( -22.50000000000000000, 11.64957080754479968, 0.09999999999999592548 ) ) ;
#101723=CARTESIAN_POINT ( 'NONE',  ( -23.15000000000000213, -11.65000000000000036, 11.75000000000000000 ) ) ;
#101735=VERTEX_POINT ( 'NONE', #83355 ) ;
#101738=ORIENTED_EDGE ( 'NONE', *, *, #231985, .T. ) ;
#101742=ORIENTED_EDGE ( 'NONE', *, *, #123184, .F. ) ;
#101745=ORIENTED_EDGE ( 'NONE', *, *, #34380, .T. ) ;
#101784=ORIENTED_EDGE ( 'NONE', *, *, #257293, .T. ) ;
#101791=B_SPLINE_CURVE_WITH_KNOTS ( 'NONE', 3,
 ( #80286, #233005, #54326, #133874 ),
 .UNSPECIFIED., .F., .F.,
 ( 4, 4 ),
 ( 0.000000000000000000, 0.0001048066582182440823 ),
 .UNSPECIFIED. ) ;
#101817=CARTESIAN_POINT ( 'NONE',  ( 21.14999999999999858, 6.550000000000000711, -12.35000000000000320 ) ) ;
#101825=ORIENTED_EDGE ( 'NONE', *, *, #240373, .F. ) ;
#101842=CARTESIAN_POINT ( 'NONE',  ( 18.59999999999999787, -1.736705739467587772, -45.01742258762372728 ) ) ;
#101882=CARTESIAN_POINT ( 'NONE',  ( -21.14999999999999858, -11.65000000000000036, 0.000000000000000000 ) ) ;
#101902=ORIENTED_EDGE ( 'NONE', *, *, #160197, .T. ) ;
#101955=CYLINDRICAL_SURFACE ( 'NONE', #228414, 0.09999999999999939493 ) ;
#101992=DIRECTION ( 'NONE',  ( 1.000000000000000000, 2.952720810173289112E-16, -0.000000000000000000 ) ) ;
#102041=EDGE_LOOP ( 'NONE', ( #10315, #61133, #19355, #83057 ) ) ;
#102062=ORIENTED_EDGE ( 'NONE', *, *, #128000, .T. ) ;
#102065=AXIS2_PLACEMENT_3D ( 'NONE', #192826, #254057, #178415 ) ;
#102106=EDGE_LOOP ( 'NONE', ( #99726, #61607, #39250, #159536 ) ) ;
#102116=PLANE ( 'NONE',  #140388 ) ;
#102126=DIRECTION ( 'NONE',  ( 0.000000000000000000, 0.000000000000000000, -1.000000000000000000 ) ) ;
#102129=( NAMED_UNIT ( * ) PLANE_ANGLE_UNIT ( ) SI_UNIT ( $, .RADIAN. ) );
#102134=VERTEX_POINT ( 'NONE', #80463 ) ;
#102159=AXIS2_PLACEMENT_3D ( 'NONE', #7416, #187366, #11285 ) ;
#102161=TOROIDAL_SURFACE ( 'NONE', #168879, 0.6000000000000009770, 0.1000000000000000056 ) ;
#102165=ORIENTED_EDGE ( 'NONE', *, *, #199289, .F. ) ;
#102168=ORIENTED_EDGE ( 'NONE', *, *, #202366, .F. ) ;
#102180=LINE ( 'NONE', #82617, #81792 ) ;
#102190=CIRCLE ( 'NONE', #202187, 1.900000000000005906 ) ;
#102206=ORIENTED_EDGE ( 'NONE', *, *, #220050, .F. ) ;
#102271=ORIENTED_EDGE ( 'NONE', *, *, #113325, .T. ) ;
#102295=CIRCLE ( 'NONE', #214763, 11.65000000000000036 ) ;
#102307=CARTESIAN_POINT ( 'NONE',  ( 23.14999999999999503, 11.75000000000000711, -26.48519422934605672 ) ) ;
#102320=AXIS2_PLACEMENT_3D ( 'NONE', #233139, #212279, #132742 ) ;
#102353=ORIENTED_EDGE ( 'NONE', *, *, #207502, .T. ) ;
#102394=EDGE_LOOP ( 'NONE', ( #173976, #182385, #148936, #99955 ) ) ;
#102408=CARTESIAN_POINT ( 'NONE',  ( -22.47071067811865319, 0.000000000000000000, 0.000000000000000000 ) ) ;
#102455=EDGE_LOOP ( 'NONE', ( #18174, #241197, #109147 ) ) ;
#102475=EDGE_CURVE ( 'NONE', #163200, #15934, #85219, .T. ) ;
#102488=CARTESIAN_POINT ( 'NONE',  ( 20.94999999999999929, 0.000000000000000000, -33.50000000000000000 ) ) ;
#102531=DIRECTION ( 'NONE',  ( -1.000000000000000000, 0.000000000000000000, 0.000000000000000000 ) ) ;
#102570=EDGE_CURVE ( 'NONE', #210699, #96622, #218504, .T. ) ;
#102573=CARTESIAN_POINT ( 'NONE',  ( 21.05000000000000426, -0.03753606328566945483, 6.332272273935667606 ) ) ;
#102576=FACE_OUTER_BOUND ( 'NONE', #173821, .T. ) ;
#102579=CARTESIAN_POINT ( 'NONE',  ( -20.64999999999999858, 1.999999999999998224, -20.77537807723789953 ) ) ;
#102582=CYLINDRICAL_SURFACE ( 'NONE', #175544, 0.09999999999999939493 ) ;
#102588=CARTESIAN_POINT ( 'NONE',  ( 20.85000000000000142, 6.982009704856448451, -37.19615211825629331 ) ) ;
#102592=ORIENTED_EDGE ( 'NONE', *, *, #123253, .T. ) ;
#102603=AXIS2_PLACEMENT_3D ( 'NONE', #182389, #198081, #121152 ) ;
#102628=DIRECTION ( 'NONE',  ( 0.000000000000000000, -1.000000000000000000, -1.224646799147353207E-16 ) ) ;
#102739=AXIS2_PLACEMENT_3D ( 'NONE', #203556, #83571, #200991 ) ;
#102744=ORIENTED_EDGE ( 'NONE', *, *, #130796, .F. ) ;
#102745=CARTESIAN_POINT ( 'NONE',  ( -21.00023020733437917, 6.390869245267705168, -6.911788849595090767E-16 ) ) ;
#102753=CIRCLE ( 'NONE', #23715, 11.65000000000000036 ) ;
#102759=ORIENTED_EDGE ( 'NONE', *, *, #13153, .F. ) ;
#102795=DIRECTION ( 'NONE',  ( 0.000000000000000000, 2.891205793294679805E-16, -1.000000000000000000 ) ) ;
#102801=VECTOR ( 'NONE', #218859, 1000.000000000000000 ) ;
#102818=EDGE_LOOP ( 'NONE', ( #142139, #113663, #10241, #61586 ) ) ;
#102825=CARTESIAN_POINT ( 'NONE',  ( 21.05000000000000426, 6.413826288812974674, -0.08574093703339950856 ) ) ;
#102828=CIRCLE ( 'NONE', #249175, 11.79999999999999716 ) ;
#102859=FACE_OUTER_BOUND ( 'NONE', #83509, .T. ) ;
#102862=CARTESIAN_POINT ( 'NONE',  ( -18.50000000000000000, 11.64999999999999680, 11.75000000000000000 ) ) ;
#102883=DIRECTION ( 'NONE',  ( 6.938893903907030216E-14, 0.000000000000000000, 1.000000000000000000 ) ) ;
#102931=AXIS2_PLACEMENT_3D ( 'NONE', #220553, #143582, #41936 ) ;
#102986=CIRCLE ( 'NONE', #207063, 0.09999999999999939493 ) ;
#102995=CARTESIAN_POINT ( 'NONE',  ( 23.14999999999999858, 0.000000000000000000, -33.50000000000000000 ) ) ;
#103039=ORIENTED_EDGE ( 'NONE', *, *, #238285, .T. ) ;
#103040=DIRECTION ( 'NONE',  ( -0.000000000000000000, 0.000000000000000000, 1.000000000000000000 ) ) ;
#103054=ORIENTED_EDGE ( 'NONE', *, *, #185399, .T. ) ;
#103069=VERTEX_POINT ( 'NONE', #207246 ) ;
#103075=CARTESIAN_POINT ( 'NONE',  ( -20.64999999999999858, 2.499999999999998668, -20.27537807723789953 ) ) ;
#103098=AXIS2_PLACEMENT_3D ( 'NONE', #222450, #243317, #28166 ) ;
#103102=EDGE_LOOP ( 'NONE', ( #190684, #187431, #160937, #10399 ) ) ;
#103116=VECTOR ( 'NONE', #12340, 1000.000000000000000 ) ;
#103121=EDGE_LOOP ( 'NONE', ( #170371, #64284, #117666, #235225 ) ) ;
#103178=CARTESIAN_POINT ( 'NONE',  ( -20.99142135623731065, 11.59999999999999787, -26.57179676972450011 ) ) ;
#103217=EDGE_LOOP ( 'NONE', ( #118291, #166760, #157958 ) ) ;
#103226=CARTESIAN_POINT ( 'NONE',  ( 18.59999999999999432, -1.299733671230788756, 9.971870477130599042 ) ) ;
#103246=CARTESIAN_POINT ( 'NONE',  ( -20.94999999999999929, 0.000000000000000000, -33.50000000000000000 ) ) ;
#103255=ORIENTED_EDGE ( 'NONE', *, *, #218792, .T. ) ;
#103260=CARTESIAN_POINT ( 'NONE',  ( 18.54116936837188234, -9.463564198372441894, -7.048542490888269896 ) ) ;
#103264=EDGE_LOOP ( 'NONE', ( #220225, #82227, #133284, #45020 ) ) ;
#103268=DIRECTION ( 'NONE',  ( -3.265361837132813093E-16, 1.000000000000000000, -0.000000000000000000 ) ) ;
#103273=DIRECTION ( 'NONE',  ( 2.840903330521633255E-16, -0.8700118002898322711, 0.4930308989875231696 ) ) ;
#103279=ADVANCED_FACE ( 'NONE', ( #144338 ), #223889, .T. ) ;
#103307=ORIENTED_EDGE ( 'NONE', *, *, #23538, .T. ) ;
#103328=DIRECTION ( 'NONE',  ( -0.000000000000000000, -0.000000000000000000, 1.000000000000000000 ) ) ;
#103345=AXIS2_PLACEMENT_3D ( 'NONE', #3040, #123020, #85125 ) ;
#103351=EDGE_LOOP ( 'NONE', ( #122051, #59219, #109344, #97976 ) ) ;
#103374=ORIENTED_EDGE ( 'NONE', *, *, #147678, .T. ) ;
#103399=DIRECTION ( 'NONE',  ( 1.000000000000000000, 0.000000000000000000, 0.000000000000000000 ) ) ;
#103425=EDGE_CURVE ( 'NONE', #138366, #71227, #198048, .T. ) ;
#103432=DIRECTION ( 'NONE',  ( 0.000000000000000000, 1.000000000000000000, 0.000000000000000000 ) ) ;
#103433=EDGE_CURVE ( 'NONE', #68319, #195886, #227272, .T. ) ;
#103434=DIRECTION ( 'NONE',  ( 0.000000000000000000, -1.265107689135680095E-16, 1.000000000000000000 ) ) ;
#103438=AXIS2_PLACEMENT_3D ( 'NONE', #130046, #132639, #36114 ) ;
#103443=DIRECTION ( 'NONE',  ( 1.000000000000000000, -0.000000000000000000, -0.000000000000000000 ) ) ;
#103450=LINE ( 'NONE', #186886, #45468 ) ;
#103487=ADVANCED_FACE ( 'NONE', ( #230321 ), #229057, .T. ) ;
#103581=ADVANCED_FACE ( 'NONE', ( #171676 ), #172965, .T. ) ;
#103609=EDGE_LOOP ( 'NONE', ( #23280, #117182, #233145, #165460 ) ) ;
#103612=DIRECTION ( 'NONE',  ( -1.000000000000000000, -0.000000000000000000, -0.000000000000000000 ) ) ;
#103639=EDGE_CURVE ( 'NONE', #197037, #243103, #123223, .T. ) ;
#103643=CARTESIAN_POINT ( 'NONE',  ( 21.14999999999999858, 11.75000000000000711, 11.75000000000000000 ) ) ;
#103657=EDGE_LOOP ( 'NONE', ( #207821, #213327, #176738, #148942 ) ) ;
#103662=CARTESIAN_POINT ( 'NONE',  ( 23.15000000000000213, -11.48912529307605546, -30.39999999999999503 ) ) ;
#103673=VERTEX_POINT ( 'NONE', #42399 ) ;
#103676=ORIENTED_EDGE ( 'NONE', *, *, #32369, .T. ) ;
#103685=ORIENTED_EDGE ( 'NONE', *, *, #244603, .F. ) ;
#103713=ORIENTED_EDGE ( 'NONE', *, *, #89613, .F. ) ;
#103718=EDGE_LOOP ( 'NONE', ( #192295, #6534, #57146 ) ) ;
#103735=VERTEX_POINT ( 'NONE', #183203 ) ;
#103750=CIRCLE ( 'NONE', #91333, 11.65000000000000036 ) ;
#103759=EDGE_LOOP ( 'NONE', ( #72422, #37889, #53658 ) ) ;
#103771=ORIENTED_EDGE ( 'NONE', *, *, #65192, .F. ) ;
#103788=CARTESIAN_POINT ( 'NONE',  ( 21.05000000000000071, 5.850000000000001421, -23.36750277572207679 ) ) ;
#103811=CARTESIAN_POINT ( 'NONE',  ( -23.25000000000000000, 11.75000000000000000, -26.48519422934605672 ) ) ;
#103827=EDGE_LOOP ( 'NONE', ( #52396, #151899, #52680, #20485, #98237 ) ) ;
#103838=DIRECTION ( 'NONE',  ( 1.000000000000000000, 0.000000000000000000, 0.000000000000000000 ) ) ;
#103848=VECTOR ( 'NONE', #209608, 1000.000000000000000 ) ;
#103862=EDGE_LOOP ( 'NONE', ( #235284, #150093, #72736, #240669 ) ) ;
#103863=CYLINDRICAL_SURFACE ( 'NONE', #168391, 0.09999999999999999167 ) ;
#103875=TOROIDAL_SURFACE ( 'NONE', #212260, 0.6000000000000013101, 0.1000000000000000056 ) ;
#103877=CARTESIAN_POINT ( 'NONE',  ( 18.45139536634708577, -9.486081720281200447, -40.14051161781065957 ) ) ;
#103883=DIRECTION ( 'NONE',  ( 0.000000000000000000, 0.000000000000000000, -1.000000000000000000 ) ) ;
#103887=VERTEX_POINT ( 'NONE', #254673 ) ;
#103904=DIRECTION ( 'NONE',  ( -0.000000000000000000, -0.000000000000000000, -1.000000000000000000 ) ) ;
#103908=CARTESIAN_POINT ( 'NONE',  ( -21.55000000000000071, 7.150000000000000355, -21.25000000000000000 ) ) ;
#103918=ORIENTED_EDGE ( 'NONE', *, *, #235089, .T. ) ;
#103970=DIRECTION ( 'NONE',  ( -1.000000000000000000, -0.000000000000000000, -0.000000000000000000 ) ) ;
#103987=CARTESIAN_POINT ( 'NONE',  ( 21.14999999999999503, -0.09999999999999939493, 11.64957080754479968 ) ) ;
#104005=LINE ( 'NONE', #124892, #188717 ) ;
#104023=AXIS2_PLACEMENT_3D ( 'NONE', #63525, #127367, #106484 ) ;
#104074=ORIENTED_EDGE ( 'NONE', *, *, #174940, .F. ) ;
#104093=CARTESIAN_POINT ( 'NONE',  ( 23.25000000000000000, -11.74999999999999112, 11.75000000000000000 ) ) ;
#104095=CARTESIAN_POINT ( 'NONE',  ( -18.59999999999999787, 5.899999999999947065, -10.21909976465641456 ) ) ;
#104098=CARTESIAN_POINT ( 'NONE',  ( -20.54999999999999716, -9.400000000000002132, -23.60603087734756045 ) ) ;
#104108=CARTESIAN_POINT ( 'NONE',  ( 21.05000000000000426, 6.258817194681471463, 0.03363273533363692058 ) ) ;
#104138=EDGE_CURVE ( 'NONE', #157985, #47066, #205672, .T. ) ;
#104151=ADVANCED_FACE ( 'NONE', ( #229108 ), #13917, .T. ) ;
#104171=EDGE_CURVE ( 'NONE', #178016, #219323, #171732, .T. ) ;
#104193=FACE_OUTER_BOUND ( 'NONE', #114874, .T. ) ;
#104229=DIRECTION ( 'NONE',  ( -1.000000000000000000, 0.000000000000000000, 0.000000000000000000 ) ) ;
#104239=DIRECTION ( 'NONE',  ( 0.000000000000000000, 0.000000000000000000, 1.000000000000000000 ) ) ;
#104248=CIRCLE ( 'NONE', #16804, 0.1000000000000000472 ) ;
#104261=CARTESIAN_POINT ( 'NONE',  ( 19.97071067811865674, 11.72071067811866385, -24.65000000000000213 ) ) ;
#104325=ORIENTED_EDGE ( 'NONE', *, *, #51178, .T. ) ;
#104337=DIRECTION ( 'NONE',  ( 0.000000000000000000, -0.1350103645451876666, -0.9908441862701600211 ) ) ;
#104342=EDGE_LOOP ( 'NONE', ( #148329, #192300, #78887, #174442 ) ) ;
#104350=ORIENTED_EDGE ( 'NONE', *, *, #48822, .F. ) ;
#104365=EDGE_LOOP ( 'NONE', ( #23682, #216641, #104074, #179205 ) ) ;
#104382=CARTESIAN_POINT ( 'NONE',  ( 18.59999999999999432, 1.261786168565025568, -8.086498963545480478 ) ) ;
#104403=CARTESIAN_POINT ( 'NONE',  ( 21.51976009735019346, 6.910458441659201867, 1.166362318020008541E-16 ) ) ;
#104408=CIRCLE ( 'NONE', #100314, 0.09999999999999939493 ) ;
#104412=DIRECTION ( 'NONE',  ( -1.000000000000000000, 0.000000000000000000, 0.000000000000000000 ) ) ;
#104421=SPHERICAL_SURFACE ( 'NONE', #77866, 0.1000000000000000056 ) ;
#104424=ORIENTED_EDGE ( 'NONE', *, *, #3741, .F. ) ;
#104436=VECTOR ( 'NONE', #158275, 1000.000000000000114 ) ;
#104446=EDGE_CURVE ( 'NONE', #177256, #254325, #63292, .T. ) ;
#104459=VERTEX_POINT ( 'NONE', #5878 ) ;
#104468=DIRECTION ( 'NONE',  ( 5.603264701231745086E-32, -1.897661533703520636E-16, 1.000000000000000000 ) ) ;
#104479=CIRCLE ( 'NONE', #241872, 2.100000000000002309 ) ;
#104481=AXIS2_PLACEMENT_3D ( 'NONE', #11803, #252938, #172182 ) ;
#104493=AXIS2_PLACEMENT_3D ( 'NONE', #167401, #124405, #24031 ) ;
#104506=TOROIDAL_SURFACE ( 'NONE', #250276, 0.6000000000000004219, 0.1000000000000000056 ) ;
#104521=AXIS2_PLACEMENT_3D ( 'NONE', #171276, #151695, #30445 ) ;
#104545=CARTESIAN_POINT ( 'NONE',  ( -20.87600722750343252, 10.33112638555853913, -39.09012289269746532 ) ) ;
#104549=MANIFOLD_SOLID_BREP ( 'Stock-MAS-200-1', #70045 ) ;
#104562=EDGE_CURVE ( 'NONE', #138911, #251327, #143850, .T. ) ;
#104564=ADVANCED_FACE ( 'NONE', ( #69743 ), #149287, .T. ) ;
#104586=CARTESIAN_POINT ( 'NONE',  ( -18.59999999999999787, 1.835341550224411922, -11.65515129256298010 ) ) ;
#104590=ORIENTED_EDGE ( 'NONE', *, *, #45917, .F. ) ;
#104592=CARTESIAN_POINT ( 'NONE',  ( 23.14999999999999503, 11.65000000000000746, -21.35000000000000142 ) ) ;
#104613=DIRECTION ( 'NONE',  ( -1.000000000000000000, 0.000000000000000000, 0.000000000000000000 ) ) ;
#104651=EDGE_LOOP ( 'NONE', ( #235215, #90407, #75718, #195021, #169352 ) ) ;
#104661=CARTESIAN_POINT ( 'NONE',  ( -20.85000000000000142, -11.64999999999999858, -33.50000000000000000 ) ) ;
#104664=EDGE_CURVE ( 'NONE', #33536, #170111, #93976, .T. ) ;
#104678=EDGE_CURVE ( 'NONE', #39469, #84969, #117832, .T. ) ;
#104685=CYLINDRICAL_SURFACE ( 'NONE', #174330, 0.09999999999999939493 ) ;
#104710=CIRCLE ( 'NONE', #238015, 0.1000000000000028644 ) ;
#104720=CARTESIAN_POINT ( 'NONE',  ( -18.50000000000000000, 10.29270135740182823, -38.95736188715194714 ) ) ;
#104726=CARTESIAN_POINT ( 'NONE',  ( -20.54999999999999716, 0.000000000000000000, -33.50000000000000000 ) ) ;
#104731=CARTESIAN_POINT ( 'NONE',  ( -21.05000000000000071, 11.74999999999999645, -26.48519422934605672 ) ) ;
#104741=AXIS2_PLACEMENT_3D ( 'NONE', #101585, #224126, #45500 ) ;
#104756=CARTESIAN_POINT ( 'NONE',  ( 20.04142135623730070, 11.65000000000000391, -21.35000000000000142 ) ) ;
#104780=CARTESIAN_POINT ( 'NONE',  ( 21.05000000000000426, 10.56275983745102032, -7.456813957918630109 ) ) ;
#104806=AXIS2_PLACEMENT_3D ( 'NONE', #127899, #187880, #228288 ) ;
#104848=LINE ( 'NONE', #123177, #135126 ) ;
#104878=FACE_OUTER_BOUND ( 'NONE', #247366, .T. ) ;
#104882=ORIENTED_EDGE ( 'NONE', *, *, #225858, .T. ) ;
#104886=VECTOR ( 'NONE', #27253, 1000.000000000000000 ) ;
#104909=AXIS2_PLACEMENT_3D ( 'NONE', #89534, #244756, #28331 ) ;
#104916=ORIENTED_EDGE ( 'NONE', *, *, #34998, .F. ) ;
#104921=CIRCLE ( 'NONE', #125801, 0.1000000000000000472 ) ;
#104955=CYLINDRICAL_SURFACE ( 'NONE', #56235, 0.5000000000000004441 ) ;
#104963=EDGE_CURVE ( 'NONE', #89621, #240969, #14610, .T. ) ;
#105015=FACE_OUTER_BOUND ( 'NONE', #43727, .T. ) ;
#105026=VERTEX_POINT ( 'NONE', #99229 ) ;
#105033=DIRECTION ( 'NONE',  ( 0.000000000000000000, 0.9908441862701596881, -0.1350103645451904977 ) ) ;
#105052=ORIENTED_EDGE ( 'NONE', *, *, #161868, .T. ) ;
#105068=CIRCLE ( 'NONE', #100957, 0.5000000000000022204 ) ;
#105085=DIRECTION ( 'NONE',  ( -0.000000000000000000, -0.000000000000000000, 1.000000000000000000 ) ) ;
#105093=DIRECTION ( 'NONE',  ( 0.000000000000000000, 0.000000000000000000, -1.000000000000000000 ) ) ;
#105108=AXIS2_PLACEMENT_3D ( 'NONE', #133707, #213234, #94576 ) ;
#105120=DIRECTION ( 'NONE',  ( 0.000000000000000000, 0.9908441862701600211, -0.1350103645451876666 ) ) ;
#105132=CARTESIAN_POINT ( 'NONE',  ( -18.51991288638512501, -9.392436789673425324, -7.143266403958832278 ) ) ;
#105148=EDGE_CURVE ( 'NONE', #53603, #174229, #221739, .T. ) ;
#105157=AXIS2_PLACEMENT_3D ( 'NONE', #23334, #62437, #42868 ) ;
#105179=CARTESIAN_POINT ( 'NONE',  ( 20.94999999999999929, 0.000000000000000000, -33.50000000000000000 ) ) ;
#105189=CARTESIAN_POINT ( 'NONE',  ( -20.85000000000000142, -1.135018845910178431, -41.21697688343231647 ) ) ;
#105196=VECTOR ( 'NONE', #118536, 1000.000000000000000 ) ;
#105218=CARTESIAN_POINT ( 'NONE',  ( -18.59999999999999787, 7.021664781900089913, -37.33356540189728889 ) ) ;
#105235=CARTESIAN_POINT ( 'NONE',  ( 23.25000000000000000, 6.550000000000000711, -12.35000000000000320 ) ) ;
#105255=ORIENTED_EDGE ( 'NONE', *, *, #106189, .T. ) ;
#105256=DIRECTION ( 'NONE',  ( 1.000000000000000000, 0.000000000000000000, 0.000000000000000000 ) ) ;
#105334=CARTESIAN_POINT ( 'NONE',  ( 20.02499999999999858, 9.749999999999998224, -21.25000000000000000 ) ) ;
#105339=SPHERICAL_SURFACE ( 'NONE', #246879, 0.1000000000000000056 ) ;
#105343=CARTESIAN_POINT ( 'NONE',  ( -22.39999999999999858, 0.09999999999999939493, 7.790779598373403836 ) ) ;
#105361=DIRECTION ( 'NONE',  ( -1.000000000000000000, -0.000000000000000000, -0.000000000000000000 ) ) ;
#105421=ORIENTED_EDGE ( 'NONE', *, *, #202651, .T. ) ;
#105467=AXIS2_PLACEMENT_3D ( 'NONE', #27603, #252685, #246603 ) ;
#105479=ORIENTED_EDGE ( 'NONE', *, *, #147841, .T. ) ;
#105510=CARTESIAN_POINT ( 'NONE',  ( -18.50000000000000000, -1.164121893241208960, -41.21484808557161017 ) ) ;
#105556=DIRECTION ( 'NONE',  ( 0.000000000000000000, 0.000000000000000000, 1.000000000000000000 ) ) ;
#105558=EDGE_CURVE ( 'NONE', #84692, #53603, #148018, .T. ) ;
#105594=CARTESIAN_POINT ( 'NONE',  ( -22.47071067811865319, 7.720074744498064412, 0.09909245470260744093 ) ) ;
#105600=ORIENTED_EDGE ( 'NONE', *, *, #185221, .T. ) ;
#105603=CIRCLE ( 'NONE', #234636, 0.2000000000000005107 ) ;
#105611=AXIS2_PLACEMENT_3D ( 'NONE', #206270, #204962, #22517 ) ;
#105614=CIRCLE ( 'NONE', #84757, 0.09999999999999843736 ) ;
#105627=ORIENTED_EDGE ( 'NONE', *, *, #32660, .T. ) ;
#105680=DIRECTION ( 'NONE',  ( -0.000000000000000000, -0.000000000000000000, 1.000000000000000000 ) ) ;
#105692=EDGE_CURVE ( 'NONE', #202111, #129010, #110162, .T. ) ;
#105693=CARTESIAN_POINT ( 'NONE',  ( 18.42555734704283310, -9.497158361936710591, -7.039830497734937076 ) ) ;
#105700=DIRECTION ( 'NONE',  ( 0.000000000000000000, -0.9915357197604853789, 0.1298341882520022694 ) ) ;
#105703=CARTESIAN_POINT ( 'NONE',  ( -21.05000000000000071, 6.497017786431962705, -0.01454569056942280232 ) ) ;
#105721=EDGE_CURVE ( 'NONE', #225666, #56536, #174041, .T. ) ;
#105725=VECTOR ( 'NONE', #43646, 999.9999999999998863 ) ;
#105761=EDGE_LOOP ( 'NONE', ( #77694, #10136 ) ) ;
#105823=VECTOR ( 'NONE', #135107, 1000.000000000000000 ) ;
#105829=CARTESIAN_POINT ( 'NONE',  ( 18.59999999999999076, 1.835341550224411922, -11.65515129256298010 ) ) ;
#105839=DIRECTION ( 'NONE',  ( -1.000000000000000000, 0.000000000000000000, -0.000000000000000000 ) ) ;
#105845=ORIENTED_EDGE ( 'NONE', *, *, #215010, .T. ) ;
#105872=EDGE_CURVE ( 'NONE', #188675, #202242, #140490, .T. ) ;
#105886=DIRECTION ( 'NONE',  ( -1.000000000000000000, 0.000000000000000000, 0.000000000000000000 ) ) ;
#105911=VERTEX_POINT ( 'NONE', #227241 ) ;
#105916=ORIENTED_EDGE ( 'NONE', *, *, #208897, .T. ) ;
#105929=CARTESIAN_POINT ( 'NONE',  ( -23.15000000000000213, 4.349999999999999645, -21.25000000000000000 ) ) ;
#105990=VERTEX_POINT ( 'NONE', #30349 ) ;
#106000=CARTESIAN_POINT ( 'NONE',  ( -20.64999999999999858, -9.000000000000003553, -9.893969122652444881 ) ) ;
#106009=DIRECTION ( 'NONE',  ( 0.000000000000000000, -0.4999999999999994449, -0.8660254037844390407 ) ) ;
#106017=CARTESIAN_POINT ( 'NONE',  ( -18.50211644919735576, 10.30207779524867284, -38.98955207167824000 ) ) ;
#106021=AXIS2_PLACEMENT_3D ( 'NONE', #59784, #19413, #178507 ) ;
#106024=DIRECTION ( 'NONE',  ( 0.000000000000000000, 0.000000000000000000, 1.000000000000000000 ) ) ;
#106030=CARTESIAN_POINT ( 'NONE',  ( 20.94999999999999929, 5.399999999999998579, -12.40526601891309788 ) ) ;
#106048=CARTESIAN_POINT ( 'NONE',  ( 20.85000000000000142, 11.75000000000000355, -26.71613433702190932 ) ) ;
#106076=AXIS2_PLACEMENT_3D ( 'NONE', #226310, #223752, #206777 ) ;
#106095=EDGE_CURVE ( 'NONE', #248248, #87594, #73345, .T. ) ;
#106103=VERTEX_POINT ( 'NONE', #249394 ) ;
#106107=CIRCLE ( 'NONE', #6159, 0.09999999999999939493 ) ;
#106129=EDGE_CURVE ( 'NONE', #255042, #108803, #173754, .T. ) ;
#106172=LINE ( 'NONE', #241846, #87604 ) ;
#106189=EDGE_CURVE ( 'NONE', #143318, #67614, #32396, .T. ) ;
#106212=ORIENTED_EDGE ( 'NONE', *, *, #64920, .T. ) ;
#106242=DIRECTION ( 'NONE',  ( 0.000000000000000000, 0.000000000000000000, -1.000000000000000000 ) ) ;
#106246=COLOUR_RGB ( '', 0.09019608, 0.27058824, 0.51372549) ;
#106255=DIRECTION ( 'NONE',  ( 1.000000000000000000, -0.000000000000000000, -0.000000000000000000 ) ) ;
#106257=FACE_OUTER_BOUND ( 'NONE', #59253, .T. ) ;
#106265=VERTEX_POINT ( 'NONE', #183968 ) ;
#106273=CYLINDRICAL_SURFACE ( 'NONE', #95034, 3.999999999999996447 ) ;
#106294=EDGE_LOOP ( 'NONE', ( #144381, #139751, #106452, #10739 ) ) ;
#106299=VERTEX_POINT ( 'NONE', #47000 ) ;
#106309=DIRECTION ( 'NONE',  ( 0.7071359030027680737, 0.7070776581709111719, 0.000000000000000000 ) ) ;
#106325=VERTEX_POINT ( 'NONE', #221779 ) ;
#106334=EDGE_CURVE ( 'NONE', #126780, #51098, #135953, .T. ) ;
#106346=DIRECTION ( 'NONE',  ( 1.000000000000000000, 7.304098846218134667E-16, 0.000000000000000000 ) ) ;
#106356=DIRECTION ( 'NONE',  ( 0.000000000000000000, 0.000000000000000000, 1.000000000000000000 ) ) ;
#106373=DIRECTION ( 'NONE',  ( -2.827886303505249259E-16, 0.8660254037844412611, 0.4999999999999956701 ) ) ;
#106388=CIRCLE ( 'NONE', #256183, 0.1000000000000028644 ) ;
#106391=CARTESIAN_POINT ( 'NONE',  ( 20.86777300164945004, 10.33200063079656417, -39.09316749566428939 ) ) ;
#106441=DIRECTION ( 'NONE',  ( -1.836970198721029934E-16, 1.000000000000000000, 0.000000000000000000 ) ) ;
#106452=ORIENTED_EDGE ( 'NONE', *, *, #177489, .F. ) ;
#106473=DIRECTION ( 'NONE',  ( 0.000000000000000000, 0.000000000000000000, -1.000000000000000000 ) ) ;
#106484=DIRECTION ( 'NONE',  ( 0.7071067811865474617, 0.7071067811865474617, 0.000000000000000000 ) ) ;
#106499=ORIENTED_EDGE ( 'NONE', *, *, #193367, .T. ) ;
#106538=CARTESIAN_POINT ( 'NONE',  ( -23.25000000000000000, 11.65000000000000036, -21.34999999999999787 ) ) ;
#106542=VECTOR ( 'NONE', #182078, 1000.000000000000000 ) ;
#106596=CIRCLE ( 'NONE', #110903, 0.09999999999999939493 ) ;
#106607=ORIENTED_EDGE ( 'NONE', *, *, #89079, .T. ) ;
#106654=VERTEX_POINT ( 'NONE', #207083 ) ;
#106664=SPHERICAL_SURFACE ( 'NONE', #105157, 0.1000000000000000056 ) ;
#106667=DIRECTION ( 'NONE',  ( 1.000000000000000000, -3.965082230804126670E-15, 0.000000000000000000 ) ) ;
#106668=EDGE_LOOP ( 'NONE', ( #87609, #126324, #3012, #196687 ) ) ;
#106692=CARTESIAN_POINT ( 'NONE',  ( 21.98333005346336577, 0.000000000000000000, 7.374075329056667627 ) ) ;
#106735=EDGE_CURVE ( 'NONE', #19733, #109777, #117015, .T. ) ;
#106742=FACE_OUTER_BOUND ( 'NONE', #89530, .T. ) ;
#106746=CARTESIAN_POINT ( 'NONE',  ( -20.94999999999999929, -1.164121893241208960, -41.41484808557160591 ) ) ;
#106760=DIRECTION ( 'NONE',  ( -0.000000000000000000, 0.8660254037844502539, 0.4999999999999799050 ) ) ;
#106788=VERTEX_POINT ( 'NONE', #135220 ) ;
#106791=AXIS2_PLACEMENT_3D ( 'NONE', #36663, #154062, #97851 ) ;
#106801=LINE ( 'NONE', #67686, #151450 ) ;
#106837=CARTESIAN_POINT ( 'NONE',  ( 19.83283456528359423, 11.75000000000000711, -24.84999999941982551 ) ) ;
#106840=DIRECTION ( 'NONE',  ( -1.000000000000000000, 0.000000000000000000, 0.000000000000000000 ) ) ;
#106865=CARTESIAN_POINT ( 'NONE',  ( -22.59999985501179154, 11.74986979300298806, 0.06559866979945758181 ) ) ;
#106867=TOROIDAL_SURFACE ( 'NONE', #215020, 0.9750000000000019762, 0.1000000000000000056 ) ;
#106868=DIRECTION ( 'NONE',  ( 0.000000000000000000, 0.000000000000000000, -1.000000000000000000 ) ) ;
#106884=EDGE_CURVE ( 'NONE', #31072, #172386, #82931, .T. ) ;
#106931=ORIENTED_EDGE ( 'NONE', *, *, #103425, .T. ) ;
#106938=CARTESIAN_POINT ( 'NONE',  ( 21.05000000000000071, 14.05000000000000071, -27.98630492923908619 ) ) ;
#106960=CARTESIAN_POINT ( 'NONE',  ( 20.94999999999999929, 6.550000000000000711, -12.24999999999999289 ) ) ;
#106964=ORIENTED_EDGE ( 'NONE', *, *, #226880, .F. ) ;
#106983=CARTESIAN_POINT ( 'NONE',  ( -22.50000000000000000, 0.09999999999999939493, 0.000000000000000000 ) ) ;
#106998=VERTEX_POINT ( 'NONE', #43846 ) ;
#107004=CARTESIAN_POINT ( 'NONE',  ( -18.59999999999999787, -1.261786168565025568, -8.086498963545480478 ) ) ;
#107032=ADVANCED_FACE ( 'NONE', ( #65971 ), #200351, .T. ) ;
#107057=ADVANCED_FACE ( 'NONE', ( #110221 ), #199327, .T. ) ;
#107077=EDGE_CURVE ( 'NONE', #126171, #158135, #16181, .T. ) ;
#107088=EDGE_CURVE ( 'NONE', #232204, #41537, #185915, .T. ) ;
#107141=VECTOR ( 'NONE', #242364, 1000.000000000000000 ) ;
#107143=ADVANCED_FACE ( 'NONE', ( #13692 ), #29452, .T. ) ;
#107149=ORIENTED_EDGE ( 'NONE', *, *, #6525, .F. ) ;
#107157=VECTOR ( 'NONE', #152360, 1000.000000000000000 ) ;
#107187=AXIS2_PLACEMENT_3D ( 'NONE', #205514, #223790, #66015 ) ;
#107316=CARTESIAN_POINT ( 'NONE',  ( 23.14999999999999503, 11.75000000000000000, -21.25000000000000000 ) ) ;
#107317=CARTESIAN_POINT ( 'NONE',  ( -23.15000000000000213, -8.663551401869161950, -9.524101118067305194 ) ) ;
#107333=DIRECTION ( 'NONE',  ( 0.000000000000000000, -0.4999999999999863998, 0.8660254037844464792 ) ) ;
#107336=ADVANCED_FACE ( 'NONE', ( #202295 ), #5342, .T. ) ;
#107338=VECTOR ( 'NONE', #129574, 1000.000000000000114 ) ;
#107366=DIRECTION ( 'NONE',  ( -0.000000000000000000, -1.000000000000000000, 6.308085367188393199E-16 ) ) ;
#107375=DIRECTION ( 'NONE',  ( 0.000000000000000000, 1.000000000000000000, 0.000000000000000000 ) ) ;
#107381=EDGE_CURVE ( 'NONE', #97348, #5738, #208372, .T. ) ;
#107388=CIRCLE ( 'NONE', #211448, 0.09999999999999939493 ) ;
#107400=CARTESIAN_POINT ( 'NONE',  ( -20.64999999999999858, 4.250000000000000000, -12.35000000000000142 ) ) ;
#107410=CIRCLE ( 'NONE', #36709, 0.1000000000000008799 ) ;
#107519=FACE_BOUND ( 'NONE', #109500, .T. ) ;
#107544=ORIENTED_EDGE ( 'NONE', *, *, #231246, .T. ) ;
#107550=CARTESIAN_POINT ( 'NONE',  ( -21.05000000000000071, -11.48912529307605546, -30.59999999999999432 ) ) ;
#107559=AXIS2_PLACEMENT_3D ( 'NONE', #90313, #227264, #188154 ) ;
#107645=CIRCLE ( 'NONE', #253399, 0.09999999999999993616 ) ;
#107669=ADVANCED_FACE ( 'NONE', ( #31022 ), #54396, .F. ) ;
#107673=FACE_OUTER_BOUND ( 'NONE', #48404, .T. ) ;
#107678=EDGE_CURVE ( 'NONE', #129336, #138911, #46202, .T. ) ;
#107690=VECTOR ( 'NONE', #166116, 1000.000000000000000 ) ;
#107693=CARTESIAN_POINT ( 'NONE',  ( 20.84999999999998721, 10.33248238082518711, -39.09484654391314962 ) ) ;
#107696=VERTEX_POINT ( 'NONE', #251304 ) ;
#107703=CARTESIAN_POINT ( 'NONE',  ( 21.05000005001280172, 8.871279691770906695, -12.17794758824605239 ) ) ;
#107708=CARTESIAN_POINT ( 'NONE',  ( -20.54999999999999716, 2.499999999999998668, -20.27537807723789953 ) ) ;
#107719=DIRECTION ( 'NONE',  ( 0.000000000000000000, 0.000000000000000000, -1.000000000000000000 ) ) ;
#107753=VECTOR ( 'NONE', #56071, 1000.000000000000000 ) ;
#107759=EDGE_LOOP ( 'NONE', ( #84903, #91204, #41973, #237527 ) ) ;
#107792=DIRECTION ( 'NONE',  ( 1.000000000000000000, 0.000000000000000000, 0.000000000000000000 ) ) ;
#107793=ORIENTED_EDGE ( 'NONE', *, *, #197743, .F. ) ;
#107797=CIRCLE ( 'NONE', #241105, 0.1999999999999987899 ) ;
#107809=ORIENTED_EDGE ( 'NONE', *, *, #54355, .F. ) ;
#107819=DIRECTION ( 'NONE',  ( 1.000000000000000000, 0.000000000000000000, -0.000000000000000000 ) ) ;
#107823=VERTEX_POINT ( 'NONE', #97340 ) ;
#107827=AXIS2_PLACEMENT_3D ( 'NONE', #115397, #69883, #132406 ) ;
#107835=DIRECTION ( 'NONE',  ( -1.000000000000000000, 0.000000000000000000, 0.000000000000000000 ) ) ;
#107867=AXIS2_PLACEMENT_3D ( 'NONE', #156717, #112432, #236211 ) ;
#107887=CARTESIAN_POINT ( 'NONE',  ( -18.59999999999999787, 6.846123162352588665, -37.23772626684986164 ) ) ;
#107909=CARTESIAN_POINT ( 'NONE',  ( 23.24999999999999289, 11.65000000000000746, -0.1000000000000028644 ) ) ;
#107917=EDGE_LOOP ( 'NONE', ( #183651, #100749, #40134, #180465 ) ) ;
#107950=EDGE_CURVE ( 'NONE', #123338, #71514, #52523, .T. ) ;
#107960=CYLINDRICAL_SURFACE ( 'NONE', #19981, 0.1000000000000008105 ) ;
#107979=CARTESIAN_POINT ( 'NONE',  ( 21.11747605621531321, 8.778708005492896760, -12.24456316978977988 ) ) ;
#107989=EDGE_CURVE ( 'NONE', #113573, #146959, #60896, .T. ) ;
#108030=VERTEX_POINT ( 'NONE', #48946 ) ;
#108057=ORIENTED_EDGE ( 'NONE', *, *, #185047, .T. ) ;
#108062=DIRECTION ( 'NONE',  ( 0.000000000000000000, -0.9915357197604882655, 0.1298341882519793711 ) ) ;
#108109=DIRECTION ( 'NONE',  ( 1.000000000000000000, -0.000000000000000000, -0.000000000000000000 ) ) ;
#108114=ORIENTED_EDGE ( 'NONE', *, *, #16516, .F. ) ;
#108139=CARTESIAN_POINT ( 'NONE',  ( 19.86930884467583525, 11.68691006697099866, -24.73922263893871332 ) ) ;
#108211=ORIENTED_EDGE ( 'NONE', *, *, #42276, .T. ) ;
#108224=ORIENTED_EDGE ( 'NONE', *, *, #219539, .T. ) ;
#108228=EDGE_CURVE ( 'NONE', #127360, #254325, #252621, .T. ) ;
#108260=ORIENTED_EDGE ( 'NONE', *, *, #164510, .F. ) ;
#108266=CARTESIAN_POINT ( 'NONE',  ( -23.25000000000000000, 0.000000000000000000, 0.000000000000000000 ) ) ;
#108272=ORIENTED_EDGE ( 'NONE', *, *, #56353, .F. ) ;
#108290=FACE_OUTER_BOUND ( 'NONE', #44105, .T. ) ;
#108298=CARTESIAN_POINT ( 'NONE',  ( -21.11833042828136442, 0.007100509059333399813, 6.445644693855379082 ) ) ;
#108302=VECTOR ( 'NONE', #237029, 999.9999999999998863 ) ;
#108303=CARTESIAN_POINT ( 'NONE',  ( 18.47654891039379166, -9.465274948382308651, -7.125975905194652960 ) ) ;
#108311=FACE_OUTER_BOUND ( 'NONE', #66164, .T. ) ;
#108312=LINE ( 'NONE', #186575, #144191 ) ;
#108350=VERTEX_POINT ( 'NONE', #106030 ) ;
#108354=ORIENTED_EDGE ( 'NONE', *, *, #67476, .T. ) ;
#108390=DIRECTION ( 'NONE',  ( 0.000000000000000000, 0.9908441862701596881, 0.1350103645451904977 ) ) ;
#108404=VERTEX_POINT ( 'NONE', #231168 ) ;
#108407=FACE_OUTER_BOUND ( 'NONE', #95582, .T. ) ;
#108419=ORIENTED_EDGE ( 'NONE', *, *, #142174, .T. ) ;
#108425=ORIENTED_EDGE ( 'NONE', *, *, #219331, .T. ) ;
#108435=AXIS2_PLACEMENT_3D ( 'NONE', #233525, #195692, #54848 ) ;
#108457=ORIENTED_EDGE ( 'NONE', *, *, #49953, .F. ) ;
#108465=EDGE_LOOP ( 'NONE', ( #181721, #229124, #153203, #147544, #98193 ) ) ;
#108515=EDGE_CURVE ( 'NONE', #135260, #124226, #127751, .T. ) ;
#108520=ORIENTED_EDGE ( 'NONE', *, *, #14360, .F. ) ;
#108524=DIRECTION ( 'NONE',  ( 0.000000000000000000, -1.000000000000000000, 0.000000000000000000 ) ) ;
#108561=FACE_OUTER_BOUND ( 'NONE', #249468, .T. ) ;
#108571=DIRECTION ( 'NONE',  ( 0.000000000000000000, 0.000000000000000000, -1.000000000000000000 ) ) ;
#108574=LINE ( 'NONE', #12068, #22292 ) ;
#108579=ORIENTED_EDGE ( 'NONE', *, *, #113984, .F. ) ;
#108581=ORIENTED_EDGE ( 'NONE', *, *, #124467, .F. ) ;
#108590=CIRCLE ( 'NONE', #175270, 0.09999999999999954758 ) ;
#108607=EDGE_CURVE ( 'NONE', #167773, #11322, #144659, .T. ) ;
#108608=DIRECTION ( 'NONE',  ( 0.000000000000000000, -1.000000000000000000, 0.000000000000000000 ) ) ;
#108621=EDGE_LOOP ( 'NONE', ( #169595, #7891, #158712, #19926 ) ) ;
#108672=CIRCLE ( 'NONE', #192082, 0.5000000000000022204 ) ;
#108706=CIRCLE ( 'NONE', #146287, 0.09999999999999939493 ) ;
#108780=DIRECTION ( 'NONE',  ( 0.000000000000000000, 0.4930308989875324399, 0.8700118002898268310 ) ) ;
#108794=ORIENTED_EDGE ( 'NONE', *, *, #214807, .F. ) ;
#108803=VERTEX_POINT ( 'NONE', #33649 ) ;
#108817=CIRCLE ( 'NONE', #25452, 11.70000000000000462 ) ;
#108823=CIRCLE ( 'NONE', #17274, 0.09999999999999982514 ) ;
#108827=DIRECTION ( 'NONE',  ( -1.000000000000000000, -0.000000000000000000, -0.000000000000000000 ) ) ;
#108840=EDGE_LOOP ( 'NONE', ( #54649, #12039, #187606, #53748 ) ) ;
#108844=CARTESIAN_POINT ( 'NONE',  ( 20.94999999999999929, 0.000000000000000000, -33.50000000000000000 ) ) ;
#108858=CARTESIAN_POINT ( 'NONE',  ( 18.59999999999998366, 7.021664781900089913, -37.33356540189728889 ) ) ;
#108877=ORIENTED_EDGE ( 'NONE', *, *, #57104, .F. ) ;
#108892=PLANE ( 'NONE',  #112023 ) ;
#108902=CARTESIAN_POINT ( 'NONE',  ( -21.05000000000000071, 5.021051876504147385E-16, -37.60000000000000142 ) ) ;
#108944=CARTESIAN_POINT ( 'NONE',  ( 19.58285714285715073, 9.015001489648581057, -8.420652816081712899 ) ) ;
#108980=CARTESIAN_POINT ( 'NONE',  ( -18.59999999999999787, 11.64999999999999680, -7.014805770653998351 ) ) ;
#108982=ORIENTED_EDGE ( 'NONE', *, *, #75123, .F. ) ;
#108995=EDGE_CURVE ( 'NONE', #75474, #78587, #238202, .T. ) ;
#109007=CIRCLE ( 'NONE', #67326, 0.09999999999999939493 ) ;
#109015=CARTESIAN_POINT ( 'NONE',  ( -18.50000000000001066, -9.421308209739168049, -7.242363214050910436 ) ) ;
#109027=ORIENTED_EDGE ( 'NONE', *, *, #83181, .F. ) ;
#109031=VERTEX_POINT ( 'NONE', #159988 ) ;
#109046=CIRCLE ( 'NONE', #254758, 0.09999999999999939493 ) ;
#109050=DIRECTION ( 'NONE',  ( 0.000000000000000000, 0.000000000000000000, -1.000000000000000000 ) ) ;
#109051=EDGE_CURVE ( 'NONE', #226810, #59020, #144226, .T. ) ;
#109147=ORIENTED_EDGE ( 'NONE', *, *, #254102, .F. ) ;
#109177=AXIS2_PLACEMENT_3D ( 'NONE', #258039, #59860, #141982 ) ;
#109220=DIRECTION ( 'NONE',  ( 1.000000000000000000, 0.000000000000000000, 0.000000000000000000 ) ) ;
#109241=DIRECTION ( 'NONE',  ( 0.000000000000000000, 0.000000000000000000, -1.000000000000000000 ) ) ;
#109255=DIRECTION ( 'NONE',  ( 0.000000000000000000, 0.9274965247785529332, -0.3738317757009255171 ) ) ;
#109271=DIRECTION ( 'NONE',  ( 0.000000000000000000, 0.1350103645451904977, -0.9908441862701596881 ) ) ;
#109279=CARTESIAN_POINT ( 'NONE',  ( 21.05000012384952868, 10.62872029887554604, -12.17797733003523497 ) ) ;
#109288=CARTESIAN_POINT ( 'NONE',  ( -18.50000000000000000, 9.150000000000002132, 11.75000000000000000 ) ) ;
#109339=DIRECTION ( 'NONE',  ( 0.000000000000000000, -0.1298341882520022694, -0.9915357197604853789 ) ) ;
#109344=ORIENTED_EDGE ( 'NONE', *, *, #145562, .T. ) ;
#109361=FACE_OUTER_BOUND ( 'NONE', #198611, .T. ) ;
#109383=DIRECTION ( 'NONE',  ( 1.000000000000000000, 0.000000000000000000, 0.000000000000000000 ) ) ;
#109389=VECTOR ( 'NONE', #6354, 1000.000000000000000 ) ;
#109402=CARTESIAN_POINT ( 'NONE',  ( 19.90621891164687440, 11.75000000000000711, -24.82844527787753464 ) ) ;
#109425=ORIENTED_EDGE ( 'NONE', *, *, #14446, .T. ) ;
#109427=DIRECTION ( 'NONE',  ( -1.000000000000000000, 0.000000000000000000, 0.000000000000000000 ) ) ;
#109469=VERTEX_POINT ( 'NONE', #184334 ) ;
#109500=EDGE_LOOP ( 'NONE', ( #194688, #223049 ) ) ;
#109519=CARTESIAN_POINT ( 'NONE',  ( -18.59999999999999787, 0.000000000000000000, 0.000000000000000000 ) ) ;
#109526=CARTESIAN_POINT ( 'NONE',  ( -20.94999999999999929, -1.835341550224411922, -11.65515129256298010 ) ) ;
#109535=CARTESIAN_POINT ( 'NONE',  ( 20.85000000000000142, -1.835859311443637010, -45.10443916879852821 ) ) ;
#109543=ORIENTED_EDGE ( 'NONE', *, *, #218099, .F. ) ;
#109636=CARTESIAN_POINT ( 'NONE',  ( 20.94999999999999574, -1.261786168565025568, -8.086498963545480478 ) ) ;
#109661=DIRECTION ( 'NONE',  ( 4.239556034732056743E-17, -0.1298341882520022694, -0.9915357197604852679 ) ) ;
#109670=ADVANCED_FACE ( 'NONE', ( #77225 ), #237604, .T. ) ;
#109673=CIRCLE ( 'NONE', #9717, 0.1000000000000008799 ) ;
#109718=AXIS2_PLACEMENT_3D ( 'NONE', #83369, #144644, #121288 ) ;
#109729=AXIS2_PLACEMENT_3D ( 'NONE', #177566, #257010, #82238 ) ;
#109749=FACE_OUTER_BOUND ( 'NONE', #211296, .T. ) ;
#109763=AXIS2_PLACEMENT_3D ( 'NONE', #240325, #82488, #139905 ) ;
#109777=VERTEX_POINT ( 'NONE', #238887 ) ;
#109787=EDGE_CURVE ( 'NONE', #256245, #45832, #82637, .T. ) ;
#109824=AXIS2_PLACEMENT_3D ( 'NONE', #63344, #144161, #91599 ) ;
#109879=FACE_OUTER_BOUND ( 'NONE', #100845, .T. ) ;
#109915=CARTESIAN_POINT ( 'NONE',  ( 21.05000000000000071, 11.60000000000000497, -26.57179676972450366 ) ) ;
#109931=EDGE_LOOP ( 'NONE', ( #224309, #127110, #101292, #187754 ) ) ;
#109939=ORIENTED_EDGE ( 'NONE', *, *, #210130, .F. ) ;
#109977=ORIENTED_EDGE ( 'NONE', *, *, #23992, .F. ) ;
#110015=CARTESIAN_POINT ( 'NONE',  ( -18.59999999999999787, 1.162701749938009677, -8.099999999999999645 ) ) ;
#110021=VECTOR ( 'NONE', #196802, 1000.000000000000000 ) ;
#110023=CARTESIAN_POINT ( 'NONE',  ( 18.50000000000000000, -9.499999999999998224, -40.10018939122205239 ) ) ;
#110028=CARTESIAN_POINT ( 'NONE',  ( -23.25000000000000000, 11.65000000000000036, 11.75000000000000000 ) ) ;
#110069=DIRECTION ( 'NONE',  ( 1.000000000000000000, -0.000000000000000000, -0.000000000000000000 ) ) ;
#110148=DIRECTION ( 'NONE',  ( -1.000000000000000000, 0.000000000000000000, 0.000000000000000000 ) ) ;
#110162=LINE ( 'NONE', #93166, #136017 ) ;
#110178=CARTESIAN_POINT ( 'NONE',  ( 23.14999999999999858, 0.000000000000000000, -33.50000000000000000 ) ) ;
#110205=CARTESIAN_POINT ( 'NONE',  ( 18.59999999999999076, 11.65000000000000391, -33.50000000000000000 ) ) ;
#110221=FACE_OUTER_BOUND ( 'NONE', #189343, .T. ) ;
#110242=DIRECTION ( 'NONE',  ( 0.000000000000000000, 0.000000000000000000, -1.000000000000000000 ) ) ;
#110255=DIRECTION ( 'NONE',  ( -1.000000000000000000, -2.952720810173289112E-16, 0.000000000000000000 ) ) ;
#110270=FACE_OUTER_BOUND ( 'NONE', #123437, .T. ) ;
#110289=EDGE_CURVE ( 'NONE', #256663, #240042, #107797, .T. ) ;
#110293=CARTESIAN_POINT ( 'NONE',  ( 23.14999999999999858, -11.74999999999999112, 11.75000000000000000 ) ) ;
#110294=VECTOR ( 'NONE', #43513, 1000.000000000000000 ) ;
#110296=CARTESIAN_POINT ( 'NONE',  ( -18.59999999999999787, 14.05000000000000071, -5.513695070760990191 ) ) ;
#110348=DIRECTION ( 'NONE',  ( -0.000000000000000000, -0.4791956752371546169, -0.8777080977375152360 ) ) ;
#110376=DIRECTION ( 'NONE',  ( 0.7071067811865474617, 0.7071067811865474617, -0.000000000000000000 ) ) ;
#110378=CARTESIAN_POINT ( 'NONE',  ( -20.94999999999999929, 1.162701749938009677, -7.900000000000000355 ) ) ;
#110397=EDGE_LOOP ( 'NONE', ( #32211, #7882, #108419, #76558 ) ) ;
#110412=VECTOR ( 'NONE', #61718, 1000.000000000000114 ) ;
#110450=CARTESIAN_POINT ( 'NONE',  ( -22.50000000000000000, 11.75000000000000000, -3.469446951953614189E-15 ) ) ;
#110497=CARTESIAN_POINT ( 'NONE',  ( 21.14999999999999858, 10.71339244339988461, -12.25000000000000000 ) ) ;
#110505=AXIS2_PLACEMENT_3D ( 'NONE', #110015, #7062, #207868 ) ;
#110509=CARTESIAN_POINT ( 'NONE',  ( 21.05000000000000071, 8.776282648971246658, -8.487592378520258052 ) ) ;
#110550=VERTEX_POINT ( 'NONE', #244352 ) ;
#110556=CARTESIAN_POINT ( 'NONE',  ( 19.99999999999998934, 11.75000000000000355, -24.85000000000000142 ) ) ;
#110592=AXIS2_PLACEMENT_3D ( 'NONE', #211091, #49450, #32490 ) ;
#110604=EDGE_CURVE ( 'NONE', #191967, #91362, #128848, .T. ) ;
#110615=TOROIDAL_SURFACE ( 'NONE', #243708, 0.6000000000000009770, 0.1000000000000000056 ) ;
#110619=CARTESIAN_POINT ( 'NONE',  ( 20.94999999999999929, 0.000000000000000000, -33.50000000000000000 ) ) ;
#110620=CARTESIAN_POINT ( 'NONE',  ( -20.64999999999999858, 2.399999999999999467, -13.22462192276210224 ) ) ;
#110626=DIRECTION ( 'NONE',  ( -1.000000000000000000, 0.000000000000000000, -3.469446951953635015E-14 ) ) ;
#110635=DIRECTION ( 'NONE',  ( 0.000000000000000000, 0.000000000000000000, 1.000000000000000000 ) ) ;
#110642=LINE ( 'NONE', #149798, #2462 ) ;
#110649=CARTESIAN_POINT ( 'NONE',  ( 20.04142135623730070, 11.65000000000000391, -24.65000000000000213 ) ) ;
#110666=CARTESIAN_POINT ( 'NONE',  ( -21.45000000000000284, 7.708578643762696636, -21.25000000000000000 ) ) ;
#110673=CARTESIAN_POINT ( 'NONE',  ( -21.05000000000000071, 6.540656951701240729, -0.09999999999999939493 ) ) ;
#110725=ORIENTED_EDGE ( 'NONE', *, *, #221183, .T. ) ;
#110743=ORIENTED_EDGE ( 'NONE', *, *, #229460, .T. ) ;
#110749=AXIS2_PLACEMENT_3D ( 'NONE', #249020, #52059, #149922 ) ;
#110772=ORIENTED_EDGE ( 'NONE', *, *, #77516, .T. ) ;
#110775=DIRECTION ( 'NONE',  ( 0.000000000000000000, 0.000000000000000000, 1.000000000000000000 ) ) ;
#110790=ORIENTED_EDGE ( 'NONE', *, *, #178888, .F. ) ;
#110791=EDGE_LOOP ( 'NONE', ( #207311, #160295, #199007, #205560 ) ) ;
#110797=DIRECTION ( 'NONE',  ( 0.000000000000000000, 0.01562500000001058528, 0.9998779222360095753 ) ) ;
#110844=PLANE ( 'NONE',  #211773 ) ;
#110875=CARTESIAN_POINT ( 'NONE',  ( -21.05000000000000071, 6.300179817914679070, 0.05148288188165942719 ) ) ;
#110903=AXIS2_PLACEMENT_3D ( 'NONE', #215817, #179312, #257473 ) ;
#110940=VECTOR ( 'NONE', #238095, 1000.000000000000000 ) ;
#110945=EDGE_CURVE ( 'NONE', #71883, #64464, #53443, .T. ) ;
#110958=DIRECTION ( 'NONE',  ( 0.000000000000000000, 0.8660254037844309360, -0.5000000000000134337 ) ) ;
#110962=AXIS2_PLACEMENT_3D ( 'NONE', #51231, #33034, #27884 ) ;
#111006=VERTEX_POINT ( 'NONE', #135823 ) ;
#111016=CIRCLE ( 'NONE', #131861, 0.1000000000000028644 ) ;
#111020=EDGE_CURVE ( 'NONE', #40483, #232204, #165887, .T. ) ;
#111021=ORIENTED_EDGE ( 'NONE', *, *, #2894, .F. ) ;
#111029=CARTESIAN_POINT ( 'NONE',  ( -21.13614978966382196, 6.499104701833789299, 1.201516235680224439E-15 ) ) ;
#111030=CARTESIAN_POINT ( 'NONE',  ( 23.24999999999999289, 11.65000000000000746, -12.15000000000000036 ) ) ;
#111039=CARTESIAN_POINT ( 'NONE',  ( -21.05000000000000071, 5.204170427930421283E-15, -2.899999999999982592 ) ) ;
#111048=AXIS2_PLACEMENT_3D ( 'NONE', #240672, #122014, #140266 ) ;
#111081=EDGE_CURVE ( 'NONE', #126038, #6193, #24415, .T. ) ;
#111097=ADVANCED_FACE ( 'NONE', ( #123995 ), #243918, .T. ) ;
#111102=VECTOR ( 'NONE', #121109, 1000.000000000000000 ) ;
#111120=TOROIDAL_SURFACE ( 'NONE', #136030, 11.90000000000000213, 0.1000000000000000056 ) ;
#111164=CARTESIAN_POINT ( 'NONE',  ( -20.54999999999999716, 0.000000000000000000, -33.50000000000000000 ) ) ;
#111165=ORIENTED_EDGE ( 'NONE', *, *, #204096, .T. ) ;
#111183=DIRECTION ( 'NONE',  ( -1.000000000000000000, 0.000000000000000000, 0.000000000000000000 ) ) ;
#111190=DIRECTION ( 'NONE',  ( 1.000000000000000000, -0.000000000000000000, -0.000000000000000000 ) ) ;
#111214=CARTESIAN_POINT ( 'NONE',  ( 20.94999999999999929, 11.74999999999999822, -26.71613433702190932 ) ) ;
#111259=DIRECTION ( 'NONE',  ( 0.000000000000000000, -0.9908441862701644620, 0.1350103645451558587 ) ) ;
#111305=CARTESIAN_POINT ( 'NONE',  ( -20.54999999999999716, 0.000000000000000000, -33.50000000000000000 ) ) ;
#111339=DIRECTION ( 'NONE',  ( 1.000000000000000000, 3.265361837132813093E-16, -0.000000000000000000 ) ) ;
#111345=CARTESIAN_POINT ( 'NONE',  ( 20.94999999999999929, 0.000000000000000000, -33.50000000000000000 ) ) ;
#111360=EDGE_CURVE ( 'NONE', #244742, #220385, #57871, .T. ) ;
#111362=CIRCLE ( 'NONE', #3194, 12.77500000000000036 ) ;
#111370=EDGE_LOOP ( 'NONE', ( #215076, #224016, #121094, #208388 ) ) ;
#111403=DIRECTION ( 'NONE',  ( 0.000000000000000000, -0.9915357197604882655, 0.1298341882519793711 ) ) ;
#111423=CARTESIAN_POINT ( 'NONE',  ( 20.94999999999999574, -1.851028230140860487, -11.65391326942249250 ) ) ;
#111425=EDGE_CURVE ( 'NONE', #163009, #224530, #256713, .T. ) ;
#111457=ADVANCED_FACE ( 'NONE', ( #100227 ), #112079, .F. ) ;
#111463=EDGE_CURVE ( 'NONE', #65265, #224530, #253514, .T. ) ;
#111465=AXIS2_PLACEMENT_3D ( 'NONE', #85368, #120710, #161107 ) ;
#111470=B_SPLINE_CURVE_WITH_KNOTS ( 'NONE', 3,
 ( #79853, #83687, #223228, #336, #163285, #159438, #181572, #244082, #184108, #139842, #141151, #203684, #25071, #42059, #220682, #104545, #82416, #5453, #84981 ),
 .UNSPECIFIED., .F., .F.,
 ( 4, 3, 3, 3, 3, 3, 4 ),
 ( -2.000416914658901521E-06, 0.000000000000000000, 4.714008503744565809E-05, 9.979203887777271477E-05, 0.0001372215519229478891, 0.0001635031576220937453, 0.0001900083748504128364 ),
 .UNSPECIFIED. ) ;
#111482=LINE ( 'NONE', #150614, #98989 ) ;
#111503=( BOUNDED_CURVE ( )  B_SPLINE_CURVE ( 3, ( #80173, #99748, #180601, #178048 ),
 .UNSPECIFIED., .F., .F. ) 
 B_SPLINE_CURVE_WITH_KNOTS ( ( 4, 4 ),
 ( 0.000000000000000000, 1.570796326794908992 ),
 .UNSPECIFIED. ) 
 CURVE ( )  GEOMETRIC_REPRESENTATION_ITEM ( )  RATIONAL_B_SPLINE_CURVE ( ( 1.000000000000000000, 0.8047378541243619399, 0.8047378541243619399, 1.000000000000000000 ) ) 
 REPRESENTATION_ITEM ( '' )  );
#111506=AXIS2_PLACEMENT_3D ( 'NONE', #157488, #236994, #131471 ) ;
#111537=CARTESIAN_POINT ( 'NONE',  ( -20.64999999999999858, 7.150000000000000355, -12.34999999999999964 ) ) ;
#111543=AXIS2_PLACEMENT_3D ( 'NONE', #15634, #52141, #95136 ) ;
#111546=AXIS2_PLACEMENT_3D ( 'NONE', #20740, #19445, #200647 ) ;
#111557=CARTESIAN_POINT ( 'NONE',  ( -20.54999999999999716, -9.000000000000003553, -9.893969122652444881 ) ) ;
#111571=PLANE ( 'NONE',  #167169 ) ;
#111598=CARTESIAN_POINT ( 'NONE',  ( 20.94999999999999929, 10.47338541491290265, -7.578654464248539391 ) ) ;
#111606=ORIENTED_EDGE ( 'NONE', *, *, #95875, .T. ) ;
#111663=AXIS2_PLACEMENT_3D ( 'NONE', #104592, #88900, #167207 ) ;
#111677=EDGE_CURVE ( 'NONE', #244526, #34172, #49709, .T. ) ;
#111693=VECTOR ( 'NONE', #52653, 1000.000000000000000 ) ;
#111696=DIRECTION ( 'NONE',  ( 0.000000000000000000, 0.000000000000000000, -1.000000000000000000 ) ) ;
#111702=LINE ( 'NONE', #75169, #197546 ) ;
#111709=CARTESIAN_POINT ( 'NONE',  ( -22.37643362114956957, 0.09908137368138361656, 7.625789993958400181 ) ) ;
#111743=PLANE ( 'NONE',  #191314 ) ;
#111755=LINE ( 'NONE', #192576, #150827 ) ;
#111762=ORIENTED_EDGE ( 'NONE', *, *, #101390, .F. ) ;
#111847=VECTOR ( 'NONE', #62678, 1000.000000000000000 ) ;
#111852=DIRECTION ( 'NONE',  ( 2.952720810173289112E-16, -1.000000000000000000, 0.000000000000000000 ) ) ;
#111863=CARTESIAN_POINT ( 'NONE',  ( 20.85000000000000142, 7.021664781900089913, -37.33356540189728889 ) ) ;
#111867=EDGE_CURVE ( 'NONE', #185056, #146767, #230261, .T. ) ;
#111888=VERTEX_POINT ( 'NONE', #47334 ) ;
#111905=CARTESIAN_POINT ( 'NONE',  ( -23.25000000000000000, 0.000000000000000000, -33.50000000000000000 ) ) ;
#111943=CARTESIAN_POINT ( 'NONE',  ( -21.55000000000000426, 7.750000000000000000, -12.34999999999999964 ) ) ;
#111994=AXIS2_PLACEMENT_3D ( 'NONE', #205418, #247114, #106309 ) ;
#111995=ADVANCED_FACE ( 'NONE', ( #150326 ), #179102, .F. ) ;
#111997=DIRECTION ( 'NONE',  ( 1.000000000000000000, -0.000000000000000000, 0.000000000000000000 ) ) ;
#112023=AXIS2_PLACEMENT_3D ( 'NONE', #187176, #151906, #52761 ) ;
#112049=PLANE ( 'NONE',  #130519 ) ;
#112057=VECTOR ( 'NONE', #22786, 1000.000000000000000 ) ;
#112079=TOROIDAL_SURFACE ( 'NONE', #170368, 0.2000000000000000111, 0.1000000000000000056 ) ;
#112086=VERTEX_POINT ( 'NONE', #78463 ) ;
#112116=DIRECTION ( 'NONE',  ( 1.000000000000000000, 0.000000000000000000, 0.000000000000000000 ) ) ;
#112118=CIRCLE ( 'NONE', #245384, 0.1000000000000002554 ) ;
#112131=ORIENTED_EDGE ( 'NONE', *, *, #19986, .F. ) ;
#112168=LINE ( 'NONE', #173465, #110021 ) ;
#112191=CARTESIAN_POINT ( 'NONE',  ( -23.15000000000000213, -9.000000000000003553, -9.893969122652444881 ) ) ;
#112246=VERTEX_POINT ( 'NONE', #240131 ) ;
#112265=CARTESIAN_POINT ( 'NONE',  ( 18.49999999999999645, 5.699452464321595357, 12.54227395656983290 ) ) ;
#112271=ORIENTED_EDGE ( 'NONE', *, *, #27868, .T. ) ;
#112277=DIRECTION ( 'NONE',  ( 1.000000000000000000, 0.000000000000000000, 0.000000000000000000 ) ) ;
#112285=CARTESIAN_POINT ( 'NONE',  ( -18.59999999999999787, -1.835859311443637010, -45.00443916879852679 ) ) ;
#112310=EDGE_CURVE ( 'NONE', #224010, #101170, #34291, .T. ) ;
#112313=CIRCLE ( 'NONE', #95712, 0.1999999999999987899 ) ;
#112318=CARTESIAN_POINT ( 'NONE',  ( -20.94999999999999929, -11.75000000000000000, -3.100000000000001865 ) ) ;
#112327=CARTESIAN_POINT ( 'NONE',  ( -21.12230431290520016, 6.457566653293005388, 0.005209851689006794913 ) ) ;
#112355=TOROIDAL_SURFACE ( 'NONE', #179023, 4.099999999999999645, 0.1000000000000000056 ) ;
#112362=EDGE_LOOP ( 'NONE', ( #96359, #171385, #169568, #108579 ) ) ;
#112370=DIRECTION ( 'NONE',  ( 1.000000000000000000, 0.000000000000000000, 0.000000000000000000 ) ) ;
#112392=DIRECTION ( 'NONE',  ( 0.000000000000000000, 1.000000000000000000, 0.000000000000000000 ) ) ;
#112416=ORIENTED_EDGE ( 'NONE', *, *, #185215, .T. ) ;
#112421=ORIENTED_EDGE ( 'NONE', *, *, #17747, .T. ) ;
#112432=DIRECTION ( 'NONE',  ( 0.000000000000000000, 0.8660254037844482555, 0.4999999999999837907 ) ) ;
#112457=VERTEX_POINT ( 'NONE', #18200 ) ;
#112458=ORIENTED_EDGE ( 'NONE', *, *, #185047, .F. ) ;
#112460=CARTESIAN_POINT ( 'NONE',  ( -22.50000000000000000, 0.000000000000000000, 0.000000000000000000 ) ) ;
#112469=ORIENTED_EDGE ( 'NONE', *, *, #66503, .F. ) ;
#112494=EDGE_LOOP ( 'NONE', ( #184115, #65304, #12979, #109939, #238042, #3488, #252543, #200295, #102206, #181606, #141408, #131026, #241022, #178301, #153076, #146322, #50143, #131170, #185346, #49128, #175597, #11450, #113866, #178372, #65407, #186523, #108211 ) ) ;
#112499=EDGE_CURVE ( 'NONE', #7751, #243103, #234682, .T. ) ;
#112532=AXIS2_PLACEMENT_3D ( 'NONE', #186879, #90310, #6931 ) ;
#112563=DIRECTION ( 'NONE',  ( 0.000000000000000000, 0.000000000000000000, -1.000000000000000000 ) ) ;
#112565=ORIENTED_EDGE ( 'NONE', *, *, #143454, .F. ) ;
#112584=ORIENTED_EDGE ( 'NONE', *, *, #49650, .T. ) ;
#112622=CYLINDRICAL_SURFACE ( 'NONE', #18667, 0.1000000000000028644 ) ;
#112628=DIRECTION ( 'NONE',  ( 1.000000000000000000, 0.000000000000000000, 0.000000000000000000 ) ) ;
#112655=DIRECTION ( 'NONE',  ( -0.000000000000000000, 0.000000000000000000, -1.000000000000000000 ) ) ;
#112671=ORIENTED_EDGE ( 'NONE', *, *, #176528, .T. ) ;
#112705=DIRECTION ( 'NONE',  ( -1.000000000000000000, -8.673617379884087537E-15, 0.000000000000000000 ) ) ;
#112707=VERTEX_POINT ( 'NONE', #25914 ) ;
#112717=PLANE ( 'NONE',  #234869 ) ;
#112725=AXIS2_PLACEMENT_3D ( 'NONE', #23714, #238880, #223148 ) ;
#112779=DIRECTION ( 'NONE',  ( 1.000000000000000000, 0.000000000000000000, 0.000000000000000000 ) ) ;
#112781=CIRCLE ( 'NONE', #54512, 0.09999999999999939493 ) ;
#112783=ORIENTED_EDGE ( 'NONE', *, *, #94363, .F. ) ;
#112815=CIRCLE ( 'NONE', #67019, 0.1000000000000002554 ) ;
#112832=CIRCLE ( 'NONE', #50269, 0.09999999999999939493 ) ;
#112834=AXIS2_PLACEMENT_3D ( 'NONE', #205460, #26866, #106346 ) ;
#112880=CARTESIAN_POINT ( 'NONE',  ( 21.05000000000000071, 10.48459288119459032, -7.456713570584089013 ) ) ;
#112907=AXIS2_PLACEMENT_3D ( 'NONE', #191777, #153950, #13117 ) ;
#112923=DIRECTION ( 'NONE',  ( 0.000000000000000000, 0.000000000000000000, -1.000000000000000000 ) ) ;
#112963=CIRCLE ( 'NONE', #150562, 11.75000000000000000 ) ;
#112970=ORIENTED_EDGE ( 'NONE', *, *, #56135, .F. ) ;
#112998=CARTESIAN_POINT ( 'NONE',  ( -21.30740335185486245, 0.09893452577585101770, 6.556657922028001906 ) ) ;
#113033=VECTOR ( 'NONE', #62783, 1000.000000000000114 ) ;
#113048=FACE_OUTER_BOUND ( 'NONE', #117283, .T. ) ;
#113100=VERTEX_POINT ( 'NONE', #29477 ) ;
#113131=LINE ( 'NONE', #110556, #148749 ) ;
#113146=CARTESIAN_POINT ( 'NONE',  ( 21.15000000000000213, 10.71339244339988461, -12.25000000000000178 ) ) ;
#113147=ORIENTED_EDGE ( 'NONE', *, *, #128385, .T. ) ;
#113180=EDGE_CURVE ( 'NONE', #94374, #135260, #108706, .T. ) ;
#113182=AXIS2_PLACEMENT_3D ( 'NONE', #75882, #233686, #248418 ) ;
#113188=DIRECTION ( 'NONE',  ( 0.000000000000000000, 0.000000000000000000, -1.000000000000000000 ) ) ;
#113202=CARTESIAN_POINT ( 'NONE',  ( -18.48408745364676520, -9.664322258663098353, -40.18307853332839130 ) ) ;
#113211=VERTEX_POINT ( 'NONE', #151984 ) ;
#113215=ADVANCED_FACE ( 'NONE', ( #51530 ), #153274, .T. ) ;
#113223=DIRECTION ( 'NONE',  ( 0.000000000000000000, -0.1568667991644863147, 0.9876197685951252359 ) ) ;
#113248=CARTESIAN_POINT ( 'NONE',  ( 21.13461538461538325, 8.885417037974459475, -12.35000000000000320 ) ) ;
#113256=AXIS2_PLACEMENT_3D ( 'NONE', #31682, #111190, #85545 ) ;
#113266=EDGE_LOOP ( 'NONE', ( #140652, #196474, #118595, #83925 ) ) ;
#113267=CARTESIAN_POINT ( 'NONE',  ( 18.54271179734059416, -9.624084290098748440, -40.24096485270028012 ) ) ;
#113275=EDGE_CURVE ( 'NONE', #57845, #63069, #165780, .T. ) ;
#113325=EDGE_CURVE ( 'NONE', #254325, #257538, #18854, .T. ) ;
#113333=ORIENTED_EDGE ( 'NONE', *, *, #119255, .F. ) ;
#113339=AXIS2_PLACEMENT_3D ( 'NONE', #55454, #35950, #175467 ) ;
#113340=AXIS2_PLACEMENT_3D ( 'NONE', #225402, #49353, #145871 ) ;
#113341=CARTESIAN_POINT ( 'NONE',  ( -18.59999999999999787, -1.149570369575693807, -41.31591248450196474 ) ) ;
#113369=VERTEX_POINT ( 'NONE', #60539 ) ;
#113406=DIRECTION ( 'NONE',  ( 0.000000000000000000, 0.000000000000000000, -1.000000000000000000 ) ) ;
#113425=EDGE_LOOP ( 'NONE', ( #153754, #244195, #220186, #196950 ) ) ;
#113430=CIRCLE ( 'NONE', #238306, 0.09999999999999939493 ) ;
#113457=ADVANCED_FACE ( 'NONE', ( #210036 ), #694, .F. ) ;
#113464=CARTESIAN_POINT ( 'NONE',  ( 18.58143601961869251, 10.43572941509456342, -24.75000000000000000 ) ) ;
#113465=CARTESIAN_POINT ( 'NONE',  ( -20.94999999999999929, -11.65000000000000036, -30.59999999999999432 ) ) ;
#113467=CARTESIAN_POINT ( 'NONE',  ( -21.14999999999999858, 0.000000000000000000, 0.000000000000000000 ) ) ;
#113495=AXIS2_PLACEMENT_3D ( 'NONE', #48960, #153240, #149380 ) ;
#113498=CARTESIAN_POINT ( 'NONE',  ( -21.55000000000000426, 7.708578643762696636, -12.34999999999999964 ) ) ;
#113506=DIRECTION ( 'NONE',  ( 1.000000000000000000, -0.000000000000000000, -0.000000000000000000 ) ) ;
#113517=CIRCLE ( 'NONE', #75922, 3.999999999999999112 ) ;
#113519=CARTESIAN_POINT ( 'NONE',  ( -18.50000000000000000, 1.162701749938009677, -8.099999999999999645 ) ) ;
#113523=CARTESIAN_POINT ( 'NONE',  ( -22.47071067811865319, 0.09909245470260570621, 7.720074744498060859 ) ) ;
#113525=ORIENTED_EDGE ( 'NONE', *, *, #235477, .T. ) ;
#113529=CARTESIAN_POINT ( 'NONE',  ( 18.49999999999999645, 0.000000000000000000, -33.50000000000000000 ) ) ;
#113552=EDGE_CURVE ( 'NONE', #117400, #172386, #154699, .T. ) ;
#113558=CARTESIAN_POINT ( 'NONE',  ( -20.64999999999999858, -9.500000000000001776, -23.60603087734756045 ) ) ;
#113567=CARTESIAN_POINT ( 'NONE',  ( 21.11927991906888025, 6.448493118491415821, 0.009083679473894629153 ) ) ;
#113569=CARTESIAN_POINT ( 'NONE',  ( -23.15000000000000213, 1.999999999999998224, -20.27537807723789953 ) ) ;
#113573=VERTEX_POINT ( 'NONE', #242406 ) ;
#113590=CIRCLE ( 'NONE', #255176, 0.09999999999999939493 ) ;
#113602=CARTESIAN_POINT ( 'NONE',  ( 18.49999999999998934, 11.65000000000000391, -24.75000000000000000 ) ) ;
#113638=EDGE_CURVE ( 'NONE', #33602, #144336, #254608, .T. ) ;
#113663=ORIENTED_EDGE ( 'NONE', *, *, #8531, .F. ) ;
#113681=EDGE_CURVE ( 'NONE', #90989, #71337, #123764, .T. ) ;
#113692=VERTEX_POINT ( 'NONE', #144583 ) ;
#113697=EDGE_CURVE ( 'NONE', #32374, #138502, #38171, .T. ) ;
#113704=DIRECTION ( 'NONE',  ( 1.000000000000000000, 0.000000000000000000, 0.000000000000000000 ) ) ;
#113712=ORIENTED_EDGE ( 'NONE', *, *, #174940, .T. ) ;
#113723=VERTEX_POINT ( 'NONE', #27263 ) ;
#113729=ORIENTED_EDGE ( 'NONE', *, *, #58529, .F. ) ;
#113735=DIRECTION ( 'NONE',  ( 0.000000000000000000, 0.2605042016806672911, -0.9654727137038716656 ) ) ;
#113744=DIRECTION ( 'NONE',  ( 0.000000000000000000, -1.000000000000000000, 0.000000000000000000 ) ) ;
#113756=ADVANCED_FACE ( 'NONE', ( #106742 ), #7673, .F. ) ;
#113787=DIRECTION ( 'NONE',  ( 0.000000000000000000, -0.000000000000000000, 1.000000000000000000 ) ) ;
#113815=DIRECTION ( 'NONE',  ( 1.000000000000000000, 0.000000000000000000, -0.000000000000000000 ) ) ;
#113866=ORIENTED_EDGE ( 'NONE', *, *, #19944, .T. ) ;
#113876=VECTOR ( 'NONE', #96619, 1000.000000000000000 ) ;
#113896=ORIENTED_EDGE ( 'NONE', *, *, #150988, .T. ) ;
#113900=FACE_OUTER_BOUND ( 'NONE', #40905, .T. ) ;
#113905=DIRECTION ( 'NONE',  ( 0.000000000000000000, 0.000000000000000000, -1.000000000000000000 ) ) ;
#113914=VECTOR ( 'NONE', #44611, 1000.000000000000000 ) ;
#113934=ORIENTED_EDGE ( 'NONE', *, *, #117126, .T. ) ;
#113984=EDGE_CURVE ( 'NONE', #5236, #133804, #150755, .T. ) ;
#113989=ORIENTED_EDGE ( 'NONE', *, *, #139811, .F. ) ;
#114024=VECTOR ( 'NONE', #147456, 1000.000000000000000 ) ;
#114063=DIRECTION ( 'NONE',  ( 0.7071359030027766224, 0.000000000000000000, -0.7070776581709024011 ) ) ;
#114148=CARTESIAN_POINT ( 'NONE',  ( -20.64999999999999858, -9.000000000000001776, -23.60603087734756045 ) ) ;
#114190=EDGE_CURVE ( 'NONE', #145748, #230477, #142277, .T. ) ;
#114205=DIRECTION ( 'NONE',  ( 0.000000000000000000, -1.000000000000000000, 0.000000000000000000 ) ) ;
#114217=ORIENTED_EDGE ( 'NONE', *, *, #53766, .F. ) ;
#114230=AXIS2_PLACEMENT_3D ( 'NONE', #174343, #97273, #176880 ) ;
#114242=ORIENTED_EDGE ( 'NONE', *, *, #256521, .F. ) ;
#114279=CARTESIAN_POINT ( 'NONE',  ( -21.05000000000000071, -1.835341550224411922, -11.65515129256297833 ) ) ;
#114280=CARTESIAN_POINT ( 'NONE',  ( -21.05000000000000071, -11.41227409414968719, -3.000000000000002665 ) ) ;
#114284=VERTEX_POINT ( 'NONE', #8637 ) ;
#114299=( GEOMETRIC_REPRESENTATION_CONTEXT ( 3 ) GLOBAL_UNCERTAINTY_ASSIGNED_CONTEXT ( ( #191203 ) ) GLOBAL_UNIT_ASSIGNED_CONTEXT ( ( #133583, #174043, #171470 ) ) REPRESENTATION_CONTEXT ( 'NONE', 'WORKASPACE' ) );
#114309=DIRECTION ( 'NONE',  ( -1.000000000000000000, -0.000000000000000000, 0.000000000000000000 ) ) ;
#114322=CIRCLE ( 'NONE', #26869, 2.100000000000004530 ) ;
#114405=CARTESIAN_POINT ( 'NONE',  ( -21.05000000000000071, 1.835341550224411922, -11.65515129256298010 ) ) ;
#114417=FACE_OUTER_BOUND ( 'NONE', #119384, .T. ) ;
#114447=EDGE_CURVE ( 'NONE', #86957, #255533, #46872, .T. ) ;
#114461=PLANE ( 'NONE',  #241174 ) ;
#114485=ORIENTED_EDGE ( 'NONE', *, *, #211233, .T. ) ;
#114516=DIRECTION ( 'NONE',  ( -1.000000000000000000, -2.952720810173289112E-16, 0.000000000000000000 ) ) ;
#114530=LINE ( 'NONE', #91111, #206827 ) ;
#114538=CARTESIAN_POINT ( 'NONE',  ( 18.43579564894469769, -9.519327535292646303, -6.972976643860169688 ) ) ;
#114576=CARTESIAN_POINT ( 'NONE',  ( -20.94999999999999929, 1.835341550224413698, -11.55515129256298401 ) ) ;
#114579=DIRECTION ( 'NONE',  ( -0.000000000000000000, -0.000000000000000000, 1.000000000000000000 ) ) ;
#114602=EDGE_CURVE ( 'NONE', #150108, #15934, #234837, .T. ) ;
#114629=ADVANCED_FACE ( 'NONE', ( #52320 ), #176168, .F. ) ;
#114642=DIRECTION ( 'NONE',  ( 0.000000000000000000, -0.000000000000000000, -1.000000000000000000 ) ) ;
#114651=ORIENTED_EDGE ( 'NONE', *, *, #233988, .T. ) ;
#114652=ORIENTED_EDGE ( 'NONE', *, *, #123182, .T. ) ;
#114668=AXIS2_PLACEMENT_3D ( 'NONE', #186479, #66531, #126495 ) ;
#114726=CARTESIAN_POINT ( 'NONE',  ( -21.65000000000000213, 7.708578643762696636, -21.15000000000000213 ) ) ;
#114732=CYLINDRICAL_SURFACE ( 'NONE', #25808, 0.5000000000000004441 ) ;
#114757=CARTESIAN_POINT ( 'NONE',  ( 18.49999999999999289, 10.23906162412143672, -24.75439743459708808 ) ) ;
#114759=TOROIDAL_SURFACE ( 'NONE', #85482, 11.90000000000000391, 0.1000000000000000056 ) ;
#114788=DIRECTION ( 'NONE',  ( 0.000000000000000000, -1.000000000000000000, 0.000000000000000000 ) ) ;
#114791=DIRECTION ( 'NONE',  ( 0.000000000000000000, 0.4999999999999929501, 0.8660254037844427044 ) ) ;
#114795=ORIENTED_EDGE ( 'NONE', *, *, #69913, .F. ) ;
#114805=FACE_OUTER_BOUND ( 'NONE', #249747, .T. ) ;
#114849=CARTESIAN_POINT ( 'NONE',  ( 21.07971444708685738, 6.329792081626547606, 0.08782343631790544281 ) ) ;
#114874=EDGE_LOOP ( 'NONE', ( #143495, #48253, #248727, #157832 ) ) ;
#114892=CARTESIAN_POINT ( 'NONE',  ( 20.95420533658165141, 10.54586447475957733, -7.567506020693237190 ) ) ;
#114910=VECTOR ( 'NONE', #64085, 1000.000000000000000 ) ;
#114935=VECTOR ( 'NONE', #198913, 1000.000000000000000 ) ;
#114946=ORIENTED_EDGE ( 'NONE', *, *, #111020, .F. ) ;
#114972=VECTOR ( 'NONE', #166678, 1000.000000000000000 ) ;
#114982=CARTESIAN_POINT ( 'NONE',  ( 21.14999999999999858, -0.09999999999999939493, 11.64957080754479968 ) ) ;
#114998=TOROIDAL_SURFACE ( 'NONE', #98200, 0.2000000000000000111, 0.1000000000000000056 ) ;
#115033=ADVANCED_FACE ( 'NONE', ( #211113 ), #35083, .T. ) ;
#115043=AXIS2_PLACEMENT_3D ( 'NONE', #107708, #167717, #244646 ) ;
#115070=DIRECTION ( 'NONE',  ( 1.000000000000000000, 2.952720810173289112E-16, -0.000000000000000000 ) ) ;
#115085=ORIENTED_EDGE ( 'NONE', *, *, #150159, .T. ) ;
#115124=CARTESIAN_POINT ( 'NONE',  ( -18.47690164073607022, -9.464844538012236796, -40.20138093983610617 ) ) ;
#115169=ORIENTED_EDGE ( 'NONE', *, *, #147130, .F. ) ;
#115182=ORIENTED_EDGE ( 'NONE', *, *, #129606, .T. ) ;
#115218=VERTEX_POINT ( 'NONE', #66150 ) ;
#115229=EDGE_LOOP ( 'NONE', ( #41339, #182814, #148099, #17157 ) ) ;
#115301=ORIENTED_EDGE ( 'NONE', *, *, #196082, .F. ) ;
#115305=EDGE_LOOP ( 'NONE', ( #166512, #210868, #211093, #193604 ) ) ;
#115310=ADVANCED_FACE ( 'NONE', ( #196054 ), #225897, .T. ) ;
#115317=ORIENTED_EDGE ( 'NONE', *, *, #33819, .F. ) ;
#115320=CARTESIAN_POINT ( 'NONE',  ( -18.59999999999999787, -9.321008403361290107, -7.235938249077882745 ) ) ;
#115331=VECTOR ( 'NONE', #52327, 1000.000000000000000 ) ;
#115356=DIRECTION ( 'NONE',  ( 1.000000000000000000, 0.000000000000000000, 0.000000000000000000 ) ) ;
#115365=DIRECTION ( 'NONE',  ( -1.000000000000000000, 0.000000000000000000, 0.000000000000000000 ) ) ;
#115388=AXIS2_PLACEMENT_3D ( 'NONE', #201763, #43982, #23165 ) ;
#115397=CARTESIAN_POINT ( 'NONE',  ( 18.59999999999999432, -1.835859311443637010, -45.00443916879852679 ) ) ;
#115401=CARTESIAN_POINT ( 'NONE',  ( 18.52928932188133970, 10.27928932188134326, -24.70857864376268509 ) ) ;
#115402=CARTESIAN_POINT ( 'NONE',  ( -18.59999999999999787, -1.835859311443640340, -45.00443916879852679 ) ) ;
#115492=ORIENTED_EDGE ( 'NONE', *, *, #189408, .T. ) ;
#115495=DIRECTION ( 'NONE',  ( 0.000000000000000000, 0.000000000000000000, -1.000000000000000000 ) ) ;
#115517=ORIENTED_EDGE ( 'NONE', *, *, #110289, .T. ) ;
#115536=CARTESIAN_POINT ( 'NONE',  ( 21.05000000000000071, 0.000000000000000000, -35.40000000000000568 ) ) ;
#115539=CARTESIAN_POINT ( 'NONE',  ( -20.64999999999999858, -8.663551401869161950, -9.524101118067305194 ) ) ;
#115547=CARTESIAN_POINT ( 'NONE',  ( 21.05000000000000071, 11.75000000000000711, -26.48519422934605316 ) ) ;
#115584=EDGE_LOOP ( 'NONE', ( #164346, #255445, #40242, #26782 ) ) ;
#115593=AXIS2_PLACEMENT_3D ( 'NONE', #252683, #156197, #195323 ) ;
#115627=ORIENTED_EDGE ( 'NONE', *, *, #166267, .F. ) ;
#115634=ORIENTED_EDGE ( 'NONE', *, *, #215535, .T. ) ;
#115654=CARTESIAN_POINT ( 'NONE',  ( 21.05000000000000071, 8.926614585087097709, -8.471683019223119615 ) ) ;
#115657=FACE_OUTER_BOUND ( 'NONE', #183577, .T. ) ;
#115689=DIRECTION ( 'NONE',  ( 0.000000000000000000, -0.1568667991644693838, -0.9876197685951279004 ) ) ;
#115720=DIRECTION ( 'NONE',  ( 1.000000000000000000, 0.000000000000000000, -0.000000000000000000 ) ) ;
#115741=EDGE_LOOP ( 'NONE', ( #40016, #131962, #200294, #153308 ) ) ;
#115768=ORIENTED_EDGE ( 'NONE', *, *, #14037, .F. ) ;
#115770=AXIS2_PLACEMENT_3D ( 'NONE', #144309, #103904, #179638 ) ;
#115776=DIRECTION ( 'NONE',  ( 1.000000000000000000, 0.000000000000000000, 0.000000000000000000 ) ) ;
#115779=ORIENTED_EDGE ( 'NONE', *, *, #38106, .T. ) ;
#115786=AXIS2_PLACEMENT_3D ( 'NONE', #123461, #139136, #162596 ) ;
#115790=AXIS2_PLACEMENT_3D ( 'NONE', #95385, #70717, #94088 ) ;
#115804=EDGE_CURVE ( 'NONE', #166638, #172600, #176085, .T. ) ;
#115810=CARTESIAN_POINT ( 'NONE',  ( -21.05000000000000426, 6.477046381789849150, -0.09999999999999885369 ) ) ;
#115817=AXIS2_PLACEMENT_3D ( 'NONE', #257106, #135909, #138468 ) ;
#115832=CARTESIAN_POINT ( 'NONE',  ( 18.49362639424895605, -9.442604367888192129, -40.26444093351152276 ) ) ;
#115868=LINE ( 'NONE', #172031, #59986 ) ;
#115872=EDGE_CURVE ( 'NONE', #57548, #202111, #2661, .T. ) ;
#115873=CARTESIAN_POINT ( 'NONE',  ( 18.59999999999999787, -1.263275465217258198, -41.40186466674640542 ) ) ;
#115904=ORIENTED_EDGE ( 'NONE', *, *, #118288, .F. ) ;
#115905=EDGE_CURVE ( 'NONE', #19688, #167418, #82154, .T. ) ;
#115921=VERTEX_POINT ( 'NONE', #190312 ) ;
#116004=CARTESIAN_POINT ( 'NONE',  ( 20.44999100639894962, 10.43971070321203953, -7.759075725970426163 ) ) ;
#116021=DIRECTION ( 'NONE',  ( 0.000000000000000000, 0.000000000000000000, -1.000000000000000000 ) ) ;
#116024=FACE_OUTER_BOUND ( 'NONE', #70359, .T. ) ;
#116056=CARTESIAN_POINT ( 'NONE',  ( 18.49999999999999289, 10.20857864376268864, -24.65000000000000213 ) ) ;
#116070=VERTEX_POINT ( 'NONE', #16814 ) ;
#116138=FACE_OUTER_BOUND ( 'NONE', #192880, .T. ) ;
#116140=DIRECTION ( 'NONE',  ( 0.000000000000000000, 1.265107689135680095E-16, -1.000000000000000000 ) ) ;
#116148=LINE ( 'NONE', #14495, #56668 ) ;
#116166=CIRCLE ( 'NONE', #16212, 7.800000000000001599 ) ;
#116171=CARTESIAN_POINT ( 'NONE',  ( 20.12500000000000000, 9.749999999999998224, -8.111771282114276005 ) ) ;
#116176=FACE_OUTER_BOUND ( 'NONE', #121916, .T. ) ;
#116190=CARTESIAN_POINT ( 'NONE',  ( -20.54999999999999716, 4.349999999999999645, -12.35000000000000142 ) ) ;
#116201=ORIENTED_EDGE ( 'NONE', *, *, #78697, .F. ) ;
#116248=DIRECTION ( 'NONE',  ( -1.000000000000000000, -2.952720810173289112E-16, 0.000000000000000000 ) ) ;
#116251=ORIENTED_EDGE ( 'NONE', *, *, #74938, .F. ) ;
#116270=EDGE_CURVE ( 'NONE', #185056, #210716, #165289, .T. ) ;
#116295=VECTOR ( 'NONE', #46519, 1000.000000000000114 ) ;
#116325=DIRECTION ( 'NONE',  ( -1.000000000000000000, 0.000000000000000000, 0.000000000000000000 ) ) ;
#116335=DIRECTION ( 'NONE',  ( 0.000000000000000000, 0.000000000000000000, -1.000000000000000000 ) ) ;
#116358=CARTESIAN_POINT ( 'NONE',  ( -21.05000000000000071, 0.000000000000000000, 0.000000000000000000 ) ) ;
#116365=AXIS2_PLACEMENT_3D ( 'NONE', #49248, #229184, #11423 ) ;
#116398=CARTESIAN_POINT ( 'NONE',  ( 22.48660254037844197, 11.65000000000000036, 0.04999999999999833050 ) ) ;
#116404=DIRECTION ( 'NONE',  ( 0.000000000000000000, 0.000000000000000000, -1.000000000000000000 ) ) ;
#116455=CIRCLE ( 'NONE', #4007, 0.4000000000000010214 ) ;
#116475=DIRECTION ( 'NONE',  ( 0.000000000000000000, 0.000000000000000000, -1.000000000000000000 ) ) ;
#116486=CARTESIAN_POINT ( 'NONE',  ( 22.39999999999999503, 11.75000000000000711, 0.09999999999999592548 ) ) ;
#116495=AXIS2_PLACEMENT_3D ( 'NONE', #111164, #152893, #90292 ) ;
#116517=EDGE_CURVE ( 'NONE', #34317, #163039, #134705, .T. ) ;
#116551=DIRECTION ( 'NONE',  ( 0.000000000000000000, 0.000000000000000000, 1.000000000000000000 ) ) ;
#116565=EDGE_CURVE ( 'NONE', #112246, #8515, #176867, .T. ) ;
#116587=ADVANCED_FACE ( 'NONE', ( #198969 ), #98541, .F. ) ;
#116597=CIRCLE ( 'NONE', #29167, 0.5000000000000004441 ) ;
#116600=EDGE_LOOP ( 'NONE', ( #4898, #237673, #99907 ) ) ;
#116616=VECTOR ( 'NONE', #180442, 1000.000000000000000 ) ;
#116618=DIRECTION ( 'NONE',  ( 1.000000000000000000, 0.000000000000000000, 0.000000000000000000 ) ) ;
#116651=CARTESIAN_POINT ( 'NONE',  ( -22.50485643085239928, -0.07878633907718655960, 11.74979493917241413 ) ) ;
#116659=CARTESIAN_POINT ( 'NONE',  ( 21.05000000000000071, 0.000000000000000000, -12.97499999999999787 ) ) ;
#116669=CARTESIAN_POINT ( 'NONE',  ( 23.15000000000000213, -11.39257802170566691, -30.42605042016806394 ) ) ;
#116685=CARTESIAN_POINT ( 'NONE',  ( 18.59999999999999076, 10.49142135623730709, -24.75000000000000000 ) ) ;
#116691=CARTESIAN_POINT ( 'NONE',  ( -23.15000000000000213, 4.349999999999999645, -12.35000000000000142 ) ) ;
#116731=CARTESIAN_POINT ( 'NONE',  ( -20.94999999999999929, -11.48912529307605901, -3.000000000000002665 ) ) ;
#116740=DIRECTION ( 'NONE',  ( -1.000000000000000000, -0.000000000000000000, -0.000000000000000000 ) ) ;
#116746=CYLINDRICAL_SURFACE ( 'NONE', #183704, 0.1000000000000028644 ) ;
#116759=EDGE_CURVE ( 'NONE', #191070, #248248, #243042, .T. ) ;
#116788=EDGE_CURVE ( 'NONE', #163200, #212474, #71041, .T. ) ;
#116805=ADVANCED_FACE ( 'NONE', ( #174017 ), #112717, .F. ) ;
#116812=DIRECTION ( 'NONE',  ( 1.000000000000000000, 0.000000000000000000, 0.000000000000000000 ) ) ;
#116866=CIRCLE ( 'NONE', #141796, 0.1000000000000002554 ) ;
#116869=DIRECTION ( 'NONE',  ( 1.000000000000000000, 0.000000000000000000, -0.000000000000000000 ) ) ;
#116888=VECTOR ( 'NONE', #136833, 1000.000000000000000 ) ;
#116901=CARTESIAN_POINT ( 'NONE',  ( -18.39999999999999858, -9.600000000000004974, -40.10018939122204529 ) ) ;
#116906=VERTEX_POINT ( 'NONE', #133556 ) ;
#116908=CARTESIAN_POINT ( 'NONE',  ( -18.60000000000001208, -9.364240527590910190, -7.180248581840769972 ) ) ;
#116942=DIRECTION ( 'NONE',  ( -1.000000000000000000, -2.952720810173289112E-16, 0.000000000000000000 ) ) ;
#116998=CARTESIAN_POINT ( 'NONE',  ( 21.13461538461538680, 10.61458296202553875, -12.25000000000000000 ) ) ;
#117003=DIRECTION ( 'NONE',  ( 1.000000000000000000, 3.265361837132813093E-16, -0.000000000000000000 ) ) ;
#117014=DIRECTION ( 'NONE',  ( 0.000000000000000000, 0.000000000000000000, -1.000000000000000000 ) ) ;
#117015=B_SPLINE_CURVE_WITH_KNOTS ( 'NONE', 3,
 ( #132682, #127540, #148392, #28483, #227924, #212230, #31044, #190084, #208381, #10166, #33624, #89676, #107979, #169273, #248780, #70161 ),
 .UNSPECIFIED., .F., .F.,
 ( 4, 3, 3, 3, 3, 4 ),
 ( 0.000000000000000000, 2.372700795693896277E-05, 5.739057815866941569E-05, 9.073899019179925297E-05, 0.0001243544287365695982, 0.0001585386695601168831 ),
 .UNSPECIFIED. ) ;
#117029=DIRECTION ( 'NONE',  ( 0.000000000000000000, 0.000000000000000000, -1.000000000000000000 ) ) ;
#117036=AXIS2_PLACEMENT_3D ( 'NONE', #253582, #55353, #134900 ) ;
#117039=EDGE_CURVE ( 'NONE', #237441, #161574, #45691, .T. ) ;
#117089=FACE_OUTER_BOUND ( 'NONE', #217228, .T. ) ;
#117101=VERTEX_POINT ( 'NONE', #130352 ) ;
#117126=EDGE_CURVE ( 'NONE', #214000, #52139, #97457, .T. ) ;
#117127=CARTESIAN_POINT ( 'NONE',  ( 23.14999999999999503, 6.649999999999999467, -21.15000000000000213 ) ) ;
#117179=DIRECTION ( 'NONE',  ( -1.000000000000000000, 0.000000000000000000, 0.000000000000000000 ) ) ;
#117182=ORIENTED_EDGE ( 'NONE', *, *, #143549, .F. ) ;
#117199=DIRECTION ( 'NONE',  ( -1.000000000000000000, 0.000000000000000000, 0.000000000000000000 ) ) ;
#117216=CARTESIAN_POINT ( 'NONE',  ( -23.25000000000000000, 0.000000000000000000, -33.50000000000000000 ) ) ;
#117240=EDGE_CURVE ( 'NONE', #156138, #28028, #187790, .T. ) ;
#117256=DIRECTION ( 'NONE',  ( -2.602085213965226419E-14, -0.000000000000000000, 1.000000000000000000 ) ) ;
#117260=ADVANCED_FACE ( 'NONE', ( #89944 ), #139342, .T. ) ;
#117276=ADVANCED_FACE ( 'NONE', ( #53396 ), #216309, .T. ) ;
#117283=EDGE_LOOP ( 'NONE', ( #40039, #169700, #69244, #222197 ) ) ;
#117300=PLANE ( 'NONE',  #150053 ) ;
#117302=CARTESIAN_POINT ( 'NONE',  ( -22.39999999999999858, 0.000000000000000000, 11.64957080754479968 ) ) ;
#117315=DIRECTION ( 'NONE',  ( 1.000000000000000000, 0.000000000000000000, 0.000000000000000000 ) ) ;
#117327=VERTEX_POINT ( 'NONE', #172104 ) ;
#117338=EDGE_CURVE ( 'NONE', #112707, #138031, #86677, .T. ) ;
#117353=CARTESIAN_POINT ( 'NONE',  ( 23.14999999999999503, 6.649999999999999467, -21.15000000000000213 ) ) ;
#117366=ORIENTED_EDGE ( 'NONE', *, *, #15082, .T. ) ;
#117382=EDGE_LOOP ( 'NONE', ( #152733, #123359, #115768, #78348 ) ) ;
#117398=DIRECTION ( 'NONE',  ( 0.000000000000000000, 1.224646799147316229E-16, 1.000000000000000000 ) ) ;
#117400=VERTEX_POINT ( 'NONE', #243583 ) ;
#117415=ADVANCED_FACE ( 'NONE', ( #1094 ), #81085, .F. ) ;
#117423=CARTESIAN_POINT ( 'NONE',  ( 21.08035267497491105, 6.331706839783013407, 0.08268862477613450612 ) ) ;
#117436=FACE_OUTER_BOUND ( 'NONE', #217604, .T. ) ;
#117461=ADVANCED_FACE ( 'NONE', ( #147033 ), #247696, .T. ) ;
#117528=DIRECTION ( 'NONE',  ( -6.938893903907222067E-15, 1.000000000000000000, 0.000000000000000000 ) ) ;
#117566=VERTEX_POINT ( 'NONE', #224009 ) ;
#117607=DIRECTION ( 'NONE',  ( 1.000000000000000000, 0.000000000000000000, 0.000000000000000000 ) ) ;
#117624=AXIS2_PLACEMENT_3D ( 'NONE', #24314, #106373, #185931 ) ;
#117635=CARTESIAN_POINT ( 'NONE',  ( -21.59142135623730852, 7.850000000000003197, -12.34999999999999964 ) ) ;
#117645=AXIS2_PLACEMENT_3D ( 'NONE', #57274, #175990, #216366 ) ;
#117666=ORIENTED_EDGE ( 'NONE', *, *, #154513, .F. ) ;
#117697=DIRECTION ( 'NONE',  ( 1.000000000000000000, -0.000000000000000000, 0.000000000000000000 ) ) ;
#117698=AXIS2_PLACEMENT_3D ( 'NONE', #84387, #221365, #64873 ) ;
#117739=TOROIDAL_SURFACE ( 'NONE', #42723, 12.97499999999999787, 0.1000000000000000056 ) ;
#117749=CIRCLE ( 'NONE', #230171, 12.87499999999999822 ) ;
#117778=ORIENTED_EDGE ( 'NONE', *, *, #174858, .F. ) ;
#117791=EDGE_LOOP ( 'NONE', ( #51396, #39295, #11696, #192131 ) ) ;
#117801=VECTOR ( 'NONE', #56177, 1000.000000000000000 ) ;
#117832=LINE ( 'NONE', #240366, #27394 ) ;
#117846=CARTESIAN_POINT ( 'NONE',  ( 20.12500000000000000, 9.749999999999998224, -8.111771282114276005 ) ) ;
#117866=CIRCLE ( 'NONE', #205336, 4.149999999999999467 ) ;
#117875=CYLINDRICAL_SURFACE ( 'NONE', #34554, 0.09999999999999939493 ) ;
#117885=CARTESIAN_POINT ( 'NONE',  ( 21.12769345151713196, 10.71928767694057072, -12.24748034619748616 ) ) ;
#117901=DIRECTION ( 'NONE',  ( 2.659396599871503635E-15, 0.6132151058540549204, -0.7899159663865520375 ) ) ;
#117905=AXIS2_PLACEMENT_3D ( 'NONE', #17951, #69290, #208793 ) ;
#117931=DIRECTION ( 'NONE',  ( 0.000000000000000000, 1.000000000000000000, 0.000000000000000000 ) ) ;
#117945=AXIS2_PLACEMENT_3D ( 'NONE', #170418, #229064, #253732 ) ;
#117963=AXIS2_PLACEMENT_3D ( 'NONE', #212311, #47102, #206203 ) ;
#117974=DIRECTION ( 'NONE',  ( 0.000000000000000000, 0.000000000000000000, -1.000000000000000000 ) ) ;
#117989=CIRCLE ( 'NONE', #126365, 7.900000000000000355 ) ;
#118008=CARTESIAN_POINT ( 'NONE',  ( -18.48179518609178018, -9.518325300493765795, -40.38970557676145745 ) ) ;
#118026=AXIS2_PLACEMENT_3D ( 'NONE', #113529, #232219, #39150 ) ;
#118030=LINE ( 'NONE', #157189, #233584 ) ;
#118056=DIRECTION ( 'NONE',  ( -0.000000000000000000, 0.7397360091702694929, 0.6728971962616898672 ) ) ;
#118058=ORIENTED_EDGE ( 'NONE', *, *, #249892, .T. ) ;
#118083=ORIENTED_EDGE ( 'NONE', *, *, #129217, .F. ) ;
#118086=EDGE_LOOP ( 'NONE', ( #16981, #245750, #197671, #125862 ) ) ;
#118094=EDGE_CURVE ( 'NONE', #210716, #204739, #245419, .T. ) ;
#118129=ORIENTED_EDGE ( 'NONE', *, *, #12690, .F. ) ;
#118176=CARTESIAN_POINT ( 'NONE',  ( -21.07928932188134041, 0.000000000000000000, 0.000000000000000000 ) ) ;
#118182=CARTESIAN_POINT ( 'NONE',  ( 20.95159278453404283, 8.907896337949049226, -8.484720185109249968 ) ) ;
#118209=ORIENTED_EDGE ( 'NONE', *, *, #162551, .F. ) ;
#118288=EDGE_CURVE ( 'NONE', #209903, #119379, #138060, .T. ) ;
#118291=ORIENTED_EDGE ( 'NONE', *, *, #177525, .T. ) ;
#118312=VECTOR ( 'NONE', #95941, 1000.000000000000000 ) ;
#118335=CARTESIAN_POINT ( 'NONE',  ( 18.60000000000000142, -9.321008403361283001, -7.235938249077890738 ) ) ;
#118438=DIRECTION ( 'NONE',  ( -1.000000000000000000, 0.000000000000000000, 0.000000000000000000 ) ) ;
#118441=ADVANCED_FACE ( 'NONE', ( #231422 ), #28098, .F. ) ;
#118482=CARTESIAN_POINT ( 'NONE',  ( -21.14999999999999858, 0.000000000000000000, 6.540656951701240729 ) ) ;
#118500=EDGE_LOOP ( 'NONE', ( #33892, #84849, #143886, #210228 ) ) ;
#118510=DIRECTION ( 'NONE',  ( 0.000000000000000000, 0.000000000000000000, -1.000000000000000000 ) ) ;
#118517=DIRECTION ( 'NONE',  ( 1.000000000000000000, 0.000000000000000000, -0.000000000000000000 ) ) ;
#118520=ORIENTED_EDGE ( 'NONE', *, *, #214235, .F. ) ;
#118521=ORIENTED_EDGE ( 'NONE', *, *, #251111, .F. ) ;
#118536=DIRECTION ( 'NONE',  ( 1.000000000000000000, -0.000000000000000000, -0.000000000000000000 ) ) ;
#118573=CARTESIAN_POINT ( 'NONE',  ( 20.59588692710267921, 10.36872342116900292, -7.639081094510505210 ) ) ;
#118589=CARTESIAN_POINT ( 'NONE',  ( 18.49999999999999645, -1.362429037193310988, -41.38888124792119783 ) ) ;
#118595=ORIENTED_EDGE ( 'NONE', *, *, #198695, .F. ) ;
#118599=LINE ( 'NONE', #159021, #13348 ) ;
#118600=DIRECTION ( 'NONE',  ( 1.000000000000000000, 0.000000000000000000, 0.000000000000000000 ) ) ;
#118617=CARTESIAN_POINT ( 'NONE',  ( 23.24999999999999645, 4.775700934579428569, -11.84876810404597158 ) ) ;
#118630=VECTOR ( 'NONE', #144617, 1000.000000000000227 ) ;
#118638=DIRECTION ( 'NONE',  ( -1.000000000000000000, 0.000000000000000000, 0.000000000000000000 ) ) ;
#118639=ORIENTED_EDGE ( 'NONE', *, *, #75821, .F. ) ;
#118653=ORIENTED_EDGE ( 'NONE', *, *, #34998, .T. ) ;
#118672=CARTESIAN_POINT ( 'NONE',  ( -18.59999999999999787, -1.736257131597395809, -11.56865232901749785 ) ) ;
#118684=DIRECTION ( 'NONE',  ( -1.000000000000000000, -2.952720810173289112E-16, 0.000000000000000000 ) ) ;
#118702=DIRECTION ( 'NONE',  ( 0.000000000000000000, 0.000000000000000000, 1.000000000000000000 ) ) ;
#118713=DIRECTION ( 'NONE',  ( 0.000000000000000000, 0.000000000000000000, -1.000000000000000000 ) ) ;
#118727=CIRCLE ( 'NONE', #164511, 12.77499999999999858 ) ;
#118787=EDGE_LOOP ( 'NONE', ( #139841, #11032, #106607, #8587 ) ) ;
#118795=VERTEX_POINT ( 'NONE', #42203 ) ;
#118796=DIRECTION ( 'NONE',  ( 0.000000000000000000, 0.000000000000000000, -1.000000000000000000 ) ) ;
#118821=ADVANCED_FACE ( 'NONE', ( #70780 ), #70824, .T. ) ;
#118824=ORIENTED_EDGE ( 'NONE', *, *, #211954, .F. ) ;
#118849=EDGE_LOOP ( 'NONE', ( #193103, #179976, #174298, #1041 ) ) ;
#118924=ORIENTED_EDGE ( 'NONE', *, *, #216186, .T. ) ;
#118950=DIRECTION ( 'NONE',  ( 1.000000000000000000, 0.000000000000000000, 0.000000000000000000 ) ) ;
#118989=AXIS2_PLACEMENT_3D ( 'NONE', #107909, #130021, #247414 ) ;
#119037=CIRCLE ( 'NONE', #214680, 0.09999999999999939493 ) ;
#119050=FACE_OUTER_BOUND ( 'NONE', #157300, .T. ) ;
#119067=CARTESIAN_POINT ( 'NONE',  ( 23.14999999999999858, 4.813084112149524252, -11.94151775652382419 ) ) ;
#119143=ADVANCED_FACE ( 'NONE', ( #223091 ), #186497, .T. ) ;
#119149=DIRECTION ( 'NONE',  ( -1.000000000000000000, -0.000000000000000000, -0.000000000000000000 ) ) ;
#119178=DIRECTION ( 'NONE',  ( 0.000000000000000000, 0.000000000000000000, -1.000000000000000000 ) ) ;
#119223=DIRECTION ( 'NONE',  ( 0.000000000000000000, 0.000000000000000000, -1.000000000000000000 ) ) ;
#119226=CARTESIAN_POINT ( 'NONE',  ( -20.94999999999999929, -1.162701749938009677, -8.099999999999999645 ) ) ;
#119236=CIRCLE ( 'NONE', #202612, 0.09999999999999999167 ) ;
#119255=EDGE_CURVE ( 'NONE', #255303, #90335, #172162, .T. ) ;
#119279=FACE_OUTER_BOUND ( 'NONE', #171547, .T. ) ;
#119295=CARTESIAN_POINT ( 'NONE',  ( 18.49999999999999645, -1.162701749938011453, -8.099999999999999645 ) ) ;
#119315=VERTEX_POINT ( 'NONE', #175993 ) ;
#119330=FACE_OUTER_BOUND ( 'NONE', #202246, .T. ) ;
#119379=VERTEX_POINT ( 'NONE', #182401 ) ;
#119384=EDGE_LOOP ( 'NONE', ( #3423, #106499, #63943 ) ) ;
#119390=CARTESIAN_POINT ( 'NONE',  ( -20.54999999999999716, 0.000000000000000000, -20.62500000000000355 ) ) ;
#119400=EDGE_CURVE ( 'NONE', #40817, #120793, #254303, .T. ) ;
#119401=( BOUNDED_CURVE ( )  B_SPLINE_CURVE ( 3, ( #197501, #115401, #37174, #116685 ),
 .UNSPECIFIED., .F., .F. ) 
 B_SPLINE_CURVE_WITH_KNOTS ( ( 4, 4 ),
 ( 3.141592653589793116, 4.712388980384689674 ),
 .UNSPECIFIED. ) 
 CURVE ( )  GEOMETRIC_REPRESENTATION_ITEM ( )  RATIONAL_B_SPLINE_CURVE ( ( 1.000000000000000000, 0.8047378541243649375, 0.8047378541243649375, 1.000000000000000000 ) ) 
 REPRESENTATION_ITEM ( '' )  );
#119472=ORIENTED_EDGE ( 'NONE', *, *, #237805, .T. ) ;
#119475=DIRECTION ( 'NONE',  ( 1.000000000000000000, 0.000000000000000000, -0.000000000000000000 ) ) ;
#119532=EDGE_LOOP ( 'NONE', ( #218056, #198302, #87370, #188873, #184617 ) ) ;
#119533=EDGE_CURVE ( 'NONE', #214079, #177816, #89686, .T. ) ;
#119545=CARTESIAN_POINT ( 'NONE',  ( -21.44999999999999929, 7.249999999999999112, -21.25000000000000000 ) ) ;
#119547=CARTESIAN_POINT ( 'NONE',  ( -20.54999999999999716, -9.500000000000001776, -23.60603087734756045 ) ) ;
#119554=ORIENTED_EDGE ( 'NONE', *, *, #26423, .F. ) ;
#119558=ORIENTED_EDGE ( 'NONE', *, *, #131163, .F. ) ;
#119559=EDGE_CURVE ( 'NONE', #255460, #106654, #200337, .T. ) ;
#119567=ORIENTED_EDGE ( 'NONE', *, *, #142941, .T. ) ;
#119588=EDGE_CURVE ( 'NONE', #63488, #151938, #87876, .T. ) ;
#119590=AXIS2_PLACEMENT_3D ( 'NONE', #130945, #166251, #10994 ) ;
#119598=VECTOR ( 'NONE', #90012, 1000.000000000000000 ) ;
#119611=CYLINDRICAL_SURFACE ( 'NONE', #168059, 0.5000000000000022204 ) ;
#119631=CARTESIAN_POINT ( 'NONE',  ( 22.50000000000000000, 0.000000000000000000, 0.000000000000000000 ) ) ;
#119640=CARTESIAN_POINT ( 'NONE',  ( 21.05000000000000071, 6.477552182493491628, -0.09999996530010009377 ) ) ;
#119644=ORIENTED_EDGE ( 'NONE', *, *, #29137, .F. ) ;
#119645=CARTESIAN_POINT ( 'NONE',  ( -18.50000000000000000, 7.021664781900089913, -37.13356540189729316 ) ) ;
#119671=DIRECTION ( 'NONE',  ( -1.000000000000000000, -0.000000000000000000, -0.000000000000000000 ) ) ;
#119693=ORIENTED_EDGE ( 'NONE', *, *, #31781, .T. ) ;
#119695=EDGE_LOOP ( 'NONE', ( #102592, #50491, #25131, #18274 ) ) ;
#119704=ORIENTED_EDGE ( 'NONE', *, *, #142174, .F. ) ;
#119729=EDGE_CURVE ( 'NONE', #201752, #82580, #79515, .T. ) ;
#119731=ORIENTED_EDGE ( 'NONE', *, *, #106735, .F. ) ;
#119733=EDGE_CURVE ( 'NONE', #150376, #105026, #133697, .T. ) ;
#119741=LINE ( 'NONE', #237108, #250947 ) ;
#119746=CARTESIAN_POINT ( 'NONE',  ( 20.94999999999999574, 1.162701749938009677, -7.900000000000000355 ) ) ;
#119776=ORIENTED_EDGE ( 'NONE', *, *, #11284, .T. ) ;
#119802=DIRECTION ( 'NONE',  ( 0.000000000000000000, 0.000000000000000000, 1.000000000000000000 ) ) ;
#119820=DIRECTION ( 'NONE',  ( 1.000000000000000000, -0.000000000000000000, -0.000000000000000000 ) ) ;
#119829=VECTOR ( 'NONE', #133981, 1000.000000000000000 ) ;
#119863=FACE_OUTER_BOUND ( 'NONE', #82922, .T. ) ;
#119880=ORIENTED_EDGE ( 'NONE', *, *, #178612, .T. ) ;
#119891=CARTESIAN_POINT ( 'NONE',  ( -21.05000000000000071, -0.09999999999999939493, 6.540656951701240729 ) ) ;
#119898=DIRECTION ( 'NONE',  ( 0.000000000000000000, 0.000000000000000000, 1.000000000000000000 ) ) ;
#119909=ORIENTED_EDGE ( 'NONE', *, *, #252232, .T. ) ;
#119925=FACE_OUTER_BOUND ( 'NONE', #50439, .T. ) ;
#119979=EDGE_CURVE ( 'NONE', #228001, #166580, #149950, .T. ) ;
#119991=LINE ( 'NONE', #159108, #87042 ) ;
#119997=DIRECTION ( 'NONE',  ( -0.000000000000000000, 0.8660254037844411501, 0.4999999999999956701 ) ) ;
#120040=DIRECTION ( 'NONE',  ( 0.000000000000000000, 0.000000000000000000, -1.000000000000000000 ) ) ;
#120047=CIRCLE ( 'NONE', #7582, 0.09999999999999939493 ) ;
#120058=CARTESIAN_POINT ( 'NONE',  ( 20.94999999999999574, 10.47338541491290442, -7.578654464248542943 ) ) ;
#120093=EDGE_LOOP ( 'NONE', ( #81632, #171274, #90015, #59071 ) ) ;
#120094=ORIENTED_EDGE ( 'NONE', *, *, #113180, .T. ) ;
#120101=EDGE_CURVE ( 'NONE', #250243, #226600, #241428, .T. ) ;
#120111=ORIENTED_EDGE ( 'NONE', *, *, #135403, .T. ) ;
#120121=ORIENTED_EDGE ( 'NONE', *, *, #83477, .F. ) ;
#120149=CARTESIAN_POINT ( 'NONE',  ( 18.59999999999999432, -1.162701749938009677, -8.000000000000000000 ) ) ;
#120156=ORIENTED_EDGE ( 'NONE', *, *, #12566, .T. ) ;
#120159=CARTESIAN_POINT ( 'NONE',  ( -23.15000000000000213, 11.65000000000000036, -12.25000000000000000 ) ) ;
#120171=AXIS2_PLACEMENT_3D ( 'NONE', #101882, #181468, #202301 ) ;
#120209=LINE ( 'NONE', #159317, #224093 ) ;
#120224=DIRECTION ( 'NONE',  ( -1.000000000000000000, -0.000000000000000000, -0.000000000000000000 ) ) ;
#120273=ORIENTED_EDGE ( 'NONE', *, *, #50303, .F. ) ;
#120295=ORIENTED_EDGE ( 'NONE', *, *, #69756, .T. ) ;
#120301=CARTESIAN_POINT ( 'NONE',  ( -18.50000000000000000, -9.400000000000005684, -40.41465834296965909 ) ) ;
#120353=EDGE_CURVE ( 'NONE', #129511, #3044, #63313, .T. ) ;
#120405=VECTOR ( 'NONE', #41638, 1000.000000000000000 ) ;
#120448=VERTEX_POINT ( 'NONE', #58605 ) ;
#120463=DIRECTION ( 'NONE',  ( 0.000000000000000000, 1.000000000000000000, 0.000000000000000000 ) ) ;
#120465=CARTESIAN_POINT ( 'NONE',  ( 18.49999999999999289, 11.75000000000000355, 11.75000000000000000 ) ) ;
#120497=AXIS2_PLACEMENT_3D ( 'NONE', #147260, #44327, #106840 ) ;
#120525=CARTESIAN_POINT ( 'NONE',  ( -22.00411653889209518, 0.09903810578596834724, 7.253442867640404579 ) ) ;
#120531=CARTESIAN_POINT ( 'NONE',  ( 23.24999999999999645, 4.999999999999997335, -12.40526601891309788 ) ) ;
#120628=CARTESIAN_POINT ( 'NONE',  ( 21.05000000000000071, 5.849999999999949019, -10.13249722427797117 ) ) ;
#120640=VERTEX_POINT ( 'NONE', #130142 ) ;
#120652=CARTESIAN_POINT ( 'NONE',  ( 23.14999999999999858, 0.000000000000000000, -33.50000000000000000 ) ) ;
#120667=DIRECTION ( 'NONE',  ( 0.000000000000000000, 0.000000000000000000, -1.000000000000000000 ) ) ;
#120710=DIRECTION ( 'NONE',  ( 1.000000000000000000, 0.000000000000000000, 0.000000000000000000 ) ) ;
#120719=FACE_OUTER_BOUND ( 'NONE', #155332, .T. ) ;
#120739=EDGE_CURVE ( 'NONE', #148838, #93175, #58293, .T. ) ;
#120743=AXIS2_PLACEMENT_3D ( 'NONE', #13661, #174062, #73663 ) ;
#120793=VERTEX_POINT ( 'NONE', #33675 ) ;
#120807=CARTESIAN_POINT ( 'NONE',  ( 23.14999999999999858, -2.100000000000002309, -33.50000000000000000 ) ) ;
#120829=ORIENTED_EDGE ( 'NONE', *, *, #3999, .F. ) ;
#120845=DIRECTION ( 'NONE',  ( 1.000000000000000000, 0.000000000000000000, 0.000000000000000000 ) ) ;
#120873=DIRECTION ( 'NONE',  ( 0.000000000000000000, -0.8700118002898359348, 0.4930308989875165082 ) ) ;
#120942=EDGE_CURVE ( 'NONE', #226810, #79078, #221500, .T. ) ;
#120955=CARTESIAN_POINT ( 'NONE',  ( 21.05000000000000071, 0.03201369318779723888, 6.258842723537621389 ) ) ;
#121017=ORIENTED_EDGE ( 'NONE', *, *, #102570, .F. ) ;
#121019=DIRECTION ( 'NONE',  ( 2.827886303505249259E-16, -0.8660254037844411501, -0.4999999999999956701 ) ) ;
#121035=SPHERICAL_SURFACE ( 'NONE', #24450, 0.1000000000000000056 ) ;
#121057=DIRECTION ( 'NONE',  ( 1.000000000000000000, 0.000000000000000000, 0.000000000000000000 ) ) ;
#121094=ORIENTED_EDGE ( 'NONE', *, *, #227902, .F. ) ;
#121109=DIRECTION ( 'NONE',  ( 1.000000000000000000, -0.000000000000000000, -0.000000000000000000 ) ) ;
#121129=DIRECTION ( 'NONE',  ( 0.000000000000000000, 1.897661533703519897E-16, -1.000000000000000000 ) ) ;
#121152=DIRECTION ( 'NONE',  ( 0.000000000000000000, 0.000000000000000000, -1.000000000000000000 ) ) ;
#121156=CARTESIAN_POINT ( 'NONE',  ( 20.52683494730037239, 8.980530818301453166, -8.505252722537006704 ) ) ;
#121171=EDGE_CURVE ( 'NONE', #94374, #72992, #16337, .T. ) ;
#121198=AXIS2_PLACEMENT_3D ( 'NONE', #25790, #66206, #144423 ) ;
#121222=CARTESIAN_POINT ( 'NONE',  ( -22.39999999999999858, 11.65000000000000036, -0.1000000000000028644 ) ) ;
#121250=CARTESIAN_POINT ( 'NONE',  ( 21.00023020733438273, 6.390869245267715826, -6.911788849595090767E-16 ) ) ;
#121268=DIRECTION ( 'NONE',  ( 1.000000000000000000, 0.000000000000000000, 0.000000000000000000 ) ) ;
#121275=EDGE_LOOP ( 'NONE', ( #158392, #151551, #30967, #243332 ) ) ;
#121288=DIRECTION ( 'NONE',  ( 1.000000000000000000, 0.000000000000000000, 0.000000000000000000 ) ) ;
#121295=DIRECTION ( 'NONE',  ( 3.469446951953609771E-14, -0.7899159663865552572, -0.6132151058540507016 ) ) ;
#121316=EDGE_CURVE ( 'NONE', #152840, #40817, #176149, .T. ) ;
#121318=EDGE_LOOP ( 'NONE', ( #164880, #73287, #73516, #10352 ) ) ;
#121336=ORIENTED_EDGE ( 'NONE', *, *, #172116, .T. ) ;
#121344=CARTESIAN_POINT ( 'NONE',  ( 22.60000000000000142, 0.000000000000000000, 0.000000000000000000 ) ) ;
#121352=CARTESIAN_POINT ( 'NONE',  ( 21.59780538579342135, 0.09897866959798530540, 6.847090529943256065 ) ) ;
#121359=CARTESIAN_POINT ( 'NONE',  ( -21.14999999999999858, -11.65000000000000036, 3.469446951953614189E-15 ) ) ;
#121369=EDGE_LOOP ( 'NONE', ( #132613, #236467, #235584, #22875, #184612 ) ) ;
#121371=CIRCLE ( 'NONE', #664, 0.1000000000000017680 ) ;
#121407=CARTESIAN_POINT ( 'NONE',  ( 18.39999999999999858, -9.499999999999998224, -40.10018939122204529 ) ) ;
#121425=EDGE_LOOP ( 'NONE', ( #7812, #182609, #62100, #34493 ) ) ;
#121447=ADVANCED_FACE ( 'NONE', ( #210376 ), #53863, .F. ) ;
#121493=DIRECTION ( 'NONE',  ( -0.000000000000000000, -0.000000000000000000, 1.000000000000000000 ) ) ;
#121509=CARTESIAN_POINT ( 'NONE',  ( 18.59999999999999076, 1.835341550224411922, -11.55515129256298046 ) ) ;
#121525=DIRECTION ( 'NONE',  ( -1.000000000000000000, 0.000000000000000000, 0.000000000000000000 ) ) ;
#121537=ORIENTED_EDGE ( 'NONE', *, *, #230112, .T. ) ;
#121541=DIRECTION ( 'NONE',  ( 0.000000000000000000, 0.000000000000000000, -1.000000000000000000 ) ) ;
#121547=TOROIDAL_SURFACE ( 'NONE', #138243, 0.2000000000000000111, 0.1000000000000000056 ) ;
#121554=ORIENTED_EDGE ( 'NONE', *, *, #147470, .F. ) ;
#121555=CARTESIAN_POINT ( 'NONE',  ( -20.64999999999999858, 7.150000000000000355, -21.25000000000000000 ) ) ;
#121600=CARTESIAN_POINT ( 'NONE',  ( 18.46921299892753510, -9.509378177823768041, -6.986578709370435014 ) ) ;
#121614=VECTOR ( 'NONE', #145176, 1000.000000000000000 ) ;
#121619=CARTESIAN_POINT ( 'NONE',  ( 23.14999999999999858, 4.999999999999997335, -12.40526601891309788 ) ) ;
#121675=ORIENTED_EDGE ( 'NONE', *, *, #257492, .T. ) ;
#121689=DIRECTION ( 'NONE',  ( 1.000000000000000000, 0.000000000000000000, -0.000000000000000000 ) ) ;
#121690=ORIENTED_EDGE ( 'NONE', *, *, #210611, .T. ) ;
#121720=ADVANCED_FACE ( 'NONE', ( #119330 ), #20237, .T. ) ;
#121740=EDGE_LOOP ( 'NONE', ( #30987, #90681, #94407, #231324 ) ) ;
#121746=DIRECTION ( 'NONE',  ( 0.000000000000000000, 0.000000000000000000, -1.000000000000000000 ) ) ;
#121758=CARTESIAN_POINT ( 'NONE',  ( -20.85000000000000142, 7.021664781900089913, -37.33356540189728889 ) ) ;
#121766=EDGE_CURVE ( 'NONE', #187076, #43421, #5770, .T. ) ;
#121780=ORIENTED_EDGE ( 'NONE', *, *, #9684, .T. ) ;
#121785=CARTESIAN_POINT ( 'NONE',  ( 20.94999999999999929, 6.450000000000001066, -10.01702717044001822 ) ) ;
#121793=ORIENTED_EDGE ( 'NONE', *, *, #142941, .F. ) ;
#121796=CARTESIAN_POINT ( 'NONE',  ( -22.47071067811865319, 0.09909245470260577560, 7.720074744498064412 ) ) ;
#121813=CARTESIAN_POINT ( 'NONE',  ( -20.64999999999999858, 2.500000000000000444, -13.22462192276210224 ) ) ;
#121854=DIRECTION ( 'NONE',  ( 0.000000000000000000, -1.000000000000000000, 0.000000000000000000 ) ) ;
#121864=EDGE_CURVE ( 'NONE', #88270, #105026, #64060, .T. ) ;
#121890=VECTOR ( 'NONE', #167356, 1000.000000000000000 ) ;
#121916=EDGE_LOOP ( 'NONE', ( #129090, #255862, #16670, #69083 ) ) ;
#121924=CARTESIAN_POINT ( 'NONE',  ( 23.14999999999999503, 11.65000000000000746, -26.48519422934606027 ) ) ;
#121937=CARTESIAN_POINT ( 'NONE',  ( 20.94999999999999929, 0.000000000000000000, 0.000000000000000000 ) ) ;
#121965=CARTESIAN_POINT ( 'NONE',  ( 21.05000000000000071, 0.000000000000000000, 0.000000000000000000 ) ) ;
#122008=CARTESIAN_POINT ( 'NONE',  ( -20.94999999999999929, 0.000000000000000000, -33.50000000000000000 ) ) ;
#122014=DIRECTION ( 'NONE',  ( 0.000000000000000000, 0.7397360091702777085, -0.6728971962616808744 ) ) ;
#122037=VERTEX_POINT ( 'NONE', #60321 ) ;
#122051=ORIENTED_EDGE ( 'NONE', *, *, #45812, .T. ) ;
#122108=ORIENTED_EDGE ( 'NONE', *, *, #25466, .T. ) ;
#122150=CARTESIAN_POINT ( 'NONE',  ( -22.50875500270928953, -0.1008579137753043697, 11.74956712739789211 ) ) ;
#122168=EDGE_CURVE ( 'NONE', #81419, #142144, #139228, .T. ) ;
#122195=FACE_OUTER_BOUND ( 'NONE', #153601, .T. ) ;
#122205=CIRCLE ( 'NONE', #201302, 0.9750000000000036415 ) ;
#122223=DIRECTION ( 'NONE',  ( 0.000000000000000000, 0.000000000000000000, -1.000000000000000000 ) ) ;
#122241=CARTESIAN_POINT ( 'NONE',  ( 18.50000000000000000, -9.399999999999998579, -40.38204184817267617 ) ) ;
#122244=CYLINDRICAL_SURFACE ( 'NONE', #115388, 0.1000000000000008105 ) ;
#122268=VERTEX_POINT ( 'NONE', #71901 ) ;
#122279=DIRECTION ( 'NONE',  ( -3.890533409366484652E-14, -0.1298341882520124002, -0.9915357197604841577 ) ) ;
#122287=DIRECTION ( 'NONE',  ( 0.000000000000000000, 1.000000000000000000, 0.000000000000000000 ) ) ;
#122291=DIRECTION ( 'NONE',  ( -0.7071067811865475727, -0.7071067811865475727, 0.000000000000000000 ) ) ;
#122296=DIRECTION ( 'NONE',  ( 0.000000000000000000, 0.000000000000000000, -1.000000000000000000 ) ) ;
#122320=ORIENTED_EDGE ( 'NONE', *, *, #130745, .F. ) ;
#122333=DIRECTION ( 'NONE',  ( 0.000000000000000000, -0.000000000000000000, 1.000000000000000000 ) ) ;
#122335=ORIENTED_EDGE ( 'NONE', *, *, #169932, .F. ) ;
#122342=CARTESIAN_POINT ( 'NONE',  ( -22.39999999999999503, 7.790779598373400283, -1.558540622947912624E-15 ) ) ;
#122344=ORIENTED_EDGE ( 'NONE', *, *, #25314, .F. ) ;
#122353=CARTESIAN_POINT ( 'NONE',  ( -21.14999999999999858, 11.75000000000000000, -6.726130636059191481 ) ) ;
#122360=EDGE_CURVE ( 'NONE', #248548, #58858, #19625, .T. ) ;
#122390=CARTESIAN_POINT ( 'NONE',  ( -18.59999999999999787, 11.64999999999999680, -12.15000000000000036 ) ) ;
#122394=DIRECTION ( 'NONE',  ( -0.000000000000000000, 1.000000000000000000, -0.000000000000000000 ) ) ;
#122399=DIRECTION ( 'NONE',  ( -1.000000000000000000, 0.000000000000000000, 0.000000000000000000 ) ) ;
#122434=DIRECTION ( 'NONE',  ( 0.000000000000000000, 0.000000000000000000, 1.000000000000000000 ) ) ;
#122475=CARTESIAN_POINT ( 'NONE',  ( -23.25000000000000000, -11.65000000000000036, 3.469446951953614189E-15 ) ) ;
#122498=DIRECTION ( 'NONE',  ( 0.000000000000000000, 1.000000000000000000, -6.308085367188393199E-16 ) ) ;
#122517=CARTESIAN_POINT ( 'NONE',  ( -21.51976009735018991, 6.910458441659202755, 1.166362318020024071E-16 ) ) ;
#122537=EDGE_LOOP ( 'NONE', ( #78021, #27982, #87829, #39534 ) ) ;
#122551=ORIENTED_EDGE ( 'NONE', *, *, #92749, .F. ) ;
#122573=VERTEX_POINT ( 'NONE', #165555 ) ;
#122574=EDGE_LOOP ( 'NONE', ( #250695, #17706, #220449, #181767 ) ) ;
#122593=CIRCLE ( 'NONE', #10152, 0.1000000000000002831 ) ;
#122680=ORIENTED_EDGE ( 'NONE', *, *, #52177, .F. ) ;
#122706=MECHANICAL_DESIGN_GEOMETRIC_PRESENTATION_REPRESENTATION('',(#51925),#168520);
#122737=ORIENTED_EDGE ( 'NONE', *, *, #121766, .T. ) ;
#122751=DIRECTION ( 'NONE',  ( -0.000000000000000000, 0.000000000000000000, -1.000000000000000000 ) ) ;
#122806=ORIENTED_EDGE ( 'NONE', *, *, #37072, .F. ) ;
#122828=ORIENTED_EDGE ( 'NONE', *, *, #189155, .F. ) ;
#122836=ORIENTED_EDGE ( 'NONE', *, *, #111463, .F. ) ;
#122845=VECTOR ( 'NONE', #113506, 1000.000000000000000 ) ;
#122856=FACE_OUTER_BOUND ( 'NONE', #212221, .T. ) ;
#122876=ORIENTED_EDGE ( 'NONE', *, *, #82777, .F. ) ;
#122878=DIRECTION ( 'NONE',  ( 0.000000000000000000, 0.000000000000000000, 1.000000000000000000 ) ) ;
#122897=DIRECTION ( 'NONE',  ( 0.000000000000000000, 1.000000000000000000, 0.000000000000000000 ) ) ;
#122948=ORIENTED_EDGE ( 'NONE', *, *, #8973, .F. ) ;
#122963=EDGE_LOOP ( 'NONE', ( #118058, #244920, #22223, #249385 ) ) ;
#122975=CARTESIAN_POINT ( 'NONE',  ( -18.50000000000000000, 0.000000000000000000, -33.50000000000000000 ) ) ;
#122998=ADVANCED_FACE ( 'NONE', ( #31848 ), #154375, .T. ) ;
#123020=DIRECTION ( 'NONE',  ( 0.000000000000000000, 1.000000000000000000, 0.000000000000000000 ) ) ;
#123023=ORIENTED_EDGE ( 'NONE', *, *, #224893, .F. ) ;
#123027=EDGE_LOOP ( 'NONE', ( #87425, #193532, #152794, #190063 ) ) ;
#123032=DIRECTION ( 'NONE',  ( 0.000000000000000000, 5.329070518200751394E-15, -1.000000000000000000 ) ) ;
#123067=EDGE_LOOP ( 'NONE', ( #214773, #27749, #129325, #123023 ) ) ;
#123081=VECTOR ( 'NONE', #151414, 1000.000000000000000 ) ;
#123102=CARTESIAN_POINT ( 'NONE',  ( -20.85000000000000142, -0.3238857010703366512, -33.45758958931398297 ) ) ;
#123104=ORIENTED_EDGE ( 'NONE', *, *, #134239, .T. ) ;
#123130=DIRECTION ( 'NONE',  ( -1.000000000000000000, 0.000000000000000000, 0.000000000000000000 ) ) ;
#123177=CARTESIAN_POINT ( 'NONE',  ( -21.55000000000000071, 7.249999999999999112, -12.34999999999999964 ) ) ;
#123182=EDGE_CURVE ( 'NONE', #56184, #150108, #17393, .T. ) ;
#123184=EDGE_CURVE ( 'NONE', #155798, #16790, #218134, .T. ) ;
#123188=ORIENTED_EDGE ( 'NONE', *, *, #120942, .F. ) ;
#123212=EDGE_CURVE ( 'NONE', #97122, #67614, #193058, .T. ) ;
#123223=CIRCLE ( 'NONE', #248123, 0.09999999999999993616 ) ;
#123226=AXIS2_PLACEMENT_3D ( 'NONE', #81873, #126154, #181029 ) ;
#123239=CARTESIAN_POINT ( 'NONE',  ( -23.15000000000000213, 11.75000000000000000, 11.75000000000000000 ) ) ;
#123242=ORIENTED_EDGE ( 'NONE', *, *, #107989, .T. ) ;
#123253=EDGE_CURVE ( 'NONE', #142144, #63069, #164009, .T. ) ;
#123308=DIRECTION ( 'NONE',  ( 0.000000000000000000, -1.000000000000000000, 0.000000000000000000 ) ) ;
#123328=DIRECTION ( 'NONE',  ( 1.000000000000000000, -0.000000000000000000, -0.000000000000000000 ) ) ;
#123338=VERTEX_POINT ( 'NONE', #51039 ) ;
#123359=ORIENTED_EDGE ( 'NONE', *, *, #112310, .T. ) ;
#123370=EDGE_CURVE ( 'NONE', #193883, #141135, #55815, .T. ) ;
#123378=DIRECTION ( 'NONE',  ( 0.000000000000000000, 0.000000000000000000, -1.000000000000000000 ) ) ;
#123384=CARTESIAN_POINT ( 'NONE',  ( -20.94999999999999929, 7.021664781900089913, -37.33356540189728889 ) ) ;
#123402=CYLINDRICAL_SURFACE ( 'NONE', #100836, 2.000000000000001776 ) ;
#123407=EDGE_CURVE ( 'NONE', #210905, #20887, #184836, .T. ) ;
#123432=ADVANCED_FACE ( 'NONE', ( #189314 ), #247985, .T. ) ;
#123437=EDGE_LOOP ( 'NONE', ( #109543, #226428, #180123, #113525 ) ) ;
#123454=ORIENTED_EDGE ( 'NONE', *, *, #150075, .T. ) ;
#123457=CARTESIAN_POINT ( 'NONE',  ( -22.39999999999999858, 0.000000000000000000, 0.1000000000000028644 ) ) ;
#123461=CARTESIAN_POINT ( 'NONE',  ( -21.05000000000000071, 1.749999999999999778, -11.66951155790164307 ) ) ;
#123464=DIRECTION ( 'NONE',  ( -1.000000000000000000, 0.000000000000000000, 0.000000000000000000 ) ) ;
#123470=CARTESIAN_POINT ( 'NONE',  ( 18.47688499308725341, -9.464855950284134067, -40.20134775313739794 ) ) ;
#123487=ADVANCED_FACE ( 'NONE', ( #157933 ), #20971, .F. ) ;
#123494=ORIENTED_EDGE ( 'NONE', *, *, #35571, .F. ) ;
#123525=CARTESIAN_POINT ( 'NONE',  ( 18.59999999999999076, 5.949999999999945111, -10.30570230503485973 ) ) ;
#123536=CARTESIAN_POINT ( 'NONE',  ( 21.05000000000000071, 4.999999999999997335, -21.09473398108690390 ) ) ;
#123590=CARTESIAN_POINT ( 'NONE',  ( 20.95512820512820440, 8.876151316288115822, -12.15000000000000036 ) ) ;
#123595=EDGE_CURVE ( 'NONE', #184931, #163009, #215286, .T. ) ;
#123624=CIRCLE ( 'NONE', #102739, 0.09999999999999939493 ) ;
#123630=CARTESIAN_POINT ( 'NONE',  ( -21.93340585971863277, 7.324147022855313161, -1.264184810800004045E-15 ) ) ;
#123638=LINE ( 'NONE', #225269, #19829 ) ;
#123641=VERTEX_POINT ( 'NONE', #125185 ) ;
#123661=LINE ( 'NONE', #6252, #28917 ) ;
#123668=ORIENTED_EDGE ( 'NONE', *, *, #234840, .F. ) ;
#123716=ORIENTED_EDGE ( 'NONE', *, *, #213948, .F. ) ;
#123726=B_SPLINE_CURVE_WITH_KNOTS ( 'NONE', 3,
 ( #82324, #182760, #4103, #163191, #242705, #64077, #143612, #223142 ),
 .UNSPECIFIED., .F., .F.,
 ( 4, 2, 2, 4 ),
 ( 0.000000000000000000, 0.0001306511400391334671, 0.0001959767100587002007, 0.0002613022800782669342 ),
 .UNSPECIFIED. ) ;
#123734=ORIENTED_EDGE ( 'NONE', *, *, #144141, .F. ) ;
#123757=CARTESIAN_POINT ( 'NONE',  ( -20.54999999999999716, 9.350000000000001421, -12.25000000000000000 ) ) ;
#123764=LINE ( 'NONE', #100315, #175542 ) ;
#123769=DIRECTION ( 'NONE',  ( 0.000000000000000000, 0.000000000000000000, 1.000000000000000000 ) ) ;
#123833=AXIS2_PLACEMENT_3D ( 'NONE', #68154, #29070, #94132 ) ;
#123879=CIRCLE ( 'NONE', #69712, 11.90000000000000036 ) ;
#123898=CARTESIAN_POINT ( 'NONE',  ( -22.39999999999999858, 0.09999999999999939493, 7.790779598373403836 ) ) ;
#123940=DIRECTION ( 'NONE',  ( -1.000000000000000000, -0.000000000000000000, -0.000000000000000000 ) ) ;
#123965=TOROIDAL_SURFACE ( 'NONE', #36688, 0.2000000000000000111, 0.1000000000000000056 ) ;
#123974=DIRECTION ( 'NONE',  ( 0.000000000000000000, -0.1455152366551522025, -0.9893560106964505163 ) ) ;
#123995=FACE_OUTER_BOUND ( 'NONE', #175960, .T. ) ;
#124010=CARTESIAN_POINT ( 'NONE',  ( 21.33487959338958362, 6.725558151911193328, -1.166372555419950539E-16 ) ) ;
#124018=CIRCLE ( 'NONE', #7470, 0.09999999999999939493 ) ;
#124048=DIRECTION ( 'NONE',  ( 0.000000000000000000, 1.000000000000000000, 0.000000000000000000 ) ) ;
#124061=EDGE_CURVE ( 'NONE', #75474, #88270, #193433, .T. ) ;
#124072=CARTESIAN_POINT ( 'NONE',  ( -18.59999999999999787, 11.74999999999999645, 11.75000000000000000 ) ) ;
#124115=CYLINDRICAL_SURFACE ( 'NONE', #157681, 11.74999999999999645 ) ;
#124127=LINE ( 'NONE', #224483, #72773 ) ;
#124135=EDGE_CURVE ( 'NONE', #73708, #38660, #10441, .T. ) ;
#124145=CIRCLE ( 'NONE', #61588, 11.80000000000000426 ) ;
#124153=EDGE_CURVE ( 'NONE', #239230, #44201, #151921, .T. ) ;
#124159=ORIENTED_EDGE ( 'NONE', *, *, #250545, .T. ) ;
#124163=VERTEX_POINT ( 'NONE', #29644 ) ;
#124167=ORIENTED_EDGE ( 'NONE', *, *, #174718, .F. ) ;
#124200=ORIENTED_EDGE ( 'NONE', *, *, #41213, .T. ) ;
#124201=EDGE_CURVE ( 'NONE', #163039, #180993, #214422, .T. ) ;
#124226=VERTEX_POINT ( 'NONE', #137673 ) ;
#124233=VECTOR ( 'NONE', #43560, 1000.000000000000114 ) ;
#124278=CIRCLE ( 'NONE', #165987, 12.87499999999999822 ) ;
#124299=AXIS2_PLACEMENT_3D ( 'NONE', #169224, #128788, #170529 ) ;
#124310=AXIS2_PLACEMENT_3D ( 'NONE', #96624, #154116, #195789 ) ;
#124311=AXIS2_PLACEMENT_3D ( 'NONE', #8645, #230251, #51583 ) ;
#124313=CARTESIAN_POINT ( 'NONE',  ( 20.85000000000000142, -1.835859311443637010, -45.00443916879852679 ) ) ;
#124330=ADVANCED_FACE ( 'NONE', ( #157286 ), #75182, .T. ) ;
#124339=CYLINDRICAL_SURFACE ( 'NONE', #143183, 2.000000000000001776 ) ;
#124342=DIRECTION ( 'NONE',  ( -1.000000000000000000, 0.000000000000000000, 0.000000000000000000 ) ) ;
#124343=ADVANCED_FACE ( 'NONE', ( #133841 ), #36044, .F. ) ;
#124346=AXIS2_PLACEMENT_3D ( 'NONE', #150084, #229603, #130485 ) ;
#124367=ORIENTED_EDGE ( 'NONE', *, *, #111360, .F. ) ;
#124397=VECTOR ( 'NONE', #99055, 1000.000000000000000 ) ;
#124405=DIRECTION ( 'NONE',  ( 1.000000000000000000, 0.000000000000000000, -0.000000000000000000 ) ) ;
#124407=DIRECTION ( 'NONE',  ( 0.000000000000000000, 0.9654727137038815465, -0.2605042016806309868 ) ) ;
#124426=EDGE_CURVE ( 'NONE', #92976, #174229, #93636, .T. ) ;
#124441=EDGE_CURVE ( 'NONE', #68319, #210177, #59400, .T. ) ;
#124449=DIRECTION ( 'NONE',  ( 0.000000000000000000, 0.000000000000000000, -1.000000000000000000 ) ) ;
#124466=AXIS2_PLACEMENT_3D ( 'NONE', #167091, #67952, #134017 ) ;
#124467=EDGE_CURVE ( 'NONE', #123641, #70529, #160308, .T. ) ;
#124508=LINE ( 'NONE', #204030, #139637 ) ;
#124538=ORIENTED_EDGE ( 'NONE', *, *, #97858, .F. ) ;
#124549=CARTESIAN_POINT ( 'NONE',  ( -20.94999999999999929, -1.835341550224411922, -11.55515129256297868 ) ) ;
#124550=DIRECTION ( 'NONE',  ( 1.000000000000000000, 0.000000000000000000, 0.000000000000000000 ) ) ;
#124574=CARTESIAN_POINT ( 'NONE',  ( 18.49999999999996803, 7.070967871798842452, -37.24656422186831151 ) ) ;
#124579=AXIS2_PLACEMENT_3D ( 'NONE', #132791, #32423, #49387 ) ;
#124593=EDGE_CURVE ( 'NONE', #150376, #6293, #14737, .T. ) ;
#124604=CARTESIAN_POINT ( 'NONE',  ( 21.87500000000000355, 9.749999999999998224, -12.35000000000000320 ) ) ;
#124619=CARTESIAN_POINT ( 'NONE',  ( 21.30000000000002558, 0.000000000000000000, -4.049999999999998934 ) ) ;
#124625=ORIENTED_EDGE ( 'NONE', *, *, #213042, .F. ) ;
#124656=CYLINDRICAL_SURFACE ( 'NONE', #236144, 0.1000000000000000472 ) ;
#124659=AXIS2_PLACEMENT_3D ( 'NONE', #74655, #122751, #180148 ) ;
#124694=DIRECTION ( 'NONE',  ( -1.000000000000000000, 7.304098846218134667E-16, -4.217023435051678980E-16 ) ) ;
#124709=DIRECTION ( 'NONE',  ( -1.000000000000000000, -0.000000000000000000, -0.000000000000000000 ) ) ;
#124713=AXIS2_PLACEMENT_3D ( 'NONE', #26958, #226383, #64763 ) ;
#124730=CARTESIAN_POINT ( 'NONE',  ( 22.49231231312462853, 11.64998490367728223, 0.06105288760137694143 ) ) ;
#124752=CARTESIAN_POINT ( 'NONE',  ( -18.43473496883415663, -9.494952410999301762, -7.045871572228188384 ) ) ;
#124812=DIRECTION ( 'NONE',  ( 0.000000000000000000, 0.000000000000000000, -1.000000000000000000 ) ) ;
#124814=ADVANCED_FACE ( 'NONE', ( #45675 ), #143486, .T. ) ;
#124817=AXIS2_PLACEMENT_3D ( 'NONE', #249706, #182371, #3711 ) ;
#124825=DIRECTION ( 'NONE',  ( 0.000000000000000000, 0.000000000000000000, -1.000000000000000000 ) ) ;
#124826=( BOUNDED_SURFACE ( )  B_SPLINE_SURFACE ( 3, 2, ( 
 ( #16954, #18228, #116056 ),
 ( #176039, #14399, #35252 ),
 ( #212586, #195600, #114757 ),
 ( #58612, #178609, #193018 ),
 ( #113464, #75651, #258068 ),
 ( #255496, #135581, #37811 ) ),
 .UNSPECIFIED., .F., .F., .F. ) 
 B_SPLINE_SURFACE_WITH_KNOTS ( ( 4, 2, 4 ),
 ( 3, 3 ),
 ( 3.141592653589793116, 3.926990816987241395, 4.712388980384689674 ),
 ( 0.000000000000000000, 1.000000000000000000 ),
 .UNSPECIFIED. ) 
 GEOMETRIC_REPRESENTATION_ITEM ( )  RATIONAL_B_SPLINE_SURFACE ( (
 ( 1.000000000000000000, 0.9238795325112820755, 1.000000000000000000),
 ( 1.000000000000000000, 0.9240297172245068857, 1.000000000000000000),
 ( 1.000000000000000000, 0.9038128468037387453, 1.000000000000000000),
 ( 1.000000000000000000, 0.8282379607651308984, 1.000000000000000000),
 ( 1.000000000000000000, 0.7727932973489990420, 1.000000000000000000),
 ( 1.000000000000000000, 0.7071067811865352493, 1.000000000000000000) ) ) 
 REPRESENTATION_ITEM ( '' )  SURFACE ( )  );
#124884=CARTESIAN_POINT ( 'NONE',  ( -18.59999999999999787, 6.982009704856444898, -37.19615211825629331 ) ) ;
#124892=CARTESIAN_POINT ( 'NONE',  ( -2.995603634470884209E-16, 6.649999999999999467, -21.25000000000000000 ) ) ;
#124917=CARTESIAN_POINT ( 'NONE',  ( -22.47071067811865319, 7.720074744498060859, 0.09909245470260481803 ) ) ;
#124927=ORIENTED_EDGE ( 'NONE', *, *, #180986, .T. ) ;
#124964=DIRECTION ( 'NONE',  ( 3.469446951953635015E-14, -0.000000000000000000, 1.000000000000000000 ) ) ;
#125014=CARTESIAN_POINT ( 'NONE',  ( 20.94999999999999929, -9.000000000000000000, -24.10603087734755690 ) ) ;
#125068=CARTESIAN_POINT ( 'NONE',  ( 21.46681500593309622, 6.857511159384197974, -9.855405879750058190E-16 ) ) ;
#125080=EDGE_CURVE ( 'NONE', #132561, #250352, #144292, .T. ) ;
#125099=VECTOR ( 'NONE', #119997, 999.9999999999998863 ) ;
#125114=AXIS2_PLACEMENT_3D ( 'NONE', #174006, #57837, #74891 ) ;
#125167=DIRECTION ( 'NONE',  ( 1.000000000000000000, -0.000000000000000000, -0.000000000000000000 ) ) ;
#125185=CARTESIAN_POINT ( 'NONE',  ( 20.94999999999999574, 1.835341550224411922, -11.65515129256298010 ) ) ;
#125208=CARTESIAN_POINT ( 'NONE',  ( 20.85000000000000142, -1.164121893241208960, -41.41484808557160591 ) ) ;
#125215=CARTESIAN_POINT ( 'NONE',  ( -20.64999999999999858, 0.000000000000000000, 0.000000000000000000 ) ) ;
#125216=VERTEX_POINT ( 'NONE', #129884 ) ;
#125223=CARTESIAN_POINT ( 'NONE',  ( -21.14999999999999858, -11.65000000000000036, -2.900000000000001688 ) ) ;
#125238=DIRECTION ( 'NONE',  ( -0.000000000000000000, 0.000000000000000000, 1.000000000000000000 ) ) ;
#125263=AXIS2_PLACEMENT_3D ( 'NONE', #166618, #240995, #3650 ) ;
#125297=CARTESIAN_POINT ( 'NONE',  ( 18.44364597020194907, -9.490487317162260794, -7.057977889683861861 ) ) ;
#125305=EDGE_CURVE ( 'NONE', #244818, #113723, #168735, .T. ) ;
#125312=DIRECTION ( 'NONE',  ( 0.000000000000000000, 0.000000000000000000, -1.000000000000000000 ) ) ;
#125353=ORIENTED_EDGE ( 'NONE', *, *, #93888, .T. ) ;
#125397=CARTESIAN_POINT ( 'NONE',  ( -23.15000000000000213, 11.75000000000000711, -12.15000000000000036 ) ) ;
#125432=VECTOR ( 'NONE', #11830, 1000.000000000000000 ) ;
#125440=DIRECTION ( 'NONE',  ( 0.000000000000000000, 0.000000000000000000, 1.000000000000000000 ) ) ;
#125447=CARTESIAN_POINT ( 'NONE',  ( -21.05000000000000071, 0.000000000000000000, -33.50000000000000000 ) ) ;
#125473=DIRECTION ( 'NONE',  ( 1.000000000000000000, -0.000000000000000000, -0.000000000000000000 ) ) ;
#125479=ORIENTED_EDGE ( 'NONE', *, *, #19245, .T. ) ;
#125490=ORIENTED_EDGE ( 'NONE', *, *, #171103, .F. ) ;
#125491=ORIENTED_EDGE ( 'NONE', *, *, #39522, .F. ) ;
#125515=CARTESIAN_POINT ( 'NONE',  ( -18.59999999999999787, -1.835859311443637010, -45.00443916879852679 ) ) ;
#125519=DIRECTION ( 'NONE',  ( 1.000000000000000000, 0.000000000000000000, -0.000000000000000000 ) ) ;
#125564=DIRECTION ( 'NONE',  ( 0.000000000000000000, -1.000000000000000000, 0.000000000000000000 ) ) ;
#125577=EDGE_CURVE ( 'NONE', #27728, #193883, #189200, .T. ) ;
#125593=DIRECTION ( 'NONE',  ( 3.616040088954497272E-32, -1.224646799147352961E-16, 1.000000000000000000 ) ) ;
#125598=DIRECTION ( 'NONE',  ( 0.000000000000000000, 0.000000000000000000, -1.000000000000000000 ) ) ;
#125653=EDGE_CURVE ( 'NONE', #154965, #141135, #223345, .T. ) ;
#125664=ORIENTED_EDGE ( 'NONE', *, *, #161146, .T. ) ;
#125691=AXIS2_PLACEMENT_3D ( 'NONE', #252916, #136819, #168625 ) ;
#125701=DIRECTION ( 'NONE',  ( 0.000000000000000000, -1.000000000000000000, -0.000000000000000000 ) ) ;
#125712=CARTESIAN_POINT ( 'NONE',  ( -20.85000000000000142, 7.021664781900089913, -37.23356540189728747 ) ) ;
#125721=ORIENTED_EDGE ( 'NONE', *, *, #28206, .F. ) ;
#125751=CARTESIAN_POINT ( 'NONE',  ( -20.64999999999999858, 0.000000000000000000, 0.000000000000000000 ) ) ;
#125755=CARTESIAN_POINT ( 'NONE',  ( -18.59999999999999787, 0.000000000000000000, -33.50000000000000000 ) ) ;
#125790=CARTESIAN_POINT ( 'NONE',  ( 18.59999999999999076, 0.000000000000000000, -33.50000000000000000 ) ) ;
#125791=EDGE_CURVE ( 'NONE', #108350, #155798, #219425, .T. ) ;
#125793=ORIENTED_EDGE ( 'NONE', *, *, #104963, .T. ) ;
#125801=AXIS2_PLACEMENT_3D ( 'NONE', #127018, #47455, #229966 ) ;
#125808=CARTESIAN_POINT ( 'NONE',  ( 20.12500000000000000, 9.749999999999998224, -8.111771282114276005 ) ) ;
#125824=EDGE_CURVE ( 'NONE', #255533, #44715, #182484, .T. ) ;
#125832=ORIENTED_EDGE ( 'NONE', *, *, #241044, .F. ) ;
#125833=DIRECTION ( 'NONE',  ( 0.000000000000000000, 0.000000000000000000, 1.000000000000000000 ) ) ;
#125844=CARTESIAN_POINT ( 'NONE',  ( 23.14999999999999503, 11.65000000000000746, -26.48519422934605672 ) ) ;
#125862=ORIENTED_EDGE ( 'NONE', *, *, #79979, .F. ) ;
#125874=CARTESIAN_POINT ( 'NONE',  ( -20.85000000000000142, 0.000000000000000000, -33.50000000000000000 ) ) ;
#125876=ADVANCED_FACE ( 'NONE', ( #171595 ), #194353, .F. ) ;
#125895=DIRECTION ( 'NONE',  ( 0.000000000000000000, 1.000000000000000000, 0.000000000000000000 ) ) ;
#125910=FACE_OUTER_BOUND ( 'NONE', #31871, .T. ) ;
#125933=DIRECTION ( 'NONE',  ( 1.000000000000000000, -0.000000000000000000, 0.000000000000000000 ) ) ;
#125943=VECTOR ( 'NONE', #247743, 1000.000000000000000 ) ;
#125952=DIRECTION ( 'NONE',  ( -1.000000000000000000, 0.000000000000000000, 0.000000000000000000 ) ) ;
#126009=FACE_OUTER_BOUND ( 'NONE', #121369, .T. ) ;
#126015=CARTESIAN_POINT ( 'NONE',  ( -18.49346865148320518, -9.443073798524933338, -7.185196255314905578 ) ) ;
#126031=CARTESIAN_POINT ( 'NONE',  ( -1.739115166359751801E-14, 11.64999999999998970, -12.25000000000000000 ) ) ;
#126038=VERTEX_POINT ( 'NONE', #42325 ) ;
#126055=ORIENTED_EDGE ( 'NONE', *, *, #186790, .T. ) ;
#126058=DIRECTION ( 'NONE',  ( 0.000000000000000000, 0.000000000000000000, -1.000000000000000000 ) ) ;
#126060=ORIENTED_EDGE ( 'NONE', *, *, #63368, .T. ) ;
#126066=DIRECTION ( 'NONE',  ( -1.000000000000000000, 0.000000000000000000, 0.000000000000000000 ) ) ;
#126083=DIRECTION ( 'NONE',  ( 0.000000000000000000, 0.000000000000000000, -1.000000000000000000 ) ) ;
#126093=CYLINDRICAL_SURFACE ( 'NONE', #90755, 0.09999999999999939493 ) ;
#126134=ORIENTED_EDGE ( 'NONE', *, *, #140101, .T. ) ;
#126154=DIRECTION ( 'NONE',  ( 0.000000000000000000, -1.000000000000000000, -0.000000000000000000 ) ) ;
#126171=VERTEX_POINT ( 'NONE', #7041 ) ;
#126181=CIRCLE ( 'NONE', #42424, 0.09999999999999954758 ) ;
#126235=AXIS2_PLACEMENT_3D ( 'NONE', #58449, #221373, #256614 ) ;
#126236=CYLINDRICAL_SURFACE ( 'NONE', #17001, 0.1000000000000028644 ) ;
#126268=DIRECTION ( 'NONE',  ( 1.000000000000000000, 0.000000000000000000, 0.000000000000000000 ) ) ;
#126293=DIRECTION ( 'NONE',  ( 1.000000000000000000, -0.000000000000000000, -0.000000000000000000 ) ) ;
#126324=ORIENTED_EDGE ( 'NONE', *, *, #31943, .T. ) ;
#126332=CARTESIAN_POINT ( 'NONE',  ( 21.05000000000000071, 6.649999999999999467, -9.843822089683124332 ) ) ;
#126365=AXIS2_PLACEMENT_3D ( 'NONE', #125755, #90483, #246988 ) ;
#126398=ORIENTED_EDGE ( 'NONE', *, *, #256833, .F. ) ;
#126468=ORIENTED_EDGE ( 'NONE', *, *, #77684, .T. ) ;
#126469=CARTESIAN_POINT ( 'NONE',  ( 23.14999999999999858, 4.813084112149527805, -21.55848224347618114 ) ) ;
#126495=DIRECTION ( 'NONE',  ( 1.000000000000000000, 0.000000000000000000, 0.000000000000000000 ) ) ;
#126502=AXIS2_PLACEMENT_3D ( 'NONE', #125515, #146345, #168547 ) ;
#126504=EDGE_LOOP ( 'NONE', ( #140109, #256965, #148415, #249051, #175044 ) ) ;
#126520=EDGE_LOOP ( 'NONE', ( #15428, #220207, #80128, #131481, #159625 ) ) ;
#126534=AXIS2_PLACEMENT_3D ( 'NONE', #161140, #116869, #136397 ) ;
#126569=EDGE_CURVE ( 'NONE', #106788, #69230, #136384, .T. ) ;
#126573=CARTESIAN_POINT ( 'NONE',  ( -21.05000000000000071, -7.589415207398530052E-16, 6.540656951701240729 ) ) ;
#126630=DIRECTION ( 'NONE',  ( 0.000000000000000000, 0.01562499999998609446, -0.9998779222360101304 ) ) ;
#126655=CARTESIAN_POINT ( 'NONE',  ( -20.85000000000000142, 0.000000000000000000, -33.50000000000000000 ) ) ;
#126682=ORIENTED_EDGE ( 'NONE', *, *, #218958, .F. ) ;
#126688=AXIS2_PLACEMENT_3D ( 'NONE', #99064, #203335, #239901 ) ;
#126711=CARTESIAN_POINT ( 'NONE',  ( 22.39999999999999503, -0.09999999999999939493, 11.64957080754479968 ) ) ;
#126726=ADVANCED_FACE ( 'NONE', ( #20895 ), #100371, .F. ) ;
#126743=EDGE_CURVE ( 'NONE', #109777, #71883, #232313, .T. ) ;
#126753=VECTOR ( 'NONE', #36300, 1000.000000000000000 ) ;
#126759=ADVANCED_FACE ( 'NONE', ( #246332 ), #243763, .F. ) ;
#126780=VERTEX_POINT ( 'NONE', #226759 ) ;
#126819=ORIENTED_EDGE ( 'NONE', *, *, #92395, .F. ) ;
#126846=AXIS2_PLACEMENT_3D ( 'NONE', #241216, #142089, #121295 ) ;
#126891=CARTESIAN_POINT ( 'NONE',  ( 21.07928932188134397, 6.328516656393303741, 0.09889514565439641580 ) ) ;
#126923=CYLINDRICAL_SURFACE ( 'NONE', #73500, 0.09999999999999939493 ) ;
#126929=CARTESIAN_POINT ( 'NONE',  ( 20.96428641294230033, 11.75000000000034461, -26.67489317794139936 ) ) ;
#126950=CARTESIAN_POINT ( 'NONE',  ( 21.05000000000000071, 10.48443348964172728, -7.456805801491905861 ) ) ;
#126989=EDGE_CURVE ( 'NONE', #106788, #134956, #131513, .T. ) ;
#126997=CARTESIAN_POINT ( 'NONE',  ( 23.25000000000000355, -22.45632476062292326, -6.793898447731608670 ) ) ;
#127018=CARTESIAN_POINT ( 'NONE',  ( 18.59999999999999076, 1.835341550224411922, -11.55515129256298046 ) ) ;
#127019=ORIENTED_EDGE ( 'NONE', *, *, #31088, .F. ) ;
#127020=CARTESIAN_POINT ( 'NONE',  ( -21.05000000000000071, 14.05000000000000071, -5.513695070760990191 ) ) ;
#127025=EDGE_CURVE ( 'NONE', #160332, #122268, #24689, .T. ) ;
#127046=EDGE_CURVE ( 'NONE', #34172, #202111, #245429, .T. ) ;
#127093=CARTESIAN_POINT ( 'NONE',  ( 21.05000000000000071, -1.360870587192041681, -8.072997927090961312 ) ) ;
#127110=ORIENTED_EDGE ( 'NONE', *, *, #160580, .T. ) ;
#127137=AXIS2_PLACEMENT_3D ( 'NONE', #77082, #19699, #18397 ) ;
#127168=CYLINDRICAL_SURFACE ( 'NONE', #206831, 2.000000000000001776 ) ;
#127175=ORIENTED_EDGE ( 'NONE', *, *, #143834, .T. ) ;
#127196=CARTESIAN_POINT ( 'NONE',  ( 18.39999999999999858, -9.519327731092436906, -6.972976376559336664 ) ) ;
#127245=AXIS2_PLACEMENT_3D ( 'NONE', #203264, #142000, #42915 ) ;
#127259=EDGE_CURVE ( 'NONE', #19688, #158624, #58313, .T. ) ;
#127264=ORIENTED_EDGE ( 'NONE', *, *, #12603, .T. ) ;
#127300=CIRCLE ( 'NONE', #102320, 0.09999999999999939493 ) ;
#127311=CARTESIAN_POINT ( 'NONE',  ( -18.41799967126733506, -9.500000000000007105, -7.032069813255726665 ) ) ;
#127318=SPHERICAL_SURFACE ( 'NONE', #201913, 0.1000000000000000056 ) ;
#127319=VECTOR ( 'NONE', #146868, 1000.000000000000000 ) ;
#127327=CYLINDRICAL_SURFACE ( 'NONE', #247786, 0.09999999999999939493 ) ;
#127360=VERTEX_POINT ( 'NONE', #231602 ) ;
#127367=DIRECTION ( 'NONE',  ( 0.7071067811865475727, -0.7071067811865475727, 0.000000000000000000 ) ) ;
#127395=EDGE_LOOP ( 'NONE', ( #207446, #180300, #26678, #177700 ) ) ;
#127403=AXIS2_PLACEMENT_3D ( 'NONE', #176501, #233889, #236452 ) ;
#127418=SPHERICAL_SURFACE ( 'NONE', #172662, 0.1000000000000000056 ) ;
#127425=DIRECTION ( 'NONE',  ( 0.7071067811865388020, -0.7071067811865561215, 0.000000000000000000 ) ) ;
#127432=CARTESIAN_POINT ( 'NONE',  ( 22.39999999999999858, 0.000000000000000000, 0.000000000000000000 ) ) ;
#127450=ORIENTED_EDGE ( 'NONE', *, *, #99381, .F. ) ;
#127472=VERTEX_POINT ( 'NONE', #16415 ) ;
#127498=FACE_OUTER_BOUND ( 'NONE', #90953, .T. ) ;
#127540=CARTESIAN_POINT ( 'NONE',  ( 21.04999999999908411, 8.776282895290673736, -12.15790900265250052 ) ) ;
#127541=CARTESIAN_POINT ( 'NONE',  ( 21.00000000000000000, 9.749999999999998224, -12.35000000000000320 ) ) ;
#127601=CARTESIAN_POINT ( 'NONE',  ( -20.85000000000000142, 7.070967871798842452, -37.24656422186831151 ) ) ;
#127603=LINE ( 'NONE', #123757, #104886 ) ;
#127637=CIRCLE ( 'NONE', #227574, 0.09999999999999939493 ) ;
#127687=EDGE_CURVE ( 'NONE', #73461, #199162, #210134, .T. ) ;
#127751=CIRCLE ( 'NONE', #244433, 0.1000000000000003803 ) ;
#127760=DIRECTION ( 'NONE',  ( 0.000000000000000000, 1.000000000000000000, 0.000000000000000000 ) ) ;
#127768=ORIENTED_EDGE ( 'NONE', *, *, #8973, .T. ) ;
#127799=VERTEX_POINT ( 'NONE', #41779 ) ;
#127899=CARTESIAN_POINT ( 'NONE',  ( 21.30000000000002558, 0.000000000000000000, 0.000000000000000000 ) ) ;
#127903=DIRECTION ( 'NONE',  ( 0.000000000000000000, 0.000000000000000000, -1.000000000000000000 ) ) ;
#127917=ORIENTED_EDGE ( 'NONE', *, *, #6457, .F. ) ;
#127962=AXIS2_PLACEMENT_3D ( 'NONE', #38711, #175659, #21714 ) ;
#127968=DIRECTION ( 'NONE',  ( 0.000000000000000000, 1.000000000000000000, 0.000000000000000000 ) ) ;
#127984=DIRECTION ( 'NONE',  ( 0.000000000000000000, 0.000000000000000000, -1.000000000000000000 ) ) ;
#128000=EDGE_CURVE ( 'NONE', #106299, #174560, #36648, .T. ) ;
#128006=VERTEX_POINT ( 'NONE', #70339 ) ;
#128017=CARTESIAN_POINT ( 'NONE',  ( -23.25000000000000000, 0.000000000000000000, 0.000000000000000000 ) ) ;
#128023=EDGE_CURVE ( 'NONE', #62457, #62255, #37612, .T. ) ;
#128084=CIRCLE ( 'NONE', #232149, 0.09999999999999939493 ) ;
#128093=VERTEX_POINT ( 'NONE', #19312 ) ;
#128111=EDGE_LOOP ( 'NONE', ( #246802, #49042, #64562, #83525 ) ) ;
#128148=CARTESIAN_POINT ( 'NONE',  ( -23.15000000000000213, 0.000000000000000000, -37.40000000000000568 ) ) ;
#128186=FACE_OUTER_BOUND ( 'NONE', #244978, .T. ) ;
#128201=AXIS2_PLACEMENT_3D ( 'NONE', #253360, #155592, #192132 ) ;
#128230=CARTESIAN_POINT ( 'NONE',  ( 20.94999999999999929, 0.000000000000000000, -33.50000000000000000 ) ) ;
#128236=EDGE_LOOP ( 'NONE', ( #53768, #219704, #26396, #137765, #184509, #21342, #173701, #197872, #221000, #247602, #188470, #67148, #129874, #257937, #212784, #108260, #220533, #217526, #194325, #109977, #211711, #125479, #198200 ) ) ;
#128247=CARTESIAN_POINT ( 'NONE',  ( -21.05000000000000071, 6.300000000000014033, -0.09999999999999939493 ) ) ;
#128270=ADVANCED_FACE ( 'NONE', ( #3591 ), #126093, .F. ) ;
#128299=ORIENTED_EDGE ( 'NONE', *, *, #78700, .F. ) ;
#128305=DIRECTION ( 'NONE',  ( 1.000000000000000000, 2.952720810173289112E-16, -0.000000000000000000 ) ) ;
#128323=CARTESIAN_POINT ( 'NONE',  ( 18.59999999999999432, -1.736257131597395809, -11.56865232901749785 ) ) ;
#128334=CIRCLE ( 'NONE', #165758, 0.1999999999999987899 ) ;
#128340=DIRECTION ( 'NONE',  ( 1.000000000000000000, -0.000000000000000000, -0.000000000000000000 ) ) ;
#128385=EDGE_CURVE ( 'NONE', #65265, #57106, #138767, .T. ) ;
#128432=FACE_OUTER_BOUND ( 'NONE', #10150, .T. ) ;
#128436=FACE_OUTER_BOUND ( 'NONE', #103264, .T. ) ;
#128451=VECTOR ( 'NONE', #81567, 1000.000000000000000 ) ;
#128468=CARTESIAN_POINT ( 'NONE',  ( 21.05000000000000071, 0.000000000000000000, 0.000000000000000000 ) ) ;
#128488=ORIENTED_EDGE ( 'NONE', *, *, #255058, .F. ) ;
#128502=DIRECTION ( 'NONE',  ( 0.000000000000000000, 0.000000000000000000, -1.000000000000000000 ) ) ;
#128549=CARTESIAN_POINT ( 'NONE',  ( 20.94999027547553894, 10.29326151434211489, -38.95928225104149334 ) ) ;
#128560=DIRECTION ( 'NONE',  ( 1.000000000000000000, 0.000000000000000000, -0.000000000000000000 ) ) ;
#128594=CARTESIAN_POINT ( 'NONE',  ( 21.05000000000000426, -0.1000000000000014072, 6.477046381789850926 ) ) ;
#128607=CYLINDRICAL_SURFACE ( 'NONE', #98016, 0.09999999999999939493 ) ;
#128610=AXIS2_PLACEMENT_3D ( 'NONE', #255926, #44329, #236415 ) ;
#128613=CIRCLE ( 'NONE', #170166, 0.09999999999999939493 ) ;
#128653=DIRECTION ( 'NONE',  ( -6.938893903907210707E-14, -0.9999176327611372095, -0.01283462868039623485 ) ) ;
#128666=EDGE_CURVE ( 'NONE', #31770, #205304, #190817, .T. ) ;
#128691=CIRCLE ( 'NONE', #66133, 0.09999999999999999167 ) ;
#128695=DIRECTION ( 'NONE',  ( 1.000000000000000000, -0.000000000000000000, -0.000000000000000000 ) ) ;
#128720=CARTESIAN_POINT ( 'NONE',  ( -23.15000000000000213, -9.000000000000001776, -23.60603087734756045 ) ) ;
#128788=DIRECTION ( 'NONE',  ( 1.000000000000000000, 2.952720810173289112E-16, -0.000000000000000000 ) ) ;
#128794=ORIENTED_EDGE ( 'NONE', *, *, #90372, .F. ) ;
#128848=CIRCLE ( 'NONE', #74713, 0.4000000000000010214 ) ;
#128863=CARTESIAN_POINT ( 'NONE',  ( 20.85000000000000142, -1.835859311443637010, -45.00443916879852679 ) ) ;
#128901=FACE_OUTER_BOUND ( 'NONE', #118086, .T. ) ;
#128920=CARTESIAN_POINT ( 'NONE',  ( -23.15000000000000213, 1.999999999999998224, -13.22462192276210224 ) ) ;
#128921=CARTESIAN_POINT ( 'NONE',  ( -23.15000000000000213, 2.499999999999998668, -20.27537807723789953 ) ) ;
#128956=EDGE_CURVE ( 'NONE', #245427, #244742, #170305, .T. ) ;
#128981=EDGE_CURVE ( 'NONE', #45344, #3631, #132665, .T. ) ;
#128987=CARTESIAN_POINT ( 'NONE',  ( -21.44999999999999929, 7.150000000000000355, -21.15000000000000213 ) ) ;
#129010=VERTEX_POINT ( 'NONE', #105929 ) ;
#129023=CARTESIAN_POINT ( 'NONE',  ( -22.48660254037843487, 11.65000000000000036, 0.04999999999998249595 ) ) ;
#129041=CARTESIAN_POINT ( 'NONE',  ( 18.49999999999999645, -1.164121893241208960, -41.41484808557160591 ) ) ;
#129079=AXIS2_PLACEMENT_3D ( 'NONE', #249574, #111339, #231299 ) ;
#129090=ORIENTED_EDGE ( 'NONE', *, *, #173494, .T. ) ;
#129095=CARTESIAN_POINT ( 'NONE',  ( 23.24999999999999289, 11.65000000000000746, 11.75000000000000000 ) ) ;
#129099=FACE_OUTER_BOUND ( 'NONE', #196442, .T. ) ;
#129100=CIRCLE ( 'NONE', #170846, 3.899999999999999467 ) ;
#129125=ORIENTED_EDGE ( 'NONE', *, *, #182768, .T. ) ;
#129141=ORIENTED_EDGE ( 'NONE', *, *, #31328, .F. ) ;
#129142=CARTESIAN_POINT ( 'NONE',  ( -21.05000000000000426, -0.01771943330858751983, 6.441084688471355513 ) ) ;
#129213=DIRECTION ( 'NONE',  ( -1.000000000000000000, -2.952720810173289112E-16, 0.000000000000000000 ) ) ;
#129217=EDGE_CURVE ( 'NONE', #251180, #50839, #66199, .T. ) ;
#129245=DIRECTION ( 'NONE',  ( 0.000000000000000000, -1.000000000000000000, 8.881784197001250351E-16 ) ) ;
#129259=DIRECTION ( 'NONE',  ( 0.000000000000000000, 0.000000000000000000, -1.000000000000000000 ) ) ;
#129270=DIRECTION ( 'NONE',  ( 1.000000000000000000, 0.000000000000000000, 0.000000000000000000 ) ) ;
#129275=CARTESIAN_POINT ( 'NONE',  ( 18.59999999999997655, -4.531599869146433551E-30, -41.40000000000000568 ) ) ;
#129315=ORIENTED_EDGE ( 'NONE', *, *, #25466, .F. ) ;
#129325=ORIENTED_EDGE ( 'NONE', *, *, #242449, .T. ) ;
#129329=CARTESIAN_POINT ( 'NONE',  ( -23.15000000000000213, 4.150000000000001243, -12.35000000000000142 ) ) ;
#129336=VERTEX_POINT ( 'NONE', #148305 ) ;
#129351=ADVANCED_FACE ( 'NONE', ( #249971 ), #220341, .F. ) ;
#129367=DIRECTION ( 'NONE',  ( 0.000000000000000000, 0.000000000000000000, -1.000000000000000000 ) ) ;
#129376=DIRECTION ( 'NONE',  ( 0.000000000000000000, 0.9908441862701600211, -0.1350103645451876666 ) ) ;
#129381=EDGE_LOOP ( 'NONE', ( #154552, #21318, #32964, #153265 ) ) ;
#129397=ORIENTED_EDGE ( 'NONE', *, *, #45938, .T. ) ;
#129405=CARTESIAN_POINT ( 'NONE',  ( -20.94999999999999929, 1.835341550224413698, -11.55515129256298401 ) ) ;
#129413=ADVANCED_FACE ( 'NONE', ( #248688 ), #111743, .F. ) ;
#129429=FACE_OUTER_BOUND ( 'NONE', #195003, .T. ) ;
#129430=EDGE_CURVE ( 'NONE', #210905, #179010, #152180, .T. ) ;
#129434=EDGE_LOOP ( 'NONE', ( #207967, #154329, #176286 ) ) ;
#129453=CARTESIAN_POINT ( 'NONE',  ( 22.39999999999999858, 0.09999999999999939493, 7.790779598373383408 ) ) ;
#129454=FACE_OUTER_BOUND ( 'NONE', #231495, .T. ) ;
#129511=VERTEX_POINT ( 'NONE', #96011 ) ;
#129513=CARTESIAN_POINT ( 'NONE',  ( 21.05000000000000071, -11.74999999999999112, -2.900000000000003464 ) ) ;
#129554=ORIENTED_EDGE ( 'NONE', *, *, #1477, .T. ) ;
#129566=EDGE_LOOP ( 'NONE', ( #247016, #182474, #257942, #189129 ) ) ;
#129574=DIRECTION ( 'NONE',  ( -2.557131231893036985E-16, 0.8660254037844384856, -0.5000000000000002220 ) ) ;
#129584=ORIENTED_EDGE ( 'NONE', *, *, #169002, .T. ) ;
#129595=DIRECTION ( 'NONE',  ( 1.000000000000000000, 0.000000000000000000, 0.000000000000000000 ) ) ;
#129606=EDGE_CURVE ( 'NONE', #167418, #31326, #20612, .T. ) ;
#129620=CARTESIAN_POINT ( 'NONE',  ( -18.59999999999999787, 1.261786168565025568, -8.086498963545480478 ) ) ;
#129621=CYLINDRICAL_SURFACE ( 'NONE', #232399, 7.900000000000003908 ) ;
#129644=CARTESIAN_POINT ( 'NONE',  ( 20.85000000000000142, 11.65000000000000391, -33.50000000000000000 ) ) ;
#129714=DIRECTION ( 'NONE',  ( -1.000000000000000000, -0.000000000000000000, -0.000000000000000000 ) ) ;
#129716=ADVANCED_FACE ( 'NONE', ( #128432 ), #106273, .T. ) ;
#129746=DIRECTION ( 'NONE',  ( 0.000000000000000000, 0.000000000000000000, -1.000000000000000000 ) ) ;
#129763=EDGE_CURVE ( 'NONE', #246027, #68319, #153538, .T. ) ;
#129813=AXIS2_PLACEMENT_3D ( 'NONE', #206262, #163291, #182869 ) ;
#129821=DIRECTION ( 'NONE',  ( 0.000000000000000000, 0.000000000000000000, 1.000000000000000000 ) ) ;
#129842=CARTESIAN_POINT ( 'NONE',  ( 21.05000000000000071, 0.000000000000000000, -37.50000000000000000 ) ) ;
#129854=ORIENTED_EDGE ( 'NONE', *, *, #33485, .F. ) ;
#129871=DIRECTION ( 'NONE',  ( 0.000000000000000000, -1.000000000000000000, -0.000000000000000000 ) ) ;
#129874=ORIENTED_EDGE ( 'NONE', *, *, #182837, .T. ) ;
#129880=CIRCLE ( 'NONE', #104909, 0.09999999999999939493 ) ;
#129884=CARTESIAN_POINT ( 'NONE',  ( 21.05000000000000071, -9.500000000000000000, -23.60603087734755690 ) ) ;
#129898=ADVANCED_FACE ( 'NONE', ( #95708 ), #253500, .F. ) ;
#129924=ORIENTED_EDGE ( 'NONE', *, *, #234532, .F. ) ;
#129930=ADVANCED_FACE ( 'NONE', ( #98247 ), #33225, .T. ) ;
#129969=VERTEX_POINT ( 'NONE', #96963 ) ;
#129985=CARTESIAN_POINT ( 'NONE',  ( 19.99999999999998934, 11.65000000000000391, -21.25000000000000000 ) ) ;
#130005=DIRECTION ( 'NONE',  ( -0.000000000000000000, -0.000000000000000000, 1.000000000000000000 ) ) ;
#130010=DIRECTION ( 'NONE',  ( 0.000000000000000000, 0.000000000000000000, -1.000000000000000000 ) ) ;
#130018=ADVANCED_FACE ( 'NONE', ( #40918 ), #180404, .T. ) ;
#130021=DIRECTION ( 'NONE',  ( 1.000000000000000000, 7.304098846218133681E-16, -4.607487905232622991E-31 ) ) ;
#130036=CARTESIAN_POINT ( 'NONE',  ( -23.15000000000000213, 0.000000000000000000, -33.50000000000000000 ) ) ;
#130037=ORIENTED_EDGE ( 'NONE', *, *, #222853, .T. ) ;
#130046=CARTESIAN_POINT ( 'NONE',  ( -20.94999999999999929, -12.41227409414968541, -30.50000000000000000 ) ) ;
#130067=DIRECTION ( 'NONE',  ( 0.000000000000000000, -1.000000000000000000, -0.000000000000000000 ) ) ;
#130072=ADVANCED_FACE ( 'NONE', ( #63006 ), #236676, .T. ) ;
#130087=CARTESIAN_POINT ( 'NONE',  ( -23.25000000000000000, -1.835859311443637010, -45.00443916879852679 ) ) ;
#130092=( BOUNDED_CURVE ( )  B_SPLINE_CURVE ( 3, ( #196192, #41002, #136180, #1823 ),
 .UNSPECIFIED., .F., .F. ) 
 B_SPLINE_CURVE_WITH_KNOTS ( ( 4, 4 ),
 ( 4.712388980384689674, 6.283185307179586232 ),
 .UNSPECIFIED. ) 
 CURVE ( )  GEOMETRIC_REPRESENTATION_ITEM ( )  RATIONAL_B_SPLINE_CURVE ( ( 1.000000000000000000, 0.8047378541243649375, 0.8047378541243649375, 1.000000000000000000 ) ) 
 REPRESENTATION_ITEM ( '' )  );
#130095=EDGE_CURVE ( 'NONE', #36387, #143318, #124278, .T. ) ;
#130097=ORIENTED_EDGE ( 'NONE', *, *, #214189, .T. ) ;
#130101=ADVANCED_FACE ( 'NONE', ( #248073 ), #182734, .T. ) ;
#130122=CARTESIAN_POINT ( 'NONE',  ( -23.25000000000000000, -0.1008583690987122083, 11.74956712348939192 ) ) ;
#130142=CARTESIAN_POINT ( 'NONE',  ( 22.39999999999999503, 11.65000000000000746, -3.469446951953614189E-15 ) ) ;
#130148=AXIS2_PLACEMENT_3D ( 'NONE', #255579, #76989, #1291 ) ;
#130165=EDGE_LOOP ( 'NONE', ( #60278, #23356, #48260, #36175 ) ) ;
#130167=ORIENTED_EDGE ( 'NONE', *, *, #188960, .T. ) ;
#130195=LINE ( 'NONE', #51932, #101091 ) ;
#130203=AXIS2_PLACEMENT_3D ( 'NONE', #233946, #16210, #31920 ) ;
#130215=DIRECTION ( 'NONE',  ( 0.000000000000000000, 1.000000000000000000, 0.000000000000000000 ) ) ;
#130223=ORIENTED_EDGE ( 'NONE', *, *, #213973, .F. ) ;
#130242=ORIENTED_EDGE ( 'NONE', *, *, #82966, .T. ) ;
#130275=FACE_OUTER_BOUND ( 'NONE', #156648, .T. ) ;
#130295=AXIS2_PLACEMENT_3D ( 'NONE', #63169, #185707, #27946 ) ;
#130309=CARTESIAN_POINT ( 'NONE',  ( -22.01447462590972748, 7.263800201229918763, 0.09903700005953296193 ) ) ;
#130343=EDGE_CURVE ( 'NONE', #23701, #244468, #220320, .T. ) ;
#130345=ORIENTED_EDGE ( 'NONE', *, *, #228889, .F. ) ;
#130347=DIRECTION ( 'NONE',  ( 0.000000000000000000, 0.000000000000000000, 1.000000000000000000 ) ) ;
#130352=CARTESIAN_POINT ( 'NONE',  ( 23.24999999999999289, 6.649999999999999467, -21.35000000000000142 ) ) ;
#130356=DIRECTION ( 'NONE',  ( 1.000000000000000000, 0.000000000000000000, 0.000000000000000000 ) ) ;
#130377=EDGE_LOOP ( 'NONE', ( #135747, #79465, #135020, #45251 ) ) ;
#130407=ORIENTED_EDGE ( 'NONE', *, *, #150075, .F. ) ;
#130422=ORIENTED_EDGE ( 'NONE', *, *, #175243, .T. ) ;
#130438=DIRECTION ( 'NONE',  ( -0.000000000000000000, -1.000000000000000000, 0.000000000000000000 ) ) ;
#130439=CARTESIAN_POINT ( 'NONE',  ( -18.46856557590792747, -9.474215907786497581, -7.101986240882300017 ) ) ;
#130462=DIRECTION ( 'NONE',  ( 0.000000000000000000, -1.000000000000000000, 0.000000000000000000 ) ) ;
#130475=VERTEX_POINT ( 'NONE', #104382 ) ;
#130478=CIRCLE ( 'NONE', #196937, 0.09999999999999939493 ) ;
#130485=DIRECTION ( 'NONE',  ( 0.000000000000000000, 0.000000000000000000, -1.000000000000000000 ) ) ;
#130495=DIRECTION ( 'NONE',  ( 0.000000000000000000, 0.9908441862701596881, -0.1350103645451904977 ) ) ;
#130496=VERTEX_POINT ( 'NONE', #243911 ) ;
#130519=AXIS2_PLACEMENT_3D ( 'NONE', #53341, #156328, #36374 ) ;
#130557=EDGE_LOOP ( 'NONE', ( #207881, #22302, #46410, #215626 ) ) ;
#130566=AXIS2_PLACEMENT_3D ( 'NONE', #60925, #217422, #63489 ) ;
#130602=EDGE_CURVE ( 'NONE', #172993, #101735, #116455, .T. ) ;
#130630=EDGE_CURVE ( 'NONE', #227113, #36387, #175968, .T. ) ;
#130649=ORIENTED_EDGE ( 'NONE', *, *, #183333, .T. ) ;
#130723=DIRECTION ( 'NONE',  ( -0.000000000000000000, -0.9876197685951252359, -0.1568667991644863424 ) ) ;
#130735=VERTEX_POINT ( 'NONE', #91279 ) ;
#130740=CARTESIAN_POINT ( 'NONE',  ( 20.94999999999999929, 0.000000000000000000, 0.000000000000000000 ) ) ;
#130745=EDGE_CURVE ( 'NONE', #253599, #111006, #178835, .T. ) ;
#130782=CARTESIAN_POINT ( 'NONE',  ( -20.54999999999999716, 4.250000000000000000, -12.25000000000000000 ) ) ;
#130796=EDGE_CURVE ( 'NONE', #84065, #197300, #198064, .T. ) ;
#130828=TOROIDAL_SURFACE ( 'NONE', #164158, 0.2000000000000000111, 0.1000000000000000056 ) ;
#130833=ORIENTED_EDGE ( 'NONE', *, *, #224414, .T. ) ;
#130849=ORIENTED_EDGE ( 'NONE', *, *, #20543, .T. ) ;
#130853=EDGE_CURVE ( 'NONE', #57106, #111888, #8113, .T. ) ;
#130937=FACE_OUTER_BOUND ( 'NONE', #135954, .T. ) ;
#130945=CARTESIAN_POINT ( 'NONE',  ( -18.39999999999999858, -9.600000000000004974, -40.10018939122204529 ) ) ;
#130975=DIRECTION ( 'NONE',  ( 1.000000000000000000, 2.952720810173289112E-16, -0.000000000000000000 ) ) ;
#130978=ORIENTED_EDGE ( 'NONE', *, *, #124441, .T. ) ;
#130979=LINE ( 'NONE', #210520, #103116 ) ;
#130993=EDGE_CURVE ( 'NONE', #209903, #141605, #20790, .T. ) ;
#131000=CARTESIAN_POINT ( 'NONE',  ( 18.59999999999999787, -11.74999999999999289, -24.85000000000000142 ) ) ;
#131006=ORIENTED_EDGE ( 'NONE', *, *, #163953, .T. ) ;
#131026=ORIENTED_EDGE ( 'NONE', *, *, #139811, .T. ) ;
#131027=FACE_OUTER_BOUND ( 'NONE', #22999, .T. ) ;
#131049=EDGE_CURVE ( 'NONE', #29639, #206018, #258046, .T. ) ;
#131094=DIRECTION ( 'NONE',  ( 1.000000000000000000, -0.000000000000000000, -0.000000000000000000 ) ) ;
#131107=CARTESIAN_POINT ( 'NONE',  ( 20.90851465518106167, 10.32532329026770590, -39.06993430183595706 ) ) ;
#131123=EDGE_CURVE ( 'NONE', #13885, #191690, #244091, .T. ) ;
#131145=DIRECTION ( 'NONE',  ( 0.000000000000000000, 0.000000000000000000, -1.000000000000000000 ) ) ;
#131147=DIRECTION ( 'NONE',  ( 0.000000000000000000, -0.6728971962616697722, 0.7397360091702875895 ) ) ;
#131148=VERTEX_POINT ( 'NONE', #179184 ) ;
#131163=EDGE_CURVE ( 'NONE', #8515, #109777, #22674, .T. ) ;
#131170=ORIENTED_EDGE ( 'NONE', *, *, #185900, .T. ) ;
#131175=ORIENTED_EDGE ( 'NONE', *, *, #38248, .F. ) ;
#131210=VECTOR ( 'NONE', #39083, 1000.000000000000000 ) ;
#131217=EDGE_CURVE ( 'NONE', #129010, #209135, #145143, .T. ) ;
#131224=EDGE_CURVE ( 'NONE', #23701, #255533, #64349, .T. ) ;
#131230=VECTOR ( 'NONE', #50050, 1000.000000000000000 ) ;
#131234=LINE ( 'NONE', #89529, #248147 ) ;
#131242=EDGE_CURVE ( 'NONE', #205304, #111888, #169914, .T. ) ;
#131304=EDGE_CURVE ( 'NONE', #207105, #198340, #175116, .T. ) ;
#131331=CARTESIAN_POINT ( 'NONE',  ( 20.84999999999999787, 11.75000000000000355, -26.58085275404129888 ) ) ;
#131365=DIRECTION ( 'NONE',  ( 0.000000000000000000, -0.8700118002898321601, 0.4930308989875230030 ) ) ;
#131399=DIRECTION ( 'NONE',  ( 0.000000000000000000, -1.000000000000000000, 0.000000000000000000 ) ) ;
#131436=AXIS2_PLACEMENT_3D ( 'NONE', #98514, #62021, #155997 ) ;
#131471=DIRECTION ( 'NONE',  ( 0.000000000000000000, 0.000000000000000000, 1.000000000000000000 ) ) ;
#131481=ORIENTED_EDGE ( 'NONE', *, *, #213156, .F. ) ;
#131482=CARTESIAN_POINT ( 'NONE',  ( -18.36527282682040507, -9.500000599999188111, -40.42214896449912942 ) ) ;
#131508=CARTESIAN_POINT ( 'NONE',  ( 23.14999999999999858, 0.000000000000000000, 0.000000000000000000 ) ) ;
#131513=LINE ( 'NONE', #94943, #20578 ) ;
#131545=EDGE_CURVE ( 'NONE', #31765, #185054, #83454, .T. ) ;
#131546=CARTESIAN_POINT ( 'NONE',  ( 18.59999996954842771, -9.523204137858824581, -40.38304171191644087 ) ) ;
#131565=EDGE_LOOP ( 'NONE', ( #27149, #49863, #70524, #150680 ) ) ;
#131602=ADVANCED_FACE ( 'NONE', ( #19797 ), #133378, .T. ) ;
#131617=FACE_OUTER_BOUND ( 'NONE', #108465, .T. ) ;
#131644=VERTEX_POINT ( 'NONE', #182725 ) ;
#131645=AXIS2_PLACEMENT_3D ( 'NONE', #187294, #11215, #131147 ) ;
#131652=CARTESIAN_POINT ( 'NONE',  ( -21.05000000000000071, 0.000000000000000000, -33.50000000000000000 ) ) ;
#131655=DIRECTION ( 'NONE',  ( -0.000000000000000000, 0.000000000000000000, 1.000000000000000000 ) ) ;
#131664=( BOUNDED_CURVE ( )  B_SPLINE_CURVE ( 3, ( #233027, #131331, #213430, #34832 ),
 .UNSPECIFIED., .F., .F. ) 
 B_SPLINE_CURVE_WITH_KNOTS ( ( 4, 4 ),
 ( 4.712388980384690562, 6.283185307179586232 ),
 .UNSPECIFIED. ) 
 CURVE ( )  GEOMETRIC_REPRESENTATION_ITEM ( )  RATIONAL_B_SPLINE_CURVE ( ( 1.000000000000000000, 0.8047378541243652705, 0.8047378541243652705, 1.000000000000000000 ) ) 
 REPRESENTATION_ITEM ( '' )  );
#131687=AXIS2_PLACEMENT_3D ( 'NONE', #10988, #133503, #76093 ) ;
#131695=CARTESIAN_POINT ( 'NONE',  ( 22.49436431346199683, 0.06690352972226094874, 11.64995094765345840 ) ) ;
#131706=CARTESIAN_POINT ( 'NONE',  ( -21.05000000000000071, -0.09999996530009948315, 6.477552182493442778 ) ) ;
#131758=ADVANCED_FACE ( 'NONE', ( #5318 ), #199459, .T. ) ;
#131772=ADVANCED_FACE ( 'NONE', ( #255465 ), #191728, .T. ) ;
#131773=AXIS2_PLACEMENT_3D ( 'NONE', #55355, #73707, #115365 ) ;
#131800=ORIENTED_EDGE ( 'NONE', *, *, #165431, .T. ) ;
#131816=EDGE_CURVE ( 'NONE', #79663, #140018, #96123, .T. ) ;
#131861=AXIS2_PLACEMENT_3D ( 'NONE', #228469, #104613, #245463 ) ;
#131877=DIRECTION ( 'NONE',  ( 0.000000000000000000, 1.000000000000000000, 0.000000000000000000 ) ) ;
#131881=DIRECTION ( 'NONE',  ( 1.000000000000000000, -0.000000000000000000, 0.000000000000000000 ) ) ;
#131905=AXIS2_PLACEMENT_3D ( 'NONE', #116358, #195899, #17257 ) ;
#131906=AXIS2_PLACEMENT_3D ( 'NONE', #121785, #5639, #180460 ) ;
#131942=ORIENTED_EDGE ( 'NONE', *, *, #207887, .T. ) ;
#131955=AXIS2_PLACEMENT_3D ( 'NONE', #132736, #177012, #135266 ) ;
#131962=ORIENTED_EDGE ( 'NONE', *, *, #124201, .F. ) ;
#131969=ORIENTED_EDGE ( 'NONE', *, *, #156283, .F. ) ;
#132018=CARTESIAN_POINT ( 'NONE',  ( 21.05000000000000071, -11.29603075033528192, -30.45210084033612929 ) ) ;
#132063=EDGE_CURVE ( 'NONE', #44319, #63693, #196103, .T. ) ;
#132099=ADVANCED_FACE ( 'NONE', ( #166723 ), #187562, .F. ) ;
#132137=ORIENTED_EDGE ( 'NONE', *, *, #162712, .T. ) ;
#132158=ORIENTED_EDGE ( 'NONE', *, *, #243323, .T. ) ;
#132229=ORIENTED_EDGE ( 'NONE', *, *, #242926, .T. ) ;
#132237=ORIENTED_EDGE ( 'NONE', *, *, #44138, .T. ) ;
#132254=ORIENTED_EDGE ( 'NONE', *, *, #211364, .T. ) ;
#132259=DIRECTION ( 'NONE',  ( 1.000000000000000000, 0.000000000000000000, 0.000000000000000000 ) ) ;
#132261=ORIENTED_EDGE ( 'NONE', *, *, #108995, .F. ) ;
#132262=ORIENTED_EDGE ( 'NONE', *, *, #160971, .F. ) ;
#132331=FACE_OUTER_BOUND ( 'NONE', #143798, .T. ) ;
#132406=DIRECTION ( 'NONE',  ( 1.000000000000000000, 0.000000000000000000, 0.000000000000000000 ) ) ;
#132420=DIRECTION ( 'NONE',  ( 1.000000000000000000, -0.000000000000000000, -0.000000000000000000 ) ) ;
#132423=DIRECTION ( 'NONE',  ( 1.000000000000000000, 0.000000000000000000, 0.000000000000000000 ) ) ;
#132429=ORIENTED_EDGE ( 'NONE', *, *, #213042, .T. ) ;
#132452=DIRECTION ( 'NONE',  ( 0.000000000000000000, 1.000000000000000000, 0.000000000000000000 ) ) ;
#132495=LINE ( 'NONE', #69976, #199694 ) ;
#132497=CARTESIAN_POINT ( 'NONE',  ( -23.25000000000000000, 0.000000000000000000, -4.049999999999998934 ) ) ;
#132513=CARTESIAN_POINT ( 'NONE',  ( -23.15000000000000213, 1.999999999999998224, -13.22462192276210224 ) ) ;
#132514=ORIENTED_EDGE ( 'NONE', *, *, #63148, .F. ) ;
#132530=CARTESIAN_POINT ( 'NONE',  ( -21.05000000000000071, -11.64999999999999858, -30.50000000000000000 ) ) ;
#132540=ORIENTED_EDGE ( 'NONE', *, *, #147895, .T. ) ;
#132561=VERTEX_POINT ( 'NONE', #40797 ) ;
#132583=ORIENTED_EDGE ( 'NONE', *, *, #192364, .T. ) ;
#132602=CARTESIAN_POINT ( 'NONE',  ( -23.25000000000000000, 0.000000000000000000, -33.50000000000000000 ) ) ;
#132607=DIRECTION ( 'NONE',  ( 1.000000000000000000, -0.000000000000000000, -0.000000000000000000 ) ) ;
#132613=ORIENTED_EDGE ( 'NONE', *, *, #9599, .F. ) ;
#132619=EDGE_LOOP ( 'NONE', ( #195792, #72275, #58107, #25232 ) ) ;
#132639=DIRECTION ( 'NONE',  ( 0.000000000000000000, 0.000000000000000000, -1.000000000000000000 ) ) ;
#132647=AXIS2_PLACEMENT_3D ( 'NONE', #205074, #9460, #245518 ) ;
#132654=EDGE_LOOP ( 'NONE', ( #133205, #220702, #252984, #147935 ) ) ;
#132655=CARTESIAN_POINT ( 'NONE',  ( 21.04999999999999716, 8.871279685995645536, -8.558628995140946216 ) ) ;
#132660=ORIENTED_EDGE ( 'NONE', *, *, #154771, .F. ) ;
#132665=CIRCLE ( 'NONE', #20239, 0.4000000000000010214 ) ;
#132682=CARTESIAN_POINT ( 'NONE',  ( 21.05000000000000071, 8.776282895292474961, -12.15000000000000036 ) ) ;
#132703=CARTESIAN_POINT ( 'NONE',  ( 18.59999999999999076, 11.65000000000000391, -24.85000000000000142 ) ) ;
#132716=ADVANCED_FACE ( 'NONE', ( #66755 ), #63174, .F. ) ;
#132735=DIRECTION ( 'NONE',  ( 0.000000000000000000, 1.734723475976817507E-14, 1.000000000000000000 ) ) ;
#132736=CARTESIAN_POINT ( 'NONE',  ( -20.64999999999999858, 7.150000000000000355, -12.34999999999999964 ) ) ;
#132742=DIRECTION ( 'NONE',  ( 1.000000000000000000, 0.000000000000000000, 0.000000000000000000 ) ) ;
#132755=DIRECTION ( 'NONE',  ( 0.000000000000000000, 0.000000000000000000, -1.000000000000000000 ) ) ;
#132763=ORIENTED_EDGE ( 'NONE', *, *, #56439, .F. ) ;
#132790=DIRECTION ( 'NONE',  ( 0.000000000000000000, 1.000000000000000000, 0.000000000000000000 ) ) ;
#132791=CARTESIAN_POINT ( 'NONE',  ( -20.94999999999999929, 0.000000000000000000, -33.50000000000000000 ) ) ;
#132828=FACE_OUTER_BOUND ( 'NONE', #212983, .T. ) ;
#132868=AXIS2_PLACEMENT_3D ( 'NONE', #106000, #222091, #242960 ) ;
#132933=EDGE_LOOP ( 'NONE', ( #232048, #233976, #241991, #21440 ) ) ;
#132949=DIRECTION ( 'NONE',  ( 4.239556034732056743E-17, -0.1298341882520022972, -0.9915357197604853789 ) ) ;
#132964=CARTESIAN_POINT ( 'NONE',  ( -23.15000000000000213, 2.600000000000000089, -13.22462192276210224 ) ) ;
#132989=CYLINDRICAL_SURFACE ( 'NONE', #219021, 11.79999999999999716 ) ;
#132991=VECTOR ( 'NONE', #31534, 1000.000000000000000 ) ;
#132994=ORIENTED_EDGE ( 'NONE', *, *, #207502, .F. ) ;
#132996=CARTESIAN_POINT ( 'NONE',  ( 22.42196299218230493, 0.002441673987300593818, 11.64961170264947121 ) ) ;
#132999=CARTESIAN_POINT ( 'NONE',  ( 22.39999999999999503, 7.790779598373379855, 0.000000000000000000 ) ) ;
#133025=DIRECTION ( 'NONE',  ( 1.000000000000000000, -0.000000000000000000, -0.000000000000000000 ) ) ;
#133049=CARTESIAN_POINT ( 'NONE',  ( -21.05000000000000071, 0.000000000000000000, 0.000000000000000000 ) ) ;
#133096=CARTESIAN_POINT ( 'NONE',  ( 18.49999999999999645, -1.866714910057309273, -11.75267524628200633 ) ) ;
#133111=CARTESIAN_POINT ( 'NONE',  ( 19.75857864376268935, 11.65000000000000391, -24.75000000000000000 ) ) ;
#133121=DIRECTION ( 'NONE',  ( 1.000000000000000000, 0.000000000000000000, 0.000000000000000000 ) ) ;
#133122=ORIENTED_EDGE ( 'NONE', *, *, #189274, .T. ) ;
#133137=ORIENTED_EDGE ( 'NONE', *, *, #79651, .F. ) ;
#133149=VECTOR ( 'NONE', #251073, 1000.000000000000000 ) ;
#133171=EDGE_CURVE ( 'NONE', #256381, #172386, #50875, .T. ) ;
#133172=( BOUNDED_SURFACE ( )  B_SPLINE_SURFACE ( 3, 2, ( 
 ( #17945, #162613, #177058 ),
 ( #83025, #157510, #58337 ),
 ( #80452, #178341, #57055 ),
 ( #137881, #136602, #79194 ),
 ( #139156, #160061, #119640 ),
 ( #140457, #37536, #199163 ) ),
 .UNSPECIFIED., .F., .F., .F. ) 
 B_SPLINE_SURFACE_WITH_KNOTS ( ( 4, 2, 4 ),
 ( 3, 3 ),
 ( 0.0001792624049599592486, 0.0003686986002124714528, 0.0005581347954649836570 ),
 ( 0.000000000000000000, 1.000000000000000000 ),
 .UNSPECIFIED. ) 
 GEOMETRIC_REPRESENTATION_ITEM ( )  RATIONAL_B_SPLINE_SURFACE ( (
 ( 1.000000000000000000, 0.9238795325112837409, 1.000000000000000000),
 ( 1.000000000000000000, 0.9229318695238861725, 1.000000000000000000),
 ( 1.000000000000000000, 0.8926288119230176843, 1.000000000000000000),
 ( 1.000000000000000000, 0.8123777807271899132, 1.000000000000000000),
 ( 1.000000000000000000, 0.7629087100931073451, 1.000000000000000000),
 ( 1.000000000000000000, 0.7071067811865475727, 1.000000000000000000) ) ) 
 REPRESENTATION_ITEM ( '' )  SURFACE ( )  );
#133205=ORIENTED_EDGE ( 'NONE', *, *, #235110, .F. ) ;
#133263=ORIENTED_EDGE ( 'NONE', *, *, #22087, .T. ) ;
#133272=CARTESIAN_POINT ( 'NONE',  ( 21.00000000000000000, 9.749999999999998224, -21.15000000000000213 ) ) ;
#133284=ORIENTED_EDGE ( 'NONE', *, *, #161247, .F. ) ;
#133338=ORIENTED_EDGE ( 'NONE', *, *, #107381, .F. ) ;
#133349=CARTESIAN_POINT ( 'NONE',  ( -20.54999999999999716, 0.000000000000000000, -33.50000000000000000 ) ) ;
#133378=TOROIDAL_SURFACE ( 'NONE', #71036, 11.65000000000000036, 0.1000000000000000056 ) ;
#133389=DIRECTION ( 'NONE',  ( -1.000000000000000000, -0.000000000000000000, -0.000000000000000000 ) ) ;
#133457=CIRCLE ( 'NONE', #21063, 12.87499999999999822 ) ;
#133463=VERTEX_POINT ( 'NONE', #225169 ) ;
#133493=VECTOR ( 'NONE', #25913, 1000.000000000000000 ) ;
#133503=DIRECTION ( 'NONE',  ( 0.000000000000000000, -0.9893560106964500722, 0.1455152366551550613 ) ) ;
#133505=CIRCLE ( 'NONE', #21114, 0.1000000000000028644 ) ;
#133512=ORIENTED_EDGE ( 'NONE', *, *, #160758, .F. ) ;
#133530=CARTESIAN_POINT ( 'NONE',  ( -23.25000000000000000, 5.950000000000010836, -23.19429769496518645 ) ) ;
#133549=CARTESIAN_POINT ( 'NONE',  ( -20.85000000000000142, 0.000000000000000000, -33.50000000000000000 ) ) ;
#133556=CARTESIAN_POINT ( 'NONE',  ( -20.64999999999999858, 1.925233644859816629, -12.73024353312613144 ) ) ;
#133562=CARTESIAN_POINT ( 'NONE',  ( 20.04142135623730070, 11.65000000000000391, -21.35000000000000142 ) ) ;
#133564=DIRECTION ( 'NONE',  ( 0.000000000000000000, 1.000000000000000000, 0.000000000000000000 ) ) ;
#133583=( LENGTH_UNIT ( ) NAMED_UNIT ( * ) SI_UNIT ( .MILLI., .METRE. ) );
#133585=EDGE_CURVE ( 'NONE', #67142, #122573, #251157, .T. ) ;
#133592=CARTESIAN_POINT ( 'NONE',  ( -20.15000000000000568, 9.291421356237307805, -21.25000000000000000 ) ) ;
#133615=CARTESIAN_POINT ( 'NONE',  ( 23.15000000000000213, -11.74999999999999289, -21.35000000000000142 ) ) ;
#133616=ADVANCED_FACE ( 'NONE', ( #210767 ), #191237, .T. ) ;
#133652=CARTESIAN_POINT ( 'NONE',  ( 21.05000000000000071, 0.000000000000000000, -33.50000000000000000 ) ) ;
#133656=AXIS2_PLACEMENT_3D ( 'NONE', #222703, #49215, #24548 ) ;
#133679=EDGE_LOOP ( 'NONE', ( #247162, #196061, #243658, #92252 ) ) ;
#133697=CIRCLE ( 'NONE', #137774, 0.09999999999999992228 ) ;
#133707=CARTESIAN_POINT ( 'NONE',  ( -18.59999999999999787, 5.949999999999945111, -10.30570230503485796 ) ) ;
#133720=CARTESIAN_POINT ( 'NONE',  ( -22.49231231312463208, 11.64998490367728223, 0.06105288760136910742 ) ) ;
#133736=CARTESIAN_POINT ( 'NONE',  ( -20.64999999999999858, 1.999999999999998224, -13.22462192276210224 ) ) ;
#133753=AXIS2_PLACEMENT_3D ( 'NONE', #179920, #1240, #44251 ) ;
#133754=CARTESIAN_POINT ( 'NONE',  ( -18.50000000000000000, 5.341242989991647150, 9.806650206488024324 ) ) ;
#133791=ORIENTED_EDGE ( 'NONE', *, *, #147130, .T. ) ;
#133798=FACE_OUTER_BOUND ( 'NONE', #5828, .T. ) ;
#133804=VERTEX_POINT ( 'NONE', #26386 ) ;
#133819=CARTESIAN_POINT ( 'NONE',  ( 21.53699400384692808, 3.391009845873812292E-12, 6.787711793240010394 ) ) ;
#133841=FACE_OUTER_BOUND ( 'NONE', #179008, .T. ) ;
#133871=CARTESIAN_POINT ( 'NONE',  ( 20.85000000000000142, -1.749999999999999778, -45.11895003862225195 ) ) ;
#133874=CARTESIAN_POINT ( 'NONE',  ( -22.57320508075687115, 11.75000000000000000, 0.000000000000000000 ) ) ;
#133895=ORIENTED_EDGE ( 'NONE', *, *, #176869, .T. ) ;
#133903=ORIENTED_EDGE ( 'NONE', *, *, #211216, .T. ) ;
#133919=ORIENTED_EDGE ( 'NONE', *, *, #82329, .F. ) ;
#133950=ORIENTED_EDGE ( 'NONE', *, *, #10553, .F. ) ;
#133981=DIRECTION ( 'NONE',  ( -0.000000000000000000, -1.265107689135680095E-16, 1.000000000000000000 ) ) ;
#133998=CARTESIAN_POINT ( 'NONE',  ( -20.64999999999999858, 1.999999999999998224, -13.22462192276210224 ) ) ;
#134002=AXIS2_PLACEMENT_3D ( 'NONE', #172227, #32714, #147478 ) ;
#134003=DIRECTION ( 'NONE',  ( 0.000000000000000000, -0.9908441862701600211, 0.1350103645451876944 ) ) ;
#134017=DIRECTION ( 'NONE',  ( 2.952720810173289112E-16, -1.000000000000000000, 0.000000000000000000 ) ) ;
#134023=DIRECTION ( 'NONE',  ( 0.000000000000000000, 0.000000000000000000, -1.000000000000000000 ) ) ;
#134024=DIRECTION ( 'NONE',  ( 4.504528286903032433E-15, -0.1298341882520124002, -0.9915357197604841577 ) ) ;
#134025=CARTESIAN_POINT ( 'NONE',  ( 21.05000000000000071, -1.162701749938009677, -7.900000000000000355 ) ) ;
#134039=DIRECTION ( 'NONE',  ( -6.938893903907222067E-15, 1.000000000000000000, 2.891205793294679805E-16 ) ) ;
#134088=ADVANCED_FACE ( 'NONE', ( #137030 ), #200856, .F. ) ;
#134096=ORIENTED_EDGE ( 'NONE', *, *, #98448, .T. ) ;
#134097=CARTESIAN_POINT ( 'NONE',  ( 18.39999999999999858, -9.500000000000000000, -40.10018939122205239 ) ) ;
#134192=DIRECTION ( 'NONE',  ( -1.000000000000000000, 0.000000000000000000, -1.734723475976817507E-14 ) ) ;
#134194=AXIS2_PLACEMENT_3D ( 'NONE', #86121, #9185, #147415 ) ;
#134196=ORIENTED_EDGE ( 'NONE', *, *, #43999, .F. ) ;
#134197=ORIENTED_EDGE ( 'NONE', *, *, #153156, .T. ) ;
#134239=EDGE_CURVE ( 'NONE', #31326, #117566, #38994, .T. ) ;
#134244=CARTESIAN_POINT ( 'NONE',  ( 22.46250603428203618, 0.02114417613880632471, 11.64986309734008074 ) ) ;
#134263=CYLINDRICAL_SURFACE ( 'NONE', #211349, 0.09999999999999939493 ) ;
#134276=EDGE_CURVE ( 'NONE', #106654, #251285, #138881, .T. ) ;
#134318=TOROIDAL_SURFACE ( 'NONE', #26023, 0.2000000000000000111, 0.1000000000000000056 ) ;
#134385=EDGE_CURVE ( 'NONE', #190309, #57548, #113430, .T. ) ;
#134448=AXIS2_PLACEMENT_3D ( 'NONE', #110649, #70274, #11569 ) ;
#134478=AXIS2_PLACEMENT_3D ( 'NONE', #95418, #175006, #215358 ) ;
#134483=EDGE_CURVE ( 'NONE', #38660, #54887, #119741, .T. ) ;
#134503=ORIENTED_EDGE ( 'NONE', *, *, #15609, .T. ) ;
#134518=AXIS2_PLACEMENT_3D ( 'NONE', #128230, #89089, #167379 ) ;
#134519=DIRECTION ( 'NONE',  ( 0.000000000000000000, -0.000000000000000000, -1.000000000000000000 ) ) ;
#134530=DIRECTION ( 'NONE',  ( 0.000000000000000000, 0.000000000000000000, 1.000000000000000000 ) ) ;
#134546=CARTESIAN_POINT ( 'NONE',  ( 18.59999999999999076, -1.835859311443637010, -45.00443916879852679 ) ) ;
#134600=ORIENTED_EDGE ( 'NONE', *, *, #146748, .T. ) ;
#134601=CARTESIAN_POINT ( 'NONE',  ( -20.64999999999999858, -9.000000000000003553, -9.893969122652444881 ) ) ;
#134675=CYLINDRICAL_SURFACE ( 'NONE', #54070, 0.09999999999999939493 ) ;
#134679=CIRCLE ( 'NONE', #34967, 0.1000000000000028644 ) ;
#134691=ADVANCED_FACE ( 'NONE', ( #2323 ), #96821, .T. ) ;
#134705=CIRCLE ( 'NONE', #126534, 12.87499999999999822 ) ;
#134729=LINE ( 'NONE', #229997, #24393 ) ;
#134759=EDGE_CURVE ( 'NONE', #31326, #144794, #220448, .T. ) ;
#134782=CARTESIAN_POINT ( 'NONE',  ( 21.05000000000000071, 8.826429739517195117, -8.414054712943700665 ) ) ;
#134787=DIRECTION ( 'NONE',  ( -1.000000000000000000, 0.000000000000000000, -0.000000000000000000 ) ) ;
#134788=AXIS2_PLACEMENT_3D ( 'NONE', #190054, #184912, #85773 ) ;
#134791=CARTESIAN_POINT ( 'NONE',  ( 18.49999999999999645, -1.299733671230788756, 9.971870477130599042 ) ) ;
#134856=DIRECTION ( 'NONE',  ( 1.000000000000000000, -0.000000000000000000, -0.000000000000000000 ) ) ;
#134881=EDGE_CURVE ( 'NONE', #75563, #67142, #51214, .T. ) ;
#134900=DIRECTION ( 'NONE',  ( 0.000000000000000000, 0.000000000000000000, -1.000000000000000000 ) ) ;
#134921=DIRECTION ( 'NONE',  ( 0.000000000000000000, 0.000000000000000000, -1.000000000000000000 ) ) ;
#134935=CARTESIAN_POINT ( 'NONE',  ( 18.59999999999999787, 0.000000000000000000, 0.000000000000000000 ) ) ;
#134948=SPHERICAL_SURFACE ( 'NONE', #17093, 0.1000000000000000056 ) ;
#134956=VERTEX_POINT ( 'NONE', #20330 ) ;
#135020=ORIENTED_EDGE ( 'NONE', *, *, #34414, .F. ) ;
#135045=EDGE_CURVE ( 'NONE', #44809, #50852, #151214, .T. ) ;
#135067=CYLINDRICAL_SURFACE ( 'NONE', #219098, 0.09999999999999939493 ) ;
#135073=DIRECTION ( 'NONE',  ( 1.000000000000000000, -0.000000000000000000, -0.000000000000000000 ) ) ;
#135107=DIRECTION ( 'NONE',  ( 1.000000000000000000, -0.000000000000000000, -0.000000000000000000 ) ) ;
#135126=VECTOR ( 'NONE', #145286, 1000.000000000000000 ) ;
#135142=DIRECTION ( 'NONE',  ( -1.000000000000000000, -1.836970198721029934E-16, -0.000000000000000000 ) ) ;
#135150=ORIENTED_EDGE ( 'NONE', *, *, #71153, .F. ) ;
#135160=DIRECTION ( 'NONE',  ( 0.000000000000000000, 0.000000000000000000, 1.000000000000000000 ) ) ;
#135174=DIRECTION ( 'NONE',  ( 0.000000000000000000, 0.000000000000000000, -1.000000000000000000 ) ) ;
#135192=VERTEX_POINT ( 'NONE', #210510 ) ;
#135213=DIRECTION ( 'NONE',  ( 0.000000000000000000, 0.000000000000000000, -1.000000000000000000 ) ) ;
#135220=CARTESIAN_POINT ( 'NONE',  ( -20.64999999999999858, 0.000000000000000000, -31.50000000000000000 ) ) ;
#135230=AXIS2_PLACEMENT_3D ( 'NONE', #242961, #206415, #246815 ) ;
#135232=CARTESIAN_POINT ( 'NONE',  ( 20.84999999999999432, -1.164121893241208960, -41.41484808557160591 ) ) ;
#135260=VERTEX_POINT ( 'NONE', #172715 ) ;
#135266=DIRECTION ( 'NONE',  ( 0.000000000000000000, 0.000000000000000000, 1.000000000000000000 ) ) ;
#135273=CYLINDRICAL_SURFACE ( 'NONE', #24140, 0.1000000000000000194 ) ;
#135276=ORIENTED_EDGE ( 'NONE', *, *, #247429, .T. ) ;
#135325=EDGE_CURVE ( 'NONE', #146767, #157290, #67995, .T. ) ;
#135338=LINE ( 'NONE', #238296, #108302 ) ;
#135354=CARTESIAN_POINT ( 'NONE',  ( -21.05000000000000071, 6.413759733810282526, -0.08561306080396846596 ) ) ;
#135355=DIRECTION ( 'NONE',  ( 2.557131231893037478E-16, -0.8660254037844385966, 0.5000000000000003331 ) ) ;
#135378=CARTESIAN_POINT ( 'NONE',  ( 18.43466021071414573, -9.494190690456539627, -40.11706156012773050 ) ) ;
#135403=EDGE_CURVE ( 'NONE', #95630, #57548, #164665, .T. ) ;
#135468=ORIENTED_EDGE ( 'NONE', *, *, #193367, .F. ) ;
#135482=CARTESIAN_POINT ( 'NONE',  ( 18.59999999999999076, 7.070967871798842452, -37.24656422186831151 ) ) ;
#135486=FACE_OUTER_BOUND ( 'NONE', #176517, .T. ) ;
#135501=ORIENTED_EDGE ( 'NONE', *, *, #147895, .F. ) ;
#135526=DIRECTION ( 'NONE',  ( -1.000000000000000000, -0.000000000000000000, -0.000000000000000000 ) ) ;
#135532=DIRECTION ( 'NONE',  ( 0.000000000000000000, 0.000000000000000000, -1.000000000000000000 ) ) ;
#135534=CIRCLE ( 'NONE', #248163, 0.09999999999999982514 ) ;
#135560=CARTESIAN_POINT ( 'NONE',  ( -22.46246831459151494, 0.02191216693942996119, 11.64986456120996650 ) ) ;
#135581=CARTESIAN_POINT ( 'NONE',  ( 18.49999999999999289, 10.49142135623730709, -24.74999999999999645 ) ) ;
#135604=DIRECTION ( 'NONE',  ( 0.000000000000000000, -1.000000000000000000, 0.000000000000000000 ) ) ;
#135613=FACE_OUTER_BOUND ( 'NONE', #121740, .T. ) ;
#135614=DIRECTION ( 'NONE',  ( -1.000000000000000000, -0.000000000000000000, -0.000000000000000000 ) ) ;
#135635=ADVANCED_FACE ( 'NONE', ( #13291 ), #22413, .T. ) ;
#135636=DIRECTION ( 'NONE',  ( 1.000000000000000000, 0.000000000000000000, 0.000000000000000000 ) ) ;
#135641=ORIENTED_EDGE ( 'NONE', *, *, #77192, .F. ) ;
#135663=CARTESIAN_POINT ( 'NONE',  ( -21.05000000000000071, 5.265981236333565222E-16, 4.299999999999956302 ) ) ;
#135705=CARTESIAN_POINT ( 'NONE',  ( 18.59999999999999076, 0.000000000000000000, -33.50000000000000000 ) ) ;
#135723=CARTESIAN_POINT ( 'NONE',  ( 20.95462737510932882, 10.55678195164374067, -7.569950056562293916 ) ) ;
#135744=EDGE_CURVE ( 'NONE', #184180, #79953, #145727, .T. ) ;
#135747=ORIENTED_EDGE ( 'NONE', *, *, #34380, .F. ) ;
#135823=CARTESIAN_POINT ( 'NONE',  ( -23.25000000000000000, 0.000000000000000000, -37.40000000000000568 ) ) ;
#135835=DIRECTION ( 'NONE',  ( 2.879366945564059217E-14, -0.9875055080513751582, 0.1575844902526747915 ) ) ;
#135838=DIRECTION ( 'NONE',  ( 2.952720810173288619E-16, -1.000000000000000000, 0.000000000000000000 ) ) ;
#135862=VECTOR ( 'NONE', #233476, 1000.000000000000000 ) ;
#135870=DIRECTION ( 'NONE',  ( 0.000000000000000000, -1.000000000000000000, 0.000000000000000000 ) ) ;
#135883=DIRECTION ( 'NONE',  ( 0.000000000000000000, 0.000000000000000000, -1.000000000000000000 ) ) ;
#135909=DIRECTION ( 'NONE',  ( 0.000000000000000000, -1.000000000000000000, 0.000000000000000000 ) ) ;
#135936=CARTESIAN_POINT ( 'NONE',  ( -23.25000000000000000, 0.000000000000000000, -33.50000000000000000 ) ) ;
#135953=B_SPLINE_CURVE_WITH_KNOTS ( 'NONE', 3,
 ( #44474, #124010, #104403, #164415, #13062, #250364, #132999 ),
 .UNSPECIFIED., .F., .F.,
 ( 4, 3, 4 ),
 ( 0.000000000000000000, 0.0007844235214594269838, 0.001767853679404345069 ),
 .UNSPECIFIED. ) ;
#135954=EDGE_LOOP ( 'NONE', ( #101738, #13282, #256788, #167566 ) ) ;
#135969=EDGE_LOOP ( 'NONE', ( #97338, #20120, #31746, #84716 ) ) ;
#136010=DIRECTION ( 'NONE',  ( 0.000000000000000000, 0.000000000000000000, -1.000000000000000000 ) ) ;
#136017=VECTOR ( 'NONE', #189712, 1000.000000000000000 ) ;
#136030=AXIS2_PLACEMENT_3D ( 'NONE', #109519, #189072, #89957 ) ;
#136087=CARTESIAN_POINT ( 'NONE',  ( -23.15000000000000213, 2.500000000000000444, -13.22462192276210224 ) ) ;
#136099=CARTESIAN_POINT ( 'NONE',  ( -21.05000000000000071, -12.41227409414968541, -30.59999999999999432 ) ) ;
#136105=LINE ( 'NONE', #76153, #240552 ) ;
#136138=EDGE_LOOP ( 'NONE', ( #96030, #121690, #124625, #241708 ) ) ;
#136178=FACE_OUTER_BOUND ( 'NONE', #80803, .T. ) ;
#136180=CARTESIAN_POINT ( 'NONE',  ( 20.99142135623731065, 11.60000000000000497, -26.57179676972450011 ) ) ;
#136195=DIRECTION ( 'NONE',  ( 0.000000000000000000, 0.000000000000000000, -1.000000000000000000 ) ) ;
#136210=( BOUNDED_SURFACE ( )  B_SPLINE_SURFACE ( 3, 2, ( 
 ( #50313, #54176, #172900 ),
 ( #33380, #189848, #171603 ),
 ( #231553, #29523, #251086 ),
 ( #211994, #213249, #193708 ),
 ( #112880, #209404, #192420 ),
 ( #174184, #72485, #111598 ) ),
 .UNSPECIFIED., .F., .F., .F. ) 
 B_SPLINE_SURFACE_WITH_KNOTS ( ( 4, 2, 4 ),
 ( 3, 3 ),
 ( 6.719893378900589293E-05, 0.0002757154632485561046, 0.0004842319927081063704 ),
 ( 0.000000000000000000, 1.000000000000000000 ),
 .UNSPECIFIED. ) 
 GEOMETRIC_REPRESENTATION_ITEM ( )  RATIONAL_B_SPLINE_SURFACE ( (
 ( 1.000000000000000000, 0.7250110520819700310, 1.000000000000000000),
 ( 1.000000000000000000, 0.7277932058357532430, 1.000000000000000000),
 ( 1.000000000000000000, 0.7278452872619737279, 1.000000000000000000),
 ( 1.000000000000000000, 0.7221445671547080947, 1.000000000000000000),
 ( 1.000000000000000000, 0.7163662143781105440, 1.000000000000000000),
 ( 1.000000000000000000, 0.7071067811865475727, 1.000000000000000000) ) ) 
 REPRESENTATION_ITEM ( '' )  SURFACE ( )  );
#136239=EDGE_LOOP ( 'NONE', ( #61664, #177521, #226152, #225973 ) ) ;
#136269=DIRECTION ( 'NONE',  ( -1.000000000000000000, 0.000000000000000000, 0.000000000000000000 ) ) ;
#136288=EDGE_LOOP ( 'NONE', ( #103676, #135150, #118824, #132261 ) ) ;
#136294=AXIS2_PLACEMENT_3D ( 'NONE', #164047, #165327, #184879 ) ;
#136322=LINE ( 'NONE', #154668, #169625 ) ;
#136339=ORIENTED_EDGE ( 'NONE', *, *, #220877, .F. ) ;
#136354=CARTESIAN_POINT ( 'NONE',  ( 21.46681500597573944, -5.827586677109586333E-16, 6.857511159430853986 ) ) ;
#136379=AXIS2_PLACEMENT_3D ( 'NONE', #222187, #237923, #217056 ) ;
#136384=CIRCLE ( 'NONE', #24017, 0.1000000000000028644 ) ;
#136397=DIRECTION ( 'NONE',  ( 0.000000000000000000, 0.000000000000000000, -1.000000000000000000 ) ) ;
#136398=AXIS2_PLACEMENT_3D ( 'NONE', #208075, #125933, #29458 ) ;
#136411=CARTESIAN_POINT ( 'NONE',  ( -20.85000000000000142, -11.75000000000000000, -30.59999999999999432 ) ) ;
#136424=EDGE_CURVE ( 'NONE', #251180, #29639, #234439, .T. ) ;
#136462=DIRECTION ( 'NONE',  ( -0.000000000000000000, -0.000000000000000000, 1.000000000000000000 ) ) ;
#136466=DIRECTION ( 'NONE',  ( 0.000000000000000000, 0.000000000000000000, 1.000000000000000000 ) ) ;
#136522=LINE ( 'NONE', #210953, #240272 ) ;
#136537=ORIENTED_EDGE ( 'NONE', *, *, #15510, .T. ) ;
#136545=CARTESIAN_POINT ( 'NONE',  ( -18.59999999999999787, -1.851028230140860487, -11.65391326942249250 ) ) ;
#136550=CARTESIAN_POINT ( 'NONE',  ( -20.64999999999999858, 7.249999999999999112, -12.25000000000000000 ) ) ;
#136586=CARTESIAN_POINT ( 'NONE',  ( 20.94999999999999929, 6.649999999999999467, -10.01702717044001822 ) ) ;
#136598=DIRECTION ( 'NONE',  ( 1.000000000000000000, 0.000000000000000000, 0.000000000000000000 ) ) ;
#136600=AXIS2_PLACEMENT_3D ( 'NONE', #214200, #35585, #254570 ) ;
#136601=VERTEX_POINT ( 'NONE', #144303 ) ;
#136602=CARTESIAN_POINT ( 'NONE',  ( 21.05000000000000071, 6.441084688471240050, -0.01771943330862802563 ) ) ;
#136610=ORIENTED_EDGE ( 'NONE', *, *, #184979, .T. ) ;
#136618=AXIS2_PLACEMENT_3D ( 'NONE', #2687, #82202, #181366 ) ;
#136624=FACE_OUTER_BOUND ( 'NONE', #231535, .T. ) ;
#136635=EDGE_LOOP ( 'NONE', ( #34546, #224366, #155096, #63331 ) ) ;
#136638=FACE_OUTER_BOUND ( 'NONE', #145732, .T. ) ;
#136651=AXIS2_PLACEMENT_3D ( 'NONE', #171834, #253885, #135213 ) ;
#136666=CARTESIAN_POINT ( 'NONE',  ( -23.25000000000000000, -9.000000000000001776, -24.20603087734755832 ) ) ;
#136667=ORIENTED_EDGE ( 'NONE', *, *, #52388, .T. ) ;
#136736=CIRCLE ( 'NONE', #157643, 0.4000000000000010214 ) ;
#136748=DIRECTION ( 'NONE',  ( 0.000000000000000000, 1.000000000000000000, -6.308085367188393199E-16 ) ) ;
#136811=LINE ( 'NONE', #80673, #235766 ) ;
#136817=AXIS2_PLACEMENT_3D ( 'NONE', #23635, #198380, #161853 ) ;
#136819=DIRECTION ( 'NONE',  ( -7.304098846218134667E-16, -1.000000000000000000, 0.000000000000000000 ) ) ;
#136820=CARTESIAN_POINT ( 'NONE',  ( 22.39999999999999503, 0.000000000000000000, 11.64957080754479968 ) ) ;
#136824=CARTESIAN_POINT ( 'NONE',  ( 20.22483756094572271, 9.501904678871314402, -8.139539128714682548 ) ) ;
#136832=CARTESIAN_POINT ( 'NONE',  ( -21.44999999999999929, 7.150000000000000355, -12.25000000000000000 ) ) ;
#136833=DIRECTION ( 'NONE',  ( 1.000000000000000000, -0.000000000000000000, -0.000000000000000000 ) ) ;
#136858=DIRECTION ( 'NONE',  ( 1.000000000000000000, 0.000000000000000000, 0.000000000000000000 ) ) ;
#136883=DIRECTION ( 'NONE',  ( 1.000000000000000000, 0.000000000000000000, 0.000000000000000000 ) ) ;
#136905=ORIENTED_EDGE ( 'NONE', *, *, #227902, .T. ) ;
#136985=VERTEX_POINT ( 'NONE', #179037 ) ;
#137001=ORIENTED_EDGE ( 'NONE', *, *, #49642, .F. ) ;
#137003=DIRECTION ( 'NONE',  ( 1.000000000000000000, 0.000000000000000000, 0.000000000000000000 ) ) ;
#137009=VECTOR ( 'NONE', #230808, 1000.000000000000000 ) ;
#137013=EDGE_CURVE ( 'NONE', #169470, #213112, #189547, .T. ) ;
#137030=FACE_OUTER_BOUND ( 'NONE', #138168, .T. ) ;
#137056=FACE_OUTER_BOUND ( 'NONE', #130557, .T. ) ;
#137065=ADVANCED_FACE ( 'NONE', ( #164580 ), #224533, .F. ) ;
#137069=CARTESIAN_POINT ( 'NONE',  ( 20.94999999999999574, 6.350000000000004974, -9.843822089683131438 ) ) ;
#137081=ORIENTED_EDGE ( 'NONE', *, *, #73671, .T. ) ;
#137088=VERTEX_POINT ( 'NONE', #26348 ) ;
#137119=ORIENTED_EDGE ( 'NONE', *, *, #136424, .T. ) ;
#137150=DIRECTION ( 'NONE',  ( -3.440080580676165868E-14, -0.1298341882520124002, -0.9915357197604841577 ) ) ;
#137172=CARTESIAN_POINT ( 'NONE',  ( 23.14999999999998437, 0.000000000000000000, 0.000000000000000000 ) ) ;
#137177=TOROIDAL_SURFACE ( 'NONE', #158081, 7.800000000000000711, 0.1000000000000000056 ) ;
#137274=ORIENTED_EDGE ( 'NONE', *, *, #17648, .T. ) ;
#137296=CIRCLE ( 'NONE', #158203, 0.1999999999999987899 ) ;
#137299=ORIENTED_EDGE ( 'NONE', *, *, #54991, .F. ) ;
#137323=EDGE_CURVE ( 'NONE', #41537, #255042, #39, .T. ) ;
#137328=CARTESIAN_POINT ( 'NONE',  ( -22.39999999999999858, 7.790779598373403836, 0.000000000000000000 ) ) ;
#137332=LINE ( 'NONE', #237737, #38069 ) ;
#137334=ORIENTED_EDGE ( 'NONE', *, *, #79324, .F. ) ;
#137368=CARTESIAN_POINT ( 'NONE',  ( 20.94999999999999929, -1.349153571976048571, -41.28749733558988311 ) ) ;
#137377=ADVANCED_FACE ( 'NONE', ( #117436 ), #134318, .T. ) ;
#137378=DIRECTION ( 'NONE',  ( -1.000000000000000000, -0.000000000000000000, -0.000000000000000000 ) ) ;
#137394=ADVANCED_FACE ( 'NONE', ( #247644 ), #142692, .F. ) ;
#137412=ADVANCED_FACE ( 'NONE', ( #49448 ), #252721, .T. ) ;
#137417=VERTEX_POINT ( 'NONE', #203392 ) ;
#137422=( NAMED_UNIT ( * ) SI_UNIT ( $, .STERADIAN. ) SOLID_ANGLE_UNIT ( ) );
#137437=CARTESIAN_POINT ( 'NONE',  ( 21.05933563467872460, 10.72452471208132074, -12.19364774895595538 ) ) ;
#137439=CARTESIAN_POINT ( 'NONE',  ( 18.49999999999999289, 6.450000000000001066, 11.75000000000000000 ) ) ;
#137483=CARTESIAN_POINT ( 'NONE',  ( -18.50000000000000000, 9.350000000000001421, -12.34999999999999964 ) ) ;
#137495=CARTESIAN_POINT ( 'NONE',  ( 23.25000000000000000, -8.596261682242985813, -24.04987248284971812 ) ) ;
#137511=DIRECTION ( 'NONE',  ( 0.000000000000000000, 0.000000000000000000, -1.000000000000000000 ) ) ;
#137515=CARTESIAN_POINT ( 'NONE',  ( -23.25000000000000000, 11.75000000000000000, -33.50000000000000000 ) ) ;
#137516=CARTESIAN_POINT ( 'NONE',  ( -21.05000000000000071, 0.000000000000000000, -29.40000000000000213 ) ) ;
#137530=DIRECTION ( 'NONE',  ( -0.000000000000000000, -0.000000000000000000, -1.000000000000000000 ) ) ;
#137563=CARTESIAN_POINT ( 'NONE',  ( -18.59999999999999787, 9.350000000000001421, -12.34999999999999964 ) ) ;
#137569=CIRCLE ( 'NONE', #37659, 0.1000000000000000472 ) ;
#137575=ORIENTED_EDGE ( 'NONE', *, *, #244142, .F. ) ;
#137579=DIRECTION ( 'NONE',  ( -0.000000000000000000, 0.000000000000000000, 1.000000000000000000 ) ) ;
#137631=CARTESIAN_POINT ( 'NONE',  ( 18.49999999999999289, 10.20857864376269575, -24.65000000000000213 ) ) ;
#137673=CARTESIAN_POINT ( 'NONE',  ( 18.49999999999999289, 6.450000000000001066, -10.01702717044001822 ) ) ;
#137686=CIRCLE ( 'NONE', #46120, 0.5000000000000013323 ) ;
#137697=VERTEX_POINT ( 'NONE', #237066 ) ;
#137721=DIRECTION ( 'NONE',  ( 0.000000000000000000, 0.000000000000000000, -1.000000000000000000 ) ) ;
#137765=ORIENTED_EDGE ( 'NONE', *, *, #90525, .T. ) ;
#137774=AXIS2_PLACEMENT_3D ( 'NONE', #192666, #14031, #115689 ) ;
#137833=AXIS2_PLACEMENT_3D ( 'NONE', #48067, #88451, #229287 ) ;
#137858=CIRCLE ( 'NONE', #29774, 0.09999999999999939493 ) ;
#137881=CARTESIAN_POINT ( 'NONE',  ( 21.11833042828132889, 6.445644693855303586, 0.007100509059361484118 ) ) ;
#137884=CIRCLE ( 'NONE', #17130, 0.5000000000000004441 ) ;
#137925=DIRECTION ( 'NONE',  ( 0.000000000000000000, 0.000000000000000000, 1.000000000000000000 ) ) ;
#137927=CARTESIAN_POINT ( 'NONE',  ( 18.47073956224755165, -9.471729412471800558, -7.108685752817913261 ) ) ;
#137930=EDGE_CURVE ( 'NONE', #219323, #13885, #201152, .T. ) ;
#137957=ORIENTED_EDGE ( 'NONE', *, *, #125577, .T. ) ;
#137965=LINE ( 'NONE', #77997, #251931 ) ;
#137968=CARTESIAN_POINT ( 'NONE',  ( 20.85000000000000142, -0.3238857010703366512, -33.45758958931398297 ) ) ;
#138008=CARTESIAN_POINT ( 'NONE',  ( -21.13498764882296044, 0.001656394731329963003, 6.495618143473942396 ) ) ;
#138010=ORIENTED_EDGE ( 'NONE', *, *, #234578, .T. ) ;
#138023=EDGE_CURVE ( 'NONE', #178493, #143742, #63787, .T. ) ;
#138026=ORIENTED_EDGE ( 'NONE', *, *, #143512, .T. ) ;
#138031=VERTEX_POINT ( 'NONE', #137631 ) ;
#138039=CARTESIAN_POINT ( 'NONE',  ( 21.97500000000000497, 9.749999999999998224, -21.15000000000000213 ) ) ;
#138044=DIRECTION ( 'NONE',  ( 1.000000000000000000, 0.000000000000000000, 0.000000000000000000 ) ) ;
#138049=DIRECTION ( 'NONE',  ( 0.000000000000000000, 0.9915357197604860451, -0.1298341882519964408 ) ) ;
#138060=LINE ( 'NONE', #224960, #237215 ) ;
#138063=TOROIDAL_SURFACE ( 'NONE', #25656, 0.2000000000000000111, 0.1000000000000000056 ) ;
#138106=DIRECTION ( 'NONE',  ( 0.000000000000000000, -0.9654727137038715545, 0.2605042016806676242 ) ) ;
#138147=CARTESIAN_POINT ( 'NONE',  ( -21.05000000000000071, -1.360870587192041681, -8.072997927090961312 ) ) ;
#138168=EDGE_LOOP ( 'NONE', ( #87027, #142599, #253376, #1923 ) ) ;
#138194=EDGE_CURVE ( 'NONE', #169542, #66484, #68065, .T. ) ;
#138210=PLANE ( 'NONE',  #144887 ) ;
#138218=CIRCLE ( 'NONE', #55377, 0.1000000000000000056 ) ;
#138224=FACE_OUTER_BOUND ( 'NONE', #46829, .T. ) ;
#138243=AXIS2_PLACEMENT_3D ( 'NONE', #19282, #77955, #179656 ) ;
#138292=ADVANCED_FACE ( 'NONE', ( #31858 ), #91804, .F. ) ;
#138304=ADVANCED_FACE ( 'NONE', ( #74843 ), #228762, .T. ) ;
#138311=EDGE_LOOP ( 'NONE', ( #63694, #72050, #2200, #162776 ) ) ;
#138317=CARTESIAN_POINT ( 'NONE',  ( -21.05000000000000071, -1.162701749938009677, -8.099999999999999645 ) ) ;
#138361=CARTESIAN_POINT ( 'NONE',  ( 20.94999999999999574, -11.48912529307605901, -3.100000000000000533 ) ) ;
#138366=VERTEX_POINT ( 'NONE', #137328 ) ;
#138468=DIRECTION ( 'NONE',  ( 0.000000000000000000, 0.000000000000000000, -1.000000000000000000 ) ) ;
#138473=CARTESIAN_POINT ( 'NONE',  ( 21.05000000000000071, -11.74999999999999112, -30.59999999999999432 ) ) ;
#138482=LINE ( 'NONE', #197195, #185633 ) ;
#138502=VERTEX_POINT ( 'NONE', #23849 ) ;
#138575=AXIS2_PLACEMENT_3D ( 'NONE', #19329, #238365, #55855 ) ;
#138607=CARTESIAN_POINT ( 'NONE',  ( 20.94999999999999929, -11.48912529307605546, -30.59999999999999432 ) ) ;
#138618=CIRCLE ( 'NONE', #163602, 0.5999999999999998668 ) ;
#138639=ORIENTED_EDGE ( 'NONE', *, *, #88445, .F. ) ;
#138685=DIRECTION ( 'NONE',  ( -1.000000000000000000, 0.000000000000000000, 0.000000000000000000 ) ) ;
#138729=CARTESIAN_POINT ( 'NONE',  ( -21.05000000000000071, -11.29603075033528015, -30.45210084033612929 ) ) ;
#138767=LINE ( 'NONE', #162251, #207511 ) ;
#138792=AXIS2_PLACEMENT_3D ( 'NONE', #163970, #239656, #6152 ) ;
#138834=EDGE_CURVE ( 'NONE', #112086, #126038, #243200, .T. ) ;
#138881=CIRCLE ( 'NONE', #26515, 12.87500000000000000 ) ;
#138899=VERTEX_POINT ( 'NONE', #243519 ) ;
#138909=VECTOR ( 'NONE', #16715, 1000.000000000000227 ) ;
#138911=VERTEX_POINT ( 'NONE', #208263 ) ;
#138921=CARTESIAN_POINT ( 'NONE',  ( -23.15000000000000213, 0.000000000000000000, -33.50000000000000000 ) ) ;
#138940=CARTESIAN_POINT ( 'NONE',  ( 23.14999999999999503, 11.75000000000000711, 11.75000000000000000 ) ) ;
#138959=ORIENTED_EDGE ( 'NONE', *, *, #140332, .F. ) ;
#138987=CARTESIAN_POINT ( 'NONE',  ( -22.59999999999999787, 0.000000000000000000, 0.000000000000000000 ) ) ;
#138991=ORIENTED_EDGE ( 'NONE', *, *, #222843, .F. ) ;
#139038=AXIS2_PLACEMENT_3D ( 'NONE', #123536, #25716, #124825 ) ;
#139074=EDGE_CURVE ( 'NONE', #6293, #137417, #231680, .T. ) ;
#139076=CARTESIAN_POINT ( 'NONE',  ( -21.05000000000000071, -11.39257802170567224, -3.073949579831933843 ) ) ;
#139136=DIRECTION ( 'NONE',  ( 0.000000000000000000, -0.9908441862701600211, -0.1350103645451876666 ) ) ;
#139156=CARTESIAN_POINT ( 'NONE',  ( 21.13422380239043363, 6.493326514805634275, -9.351243737687475743E-16 ) ) ;
#139222=DIRECTION ( 'NONE',  ( 0.000000000000000000, 0.000000000000000000, -1.000000000000000000 ) ) ;
#139228=CIRCLE ( 'NONE', #89180, 0.5000000000000004441 ) ;
#139231=ORIENTED_EDGE ( 'NONE', *, *, #96091, .F. ) ;
#139238=CIRCLE ( 'NONE', #168540, 7.900000000000000355 ) ;
#139254=CYLINDRICAL_SURFACE ( 'NONE', #36927, 0.09999999999999892308 ) ;
#139322=EDGE_LOOP ( 'NONE', ( #61497, #253391, #18141, #97844 ) ) ;
#139342=TOROIDAL_SURFACE ( 'NONE', #10210, 0.2000000000000000111, 0.1000000000000000056 ) ;
#139353=CARTESIAN_POINT ( 'NONE',  ( 21.87500000000000355, 9.749999999999998224, -21.25000000000000000 ) ) ;
#139376=CARTESIAN_POINT ( 'NONE',  ( 20.72390388899083646, 10.58996311842368243, -7.511348295744856074 ) ) ;
#139403=CARTESIAN_POINT ( 'NONE',  ( -21.05000000000000071, 0.03363273533364569134, 6.258817194681472351 ) ) ;
#139408=CYLINDRICAL_SURFACE ( 'NONE', #33119, 0.09999999999999939493 ) ;
#139430=CARTESIAN_POINT ( 'NONE',  ( 20.99999999999997868, 0.000000000000000000, 0.000000000000000000 ) ) ;
#139433=ORIENTED_EDGE ( 'NONE', *, *, #57389, .F. ) ;
#139453=CIRCLE ( 'NONE', #26486, 2.100000000000002309 ) ;
#139456=EDGE_CURVE ( 'NONE', #103887, #117101, #143028, .T. ) ;
#139459=ORIENTED_EDGE ( 'NONE', *, *, #25811, .T. ) ;
#139469=DIRECTION ( 'NONE',  ( 0.000000000000000000, -0.8660254037844247188, 0.5000000000000245359 ) ) ;
#139497=DIRECTION ( 'NONE',  ( 0.000000000000000000, 0.9908441862701596881, -0.1350103645451904977 ) ) ;
#139501=EDGE_LOOP ( 'NONE', ( #99322, #250029, #254268 ) ) ;
#139544=FACE_OUTER_BOUND ( 'NONE', #234571, .T. ) ;
#139567=DIRECTION ( 'NONE',  ( 0.000000000000000000, 0.000000000000000000, -1.000000000000000000 ) ) ;
#139575=DIRECTION ( 'NONE',  ( 1.000000000000000000, 0.000000000000000000, 0.000000000000000000 ) ) ;
#139592=EDGE_LOOP ( 'NONE', ( #166168, #241629, #60495, #14859 ) ) ;
#139596=ORIENTED_EDGE ( 'NONE', *, *, #225858, .F. ) ;
#139601=ADVANCED_FACE ( 'NONE', ( #198647 ), #168051, .T. ) ;
#139610=ORIENTED_EDGE ( 'NONE', *, *, #5136, .F. ) ;
#139637=VECTOR ( 'NONE', #162362, 999.9999999999998863 ) ;
#139658=ADVANCED_FACE ( 'NONE', ( #180381 ), #255999, .T. ) ;
#139673=ORIENTED_EDGE ( 'NONE', *, *, #95501, .T. ) ;
#139699=EDGE_LOOP ( 'NONE', ( #246754, #59114, #1576, #223283, #60090, #177480, #200193, #180109, #189570, #207620, #35087, #60724 ) ) ;
#139700=FACE_OUTER_BOUND ( 'NONE', #103217, .T. ) ;
#139737=DIRECTION ( 'NONE',  ( -1.000000000000000000, -3.265361837132813093E-16, 0.000000000000000000 ) ) ;
#139741=CARTESIAN_POINT ( 'NONE',  ( -20.64999999999999858, -9.500000000000001776, -23.60603087734756045 ) ) ;
#139751=ORIENTED_EDGE ( 'NONE', *, *, #216786, .F. ) ;
#139762=FACE_OUTER_BOUND ( 'NONE', #144407, .T. ) ;
#139796=VERTEX_POINT ( 'NONE', #75706 ) ;
#139811=EDGE_CURVE ( 'NONE', #114284, #19733, #36604, .T. ) ;
#139840=CARTESIAN_POINT ( 'NONE',  ( -18.59999999999999787, 7.021664781900089913, -37.33356540189728889 ) ) ;
#139841=ORIENTED_EDGE ( 'NONE', *, *, #206628, .T. ) ;
#139842=CARTESIAN_POINT ( 'NONE',  ( -20.92356734117541706, 10.31973158070286622, -39.05053347133544150 ) ) ;
#139862=ORIENTED_EDGE ( 'NONE', *, *, #51529, .T. ) ;
#139879=VERTEX_POINT ( 'NONE', #201129 ) ;
#139905=DIRECTION ( 'NONE',  ( 0.000000000000000000, 0.000000000000000000, -1.000000000000000000 ) ) ;
#139915=ADVANCED_FACE ( 'NONE', ( #5469 ), #85004, .F. ) ;
#139928=CARTESIAN_POINT ( 'NONE',  ( 20.94999999999999574, 10.47338541491290442, -7.578654464248542943 ) ) ;
#139940=ORIENTED_EDGE ( 'NONE', *, *, #124426, .T. ) ;
#140018=VERTEX_POINT ( 'NONE', #112318 ) ;
#140057=ORIENTED_EDGE ( 'NONE', *, *, #1416, .T. ) ;
#140101=EDGE_CURVE ( 'NONE', #197300, #49158, #172521, .T. ) ;
#140106=LINE ( 'NONE', #21485, #224706 ) ;
#140109=ORIENTED_EDGE ( 'NONE', *, *, #243323, .F. ) ;
#140135=VERTEX_POINT ( 'NONE', #116171 ) ;
#140182=CARTESIAN_POINT ( 'NONE',  ( 23.25000000000000000, -11.64999999999999147, 11.75000000000000000 ) ) ;
#140266=DIRECTION ( 'NONE',  ( 0.000000000000000000, 0.6728971962616783209, 0.7397360091702797069 ) ) ;
#140273=CARTESIAN_POINT ( 'NONE',  ( 18.59999999999999076, -1.835859311443637010, -45.10443916879852821 ) ) ;
#140304=CARTESIAN_POINT ( 'NONE',  ( -21.44999999999999929, 7.150000000000000355, -12.34999999999999964 ) ) ;
#140332=EDGE_CURVE ( 'NONE', #249634, #58239, #46868, .T. ) ;
#140338=CIRCLE ( 'NONE', #56441, 0.1999999999999987899 ) ;
#140348=ORIENTED_EDGE ( 'NONE', *, *, #204096, .F. ) ;
#140372=ORIENTED_EDGE ( 'NONE', *, *, #170397, .F. ) ;
#140388=AXIS2_PLACEMENT_3D ( 'NONE', #120465, #23928, #86405 ) ;
#140403=CARTESIAN_POINT ( 'NONE',  ( -18.50000000000000000, -1.866714910057309273, -11.75267524628200633 ) ) ;
#140429=CARTESIAN_POINT ( 'NONE',  ( -18.39999999999999858, -9.519327731092436906, -6.972976376559334888 ) ) ;
#140451=AXIS2_PLACEMENT_3D ( 'NONE', #191420, #170595, #94842 ) ;
#140457=CARTESIAN_POINT ( 'NONE',  ( 21.14999999999999858, 6.540656951701244282, -9.351243737687475743E-16 ) ) ;
#140484=ORIENTED_EDGE ( 'NONE', *, *, #10190, .T. ) ;
#140486=CARTESIAN_POINT ( 'NONE',  ( 22.40000000000020819, -0.1008583690996671112, 11.74956712348970100 ) ) ;
#140490=CIRCLE ( 'NONE', #165467, 4.049999999999998934 ) ;
#140499=CARTESIAN_POINT ( 'NONE',  ( -21.14999999999999858, 11.65000000000000036, -0.1000000000000028644 ) ) ;
#140508=ORIENTED_EDGE ( 'NONE', *, *, #145840, .F. ) ;
#140535=CIRCLE ( 'NONE', #98818, 0.1000000000000001860 ) ;
#140551=FACE_OUTER_BOUND ( 'NONE', #46793, .T. ) ;
#140558=DIRECTION ( 'NONE',  ( -0.000000000000000000, 1.000000000000000000, -0.000000000000000000 ) ) ;
#140575=CARTESIAN_POINT ( 'NONE',  ( -23.15000000000000213, -11.65000000000000036, -30.50000000000000000 ) ) ;
#140582=CARTESIAN_POINT ( 'NONE',  ( 18.59999999999999076, 6.550000000000000711, -21.15000000000000213 ) ) ;
#140603=EDGE_CURVE ( 'NONE', #253474, #256624, #207919, .T. ) ;
#140652=ORIENTED_EDGE ( 'NONE', *, *, #12566, .F. ) ;
#140711=CIRCLE ( 'NONE', #178146, 0.4000000000000010214 ) ;
#140714=CIRCLE ( 'NONE', #115770, 0.09999999999999939493 ) ;
#140727=LINE ( 'NONE', #102862, #27204 ) ;
#140754=EDGE_CURVE ( 'NONE', #183242, #28201, #97598, .T. ) ;
#140760=EDGE_LOOP ( 'NONE', ( #176576, #49855, #188903, #59968, #91731 ) ) ;
#140808=CARTESIAN_POINT ( 'NONE',  ( 18.59999999999999432, 1.162701749938009677, -8.000000000000000000 ) ) ;
#140810=CARTESIAN_POINT ( 'NONE',  ( -23.25000000000000000, -1.249999999999999334, -41.30048075441507649 ) ) ;
#140873=CARTESIAN_POINT ( 'NONE',  ( -23.25000000000000000, 0.000000000000000000, 0.000000000000000000 ) ) ;
#140903=AXIS2_PLACEMENT_3D ( 'NONE', #49914, #167327, #111183 ) ;
#140927=AXIS2_PLACEMENT_3D ( 'NONE', #73549, #110069, #249598 ) ;
#140958=VERTEX_POINT ( 'NONE', #185464 ) ;
#140997=AXIS2_PLACEMENT_3D ( 'NONE', #167588, #123308, #185837 ) ;
#140998=ORIENTED_EDGE ( 'NONE', *, *, #38261, .T. ) ;
#141020=SPHERICAL_SURFACE ( 'NONE', #87221, 0.1000000000000000056 ) ;
#141051=FACE_OUTER_BOUND ( 'NONE', #240638, .T. ) ;
#141073=ORIENTED_EDGE ( 'NONE', *, *, #185465, .F. ) ;
#141084=AXIS2_PLACEMENT_3D ( 'NONE', #7282, #177307, #166402 ) ;
#141087=LINE ( 'NONE', #182792, #180626 ) ;
#141113=EDGE_CURVE ( 'NONE', #15934, #56184, #151497, .T. ) ;
#141117=TOROIDAL_SURFACE ( 'NONE', #236963, 0.2000000000000000111, 0.1000000000000000056 ) ;
#141127=CARTESIAN_POINT ( 'NONE',  ( -21.14999999999999858, 0.000000000000000000, 11.64957080754479968 ) ) ;
#141135=VERTEX_POINT ( 'NONE', #88908 ) ;
#141151=CARTESIAN_POINT ( 'NONE',  ( -20.91682497891422798, 10.32263460346243633, -39.06059579686719019 ) ) ;
#141162=DIRECTION ( 'NONE',  ( 1.000000000000000000, 2.952720810173289112E-16, -0.000000000000000000 ) ) ;
#141166=CIRCLE ( 'NONE', #78604, 11.70000000000000639 ) ;
#141191=PLANE ( 'NONE',  #224091 ) ;
#141215=ORIENTED_EDGE ( 'NONE', *, *, #60837, .T. ) ;
#141291=ADVANCED_FACE ( 'NONE', ( #15844 ), #114759, .T. ) ;
#141330=CARTESIAN_POINT ( 'NONE',  ( -20.99749315643149217, 11.74999999999999645, -26.48519423124078642 ) ) ;
#141347=DIRECTION ( 'NONE',  ( 1.000000000000000000, 0.000000000000000000, 0.000000000000000000 ) ) ;
#141408=ORIENTED_EDGE ( 'NONE', *, *, #150159, .F. ) ;
#141418=VERTEX_POINT ( 'NONE', #66497 ) ;
#141432=EDGE_CURVE ( 'NONE', #176380, #120793, #202154, .T. ) ;
#141467=LINE ( 'NONE', #24118, #15744 ) ;
#141481=CARTESIAN_POINT ( 'NONE',  ( -20.54999999999999716, 2.388061258337340615E-16, -31.59999999999999787 ) ) ;
#141494=DIRECTION ( 'NONE',  ( 0.000000000000000000, 1.000000000000000000, 0.000000000000000000 ) ) ;
#141502=EDGE_CURVE ( 'NONE', #180993, #147671, #31582, .T. ) ;
#141538=DIRECTION ( 'NONE',  ( 0.000000000000000000, 0.000000000000000000, -1.000000000000000000 ) ) ;
#141572=AXIS2_PLACEMENT_3D ( 'NONE', #82750, #103612, #5799 ) ;
#141594=VERTEX_POINT ( 'NONE', #156332 ) ;
#141596=CARTESIAN_POINT ( 'NONE',  ( -20.64999999999999858, 7.150000000000000355, -21.15000000000000213 ) ) ;
#141605=VERTEX_POINT ( 'NONE', #237122 ) ;
#141613=DIRECTION ( 'NONE',  ( 0.000000000000000000, 1.000000000000000000, -3.469446951953635015E-14 ) ) ;
#141677=EDGE_CURVE ( 'NONE', #92976, #13199, #198316, .T. ) ;
#141688=CARTESIAN_POINT ( 'NONE',  ( -18.50000000000000000, -1.687074390091559906, 12.81457296654165212 ) ) ;
#141793=AXIS2_PLACEMENT_3D ( 'NONE', #38816, #15412, #115776 ) ;
#141796=AXIS2_PLACEMENT_3D ( 'NONE', #95910, #114205, #93350 ) ;
#141828=DIRECTION ( 'NONE',  ( 0.000000000000000000, 0.9915357197604882655, -0.1298341882519793711 ) ) ;
#141852=ADVANCED_FACE ( 'NONE', ( #66181 ), #14993, .F. ) ;
#141866=ORIENTED_EDGE ( 'NONE', *, *, #17181, .F. ) ;
#141874=DIRECTION ( 'NONE',  ( 0.000000000000000000, 0.000000000000000000, -1.000000000000000000 ) ) ;
#141896=EDGE_CURVE ( 'NONE', #141135, #192810, #248669, .T. ) ;
#141898=AXIS2_PLACEMENT_3D ( 'NONE', #188984, #231978, #168180 ) ;
#141932=LINE ( 'NONE', #238471, #184228 ) ;
#141967=AXIS2_PLACEMENT_3D ( 'NONE', #149418, #50275, #129821 ) ;
#141982=DIRECTION ( 'NONE',  ( 0.000000000000000000, 0.000000000000000000, 1.000000000000000000 ) ) ;
#141998=CIRCLE ( 'NONE', #125263, 0.1000000000000002554 ) ;
#142000=DIRECTION ( 'NONE',  ( -1.000000000000000000, -0.000000000000000000, -0.000000000000000000 ) ) ;
#142033=ADVANCED_FACE ( 'NONE', ( #247371 ), #227813, .T. ) ;
#142047=DIRECTION ( 'NONE',  ( 1.713247197920696616E-14, 0.9876197685951252359, -0.1568667991644863424 ) ) ;
#142055=CARTESIAN_POINT ( 'NONE',  ( -21.70464131381649509, 7.095358018967854896, 0.000000000000000000 ) ) ;
#142089=DIRECTION ( 'NONE',  ( -0.000000000000000000, 0.6132151058540549204, -0.7899159663865520375 ) ) ;
#142101=DIRECTION ( 'NONE',  ( -0.8660254037844500319, 0.000000000000000000, 0.4999999999999800715 ) ) ;
#142103=CARTESIAN_POINT ( 'NONE',  ( -18.59999999999999787, 1.736257131597397585, -11.56865232901749962 ) ) ;
#142124=DIRECTION ( 'NONE',  ( 1.000000000000000000, 0.000000000000000000, 0.000000000000000000 ) ) ;
#142139=ORIENTED_EDGE ( 'NONE', *, *, #79730, .T. ) ;
#142143=CYLINDRICAL_SURFACE ( 'NONE', #195916, 4.049999999999998934 ) ;
#142144=VERTEX_POINT ( 'NONE', #24200 ) ;
#142174=EDGE_CURVE ( 'NONE', #112086, #56194, #240659, .T. ) ;
#142196=AXIS2_PLACEMENT_3D ( 'NONE', #2507, #22106, #44231 ) ;
#142225=CARTESIAN_POINT ( 'NONE',  ( 20.85000000000000142, -11.74999999999999112, -30.50000000000000000 ) ) ;
#142230=ORIENTED_EDGE ( 'NONE', *, *, #191196, .T. ) ;
#142254=CARTESIAN_POINT ( 'NONE',  ( -20.15000000000000568, 9.291421356237307805, -12.34999999999999964 ) ) ;
#142277=B_SPLINE_CURVE_WITH_KNOTS ( 'NONE', 3,
 ( #90721, #170323, #145563, #209394, #28228, #7345, #249815, #50304, #166458, #150712 ),
 .UNSPECIFIED., .F., .F.,
 ( 4, 3, 3, 4 ),
 ( 0.000000000000000000, 0.0002000000000002884074, 0.001000000000045112589, 0.001967863649472103085 ),
 .UNSPECIFIED. ) ;
#142284=FACE_OUTER_BOUND ( 'NONE', #250394, .T. ) ;
#142315=CARTESIAN_POINT ( 'NONE',  ( -18.59999999999999787, 9.250000000000001776, -21.15000000000000213 ) ) ;
#142378=VECTOR ( 'NONE', #220975, 999.9999999999998863 ) ;
#142392=DIRECTION ( 'NONE',  ( 1.000000000000000000, -0.000000000000000000, -0.000000000000000000 ) ) ;
#142443=EDGE_LOOP ( 'NONE', ( #176968, #90509, #40588, #168954 ) ) ;
#142475=ORIENTED_EDGE ( 'NONE', *, *, #81431, .F. ) ;
#142524=ADVANCED_FACE ( 'NONE', ( #83492 ), #88635, .T. ) ;
#142530=AXIS2_PLACEMENT_3D ( 'NONE', #77538, #18871, #78828 ) ;
#142567=CARTESIAN_POINT ( 'NONE',  ( -23.15000000000000213, -9.600000000000001421, 11.74999999999999645 ) ) ;
#142582=CARTESIAN_POINT ( 'NONE',  ( -18.50000324121759121, 10.29307482167955001, -38.95864214669403225 ) ) ;
#142591=CARTESIAN_POINT ( 'NONE',  ( -20.94999999999999929, 11.64999999999999680, -26.71613433702190576 ) ) ;
#142599=ORIENTED_EDGE ( 'NONE', *, *, #98367, .F. ) ;
#142645=CARTESIAN_POINT ( 'NONE',  ( -20.64999999999999858, 0.000000000000000000, -33.50000000000000000 ) ) ;
#142685=CARTESIAN_POINT ( 'NONE',  ( 22.59999999999999787, 0.04781839070480805448, 11.75002241904723022 ) ) ;
#142692=TOROIDAL_SURFACE ( 'NONE', #242661, 0.9750000000000019762, 0.1000000000000000056 ) ;
#142695=DIRECTION ( 'NONE',  ( 0.000000000000000000, -0.8700118002898321601, 0.4930308989875230030 ) ) ;
#142696=EDGE_CURVE ( 'NONE', #31765, #163039, #230759, .T. ) ;
#142700=CARTESIAN_POINT ( 'NONE',  ( -21.05000000000000071, 0.000000000000000000, -33.50000000000000000 ) ) ;
#142702=DIRECTION ( 'NONE',  ( -1.000000000000000000, -2.952720810173289112E-16, 0.000000000000000000 ) ) ;
#142723=DIRECTION ( 'NONE',  ( 1.000000000000000000, 0.000000000000000000, 0.000000000000000000 ) ) ;
#142740=EDGE_CURVE ( 'NONE', #103735, #5222, #254138, .T. ) ;
#142756=ORIENTED_EDGE ( 'NONE', *, *, #206628, .F. ) ;
#142775=DIRECTION ( 'NONE',  ( 0.000000000000000000, -1.000000000000000000, 0.000000000000000000 ) ) ;
#142806=PLANE ( 'NONE',  #250557 ) ;
#142824=EDGE_CURVE ( 'NONE', #162495, #248548, #252658, .T. ) ;
#142834=EDGE_CURVE ( 'NONE', #156131, #192659, #123879, .T. ) ;
#142840=CIRCLE ( 'NONE', #88687, 12.87500000000000000 ) ;
#142845=AXIS2_PLACEMENT_3D ( 'NONE', #37156, #98344, #80068 ) ;
#142885=ORIENTED_EDGE ( 'NONE', *, *, #81664, .F. ) ;
#142886=EDGE_CURVE ( 'NONE', #207337, #211613, #65594, .T. ) ;
#142912=ADVANCED_FACE ( 'NONE', ( #181056 ), #242279, .T. ) ;
#142936=CARTESIAN_POINT ( 'NONE',  ( 21.05000000000000071, -1.849084418627015891, -11.65601052144712391 ) ) ;
#142941=EDGE_CURVE ( 'NONE', #106325, #143460, #62378, .T. ) ;
#142944=DIRECTION ( 'NONE',  ( -1.000000000000000000, -3.265361837132813093E-16, 0.000000000000000000 ) ) ;
#142947=ORIENTED_EDGE ( 'NONE', *, *, #102570, .T. ) ;
#142962=EDGE_CURVE ( 'NONE', #119379, #238460, #123638, .T. ) ;
#142990=CARTESIAN_POINT ( 'NONE',  ( 21.05000000000000071, 0.09779029130879170195, 6.257814610476124528 ) ) ;
#143019=VERTEX_POINT ( 'NONE', #51768 ) ;
#143028=CIRCLE ( 'NONE', #238736, 0.1999999999999996503 ) ;
#143073=FACE_OUTER_BOUND ( 'NONE', #109931, .T. ) ;
#143092=ORIENTED_EDGE ( 'NONE', *, *, #97645, .T. ) ;
#143095=ORIENTED_EDGE ( 'NONE', *, *, #7214, .T. ) ;
#143109=VERTEX_POINT ( 'NONE', #149632 ) ;
#143143=DIRECTION ( 'NONE',  ( 1.000000000000000000, -0.000000000000000000, -0.000000000000000000 ) ) ;
#143162=EDGE_CURVE ( 'NONE', #56398, #192073, #215611, .T. ) ;
#143165=CARTESIAN_POINT ( 'NONE',  ( -22.00411653962169467, 7.253442868370059138, 0.09903810578604851922 ) ) ;
#143183=AXIS2_PLACEMENT_3D ( 'NONE', #104726, #166055, #106024 ) ;
#143224=AXIS2_PLACEMENT_3D ( 'NONE', #11586, #211056, #91102 ) ;
#143243=ORIENTED_EDGE ( 'NONE', *, *, #142824, .T. ) ;
#143252=EDGE_CURVE ( 'NONE', #244818, #140958, #82315, .T. ) ;
#143255=CARTESIAN_POINT ( 'NONE',  ( -20.64999999999999858, -9.000000000000003553, -9.893969122652444881 ) ) ;
#143264=ORIENTED_EDGE ( 'NONE', *, *, #199555, .T. ) ;
#143270=DIRECTION ( 'NONE',  ( 2.940209281316622495E-16, -1.000000000000000000, -1.764125568789973497E-15 ) ) ;
#143281=EDGE_LOOP ( 'NONE', ( #97496, #118209, #191808, #163427 ) ) ;
#143283=CARTESIAN_POINT ( 'NONE',  ( 23.14999999999999858, 6.649999999999999467, -12.35000000000000320 ) ) ;
#143318=VERTEX_POINT ( 'NONE', #80302 ) ;
#143327=CARTESIAN_POINT ( 'NONE',  ( 21.53699400380599371, 6.787711793191639309, -6.911788849595090767E-16 ) ) ;
#143402=ORIENTED_EDGE ( 'NONE', *, *, #251362, .T. ) ;
#143420=FACE_OUTER_BOUND ( 'NONE', #30588, .T. ) ;
#143424=ORIENTED_EDGE ( 'NONE', *, *, #63523, .F. ) ;
#143438=AXIS2_PLACEMENT_3D ( 'NONE', #153214, #91911, #188449 ) ;
#143454=EDGE_CURVE ( 'NONE', #128093, #59419, #245834, .T. ) ;
#143460=VERTEX_POINT ( 'NONE', #188419 ) ;
#143465=DIRECTION ( 'NONE',  ( 1.000000000000000000, 0.000000000000000000, 0.000000000000000000 ) ) ;
#143486=CYLINDRICAL_SURFACE ( 'NONE', #114668, 0.09999999999999939493 ) ;
#143495=ORIENTED_EDGE ( 'NONE', *, *, #45938, .F. ) ;
#143512=EDGE_CURVE ( 'NONE', #96622, #208385, #232401, .T. ) ;
#143516=VERTEX_POINT ( 'NONE', #9785 ) ;
#143521=EDGE_LOOP ( 'NONE', ( #199313, #179182, #166401, #105421 ) ) ;
#143549=EDGE_CURVE ( 'NONE', #49099, #108030, #12383, .T. ) ;
#143551=CARTESIAN_POINT ( 'NONE',  ( -18.50000000000000000, 1.835341550224411922, -11.55515129256298046 ) ) ;
#143577=B_SPLINE_CURVE_WITH_KNOTS ( 'NONE', 3,
 ( #255185, #94879, #213540, #238242, #234387, #174485, #253944, #194009 ),
 .UNSPECIFIED., .F., .F.,
 ( 4, 2, 2, 4 ),
 ( 0.000000000000000000, 0.0002181133598168980686, 0.0003271700397253479026, 0.0004362267196337977094 ),
 .UNSPECIFIED. ) ;
#143582=DIRECTION ( 'NONE',  ( 0.000000000000000000, -1.000000000000000000, 0.000000000000000000 ) ) ;
#143612=CARTESIAN_POINT ( 'NONE',  ( 21.07946286933444568, 0.07668384325640636989, 6.329037319007706053 ) ) ;
#143681=CARTESIAN_POINT ( 'NONE',  ( -20.64999999999999858, 7.150000000000000355, -12.25000000000000000 ) ) ;
#143739=DIRECTION ( 'NONE',  ( 1.000000000000000000, -0.000000000000000000, -0.000000000000000000 ) ) ;
#143742=VERTEX_POINT ( 'NONE', #75521 ) ;
#143761=DIRECTION ( 'NONE',  ( 0.000000000000000000, 0.000000000000000000, 1.000000000000000000 ) ) ;
#143786=FACE_OUTER_BOUND ( 'NONE', #66234, .T. ) ;
#143798=EDGE_LOOP ( 'NONE', ( #244570, #184418, #97320, #66605 ) ) ;
#143804=ADVANCED_FACE ( 'NONE', ( #237140 ), #49205, .F. ) ;
#143834=EDGE_CURVE ( 'NONE', #171717, #214033, #186788, .T. ) ;
#143850=CIRCLE ( 'NONE', #189665, 7.900000000000000355 ) ;
#143874=CARTESIAN_POINT ( 'NONE',  ( -18.58222699835055280, 10.33200063079656417, -39.09316749566429650 ) ) ;
#143886=ORIENTED_EDGE ( 'NONE', *, *, #210509, .F. ) ;
#143900=FACE_OUTER_BOUND ( 'NONE', #5290, .T. ) ;
#143910=DIRECTION ( 'NONE',  ( 1.000000000000000000, 3.265361837132813093E-16, -0.000000000000000000 ) ) ;
#143987=CIRCLE ( 'NONE', #85517, 0.09999999999999939493 ) ;
#143995=ORIENTED_EDGE ( 'NONE', *, *, #198337, .F. ) ;
#144001=AXIS2_PLACEMENT_3D ( 'NONE', #50044, #129595, #90445 ) ;
#144002=AXIS2_PLACEMENT_3D ( 'NONE', #195908, #115070, #99327 ) ;
#144013=ORIENTED_EDGE ( 'NONE', *, *, #185994, .T. ) ;
#144029=DIRECTION ( 'NONE',  ( -1.836970198721029934E-16, 1.000000000000000000, 0.000000000000000000 ) ) ;
#144075=DIRECTION ( 'NONE',  ( 0.000000000000000000, -0.8660254037844411501, -0.4999999999999956146 ) ) ;
#144080=ORIENTED_EDGE ( 'NONE', *, *, #131049, .T. ) ;
#144081=CARTESIAN_POINT ( 'NONE',  ( 20.94999999999999929, 6.846123162352588665, -37.23772626684986164 ) ) ;
#144111=DIRECTION ( 'NONE',  ( 1.000000000000000000, 1.734723475976817507E-14, 0.000000000000000000 ) ) ;
#144137=CIRCLE ( 'NONE', #2686, 7.900000000000000355 ) ;
#144141=EDGE_CURVE ( 'NONE', #29243, #172615, #209566, .T. ) ;
#144161=DIRECTION ( 'NONE',  ( -0.000000000000000000, 1.000000000000000000, 1.734723475976807292E-15 ) ) ;
#144164=VERTEX_POINT ( 'NONE', #73935 ) ;
#144180=DIRECTION ( 'NONE',  ( 1.000000000000000000, 0.000000000000000000, -0.000000000000000000 ) ) ;
#144183=CARTESIAN_POINT ( 'NONE',  ( -23.15000000000000213, 0.000000000000000000, -33.50000000000000000 ) ) ;
#144191=VECTOR ( 'NONE', #225651, 1000.000000000000000 ) ;
#144226=LINE ( 'NONE', #103811, #86556 ) ;
#144256=CARTESIAN_POINT ( 'NONE',  ( 22.48660254037844197, 11.65000000000000746, 0.04999999999999796274 ) ) ;
#144264=AXIS2_PLACEMENT_3D ( 'NONE', #226282, #163780, #26857 ) ;
#144275=CARTESIAN_POINT ( 'NONE',  ( -18.47079683080347579, -9.471664105244876453, -7.108860540992417043 ) ) ;
#144292=LINE ( 'NONE', #126031, #127319 ) ;
#144303=CARTESIAN_POINT ( 'NONE',  ( -23.15000000000000213, 2.449293598294710359E-16, -35.50000000000000711 ) ) ;
#144308=VECTOR ( 'NONE', #158344, 1000.000000000000000 ) ;
#144309=CARTESIAN_POINT ( 'NONE',  ( -18.59999999999999787, 11.64999999999999680, -21.35000000000000142 ) ) ;
#144334=ADVANCED_FACE ( 'NONE', ( #240675 ), #747, .F. ) ;
#144336=VERTEX_POINT ( 'NONE', #226210 ) ;
#144338=FACE_OUTER_BOUND ( 'NONE', #119695, .T. ) ;
#144351=DIRECTION ( 'NONE',  ( 0.000000000000000000, 0.000000000000000000, -1.000000000000000000 ) ) ;
#144353=ORIENTED_EDGE ( 'NONE', *, *, #234532, .T. ) ;
#144375=EDGE_CURVE ( 'NONE', #112246, #210246, #223779, .T. ) ;
#144379=EDGE_CURVE ( 'NONE', #244468, #128093, #232691, .T. ) ;
#144381=ORIENTED_EDGE ( 'NONE', *, *, #52069, .T. ) ;
#144402=FACE_OUTER_BOUND ( 'NONE', #13237, .T. ) ;
#144403=DIRECTION ( 'NONE',  ( 0.000000000000000000, -1.000000000000000000, 0.000000000000000000 ) ) ;
#144407=EDGE_LOOP ( 'NONE', ( #79928, #4298, #153119, #154726, #248978 ) ) ;
#144423=DIRECTION ( 'NONE',  ( 0.000000000000000000, -0.9908441862701596881, -0.1350103645451904977 ) ) ;
#144438=CARTESIAN_POINT ( 'NONE',  ( -21.07016717456946253, 6.320940838100246317, -6.871554784600512487E-16 ) ) ;
#144439=ORIENTED_EDGE ( 'NONE', *, *, #185094, .T. ) ;
#144500=EDGE_CURVE ( 'NONE', #44319, #130475, #136105, .T. ) ;
#144533=DIRECTION ( 'NONE',  ( 0.000000000000000000, 0.000000000000000000, -1.000000000000000000 ) ) ;
#144583=CARTESIAN_POINT ( 'NONE',  ( 22.39999999999999503, -0.1008583690987139431, 11.74956712348939192 ) ) ;
#144600=CARTESIAN_POINT ( 'NONE',  ( 21.07016717456946608, 6.320940838100256975, -6.911788849595090767E-16 ) ) ;
#144617=DIRECTION ( 'NONE',  ( 0.000000000000000000, 0.8700118002898321601, -0.4930308989875230585 ) ) ;
#144618=CYLINDRICAL_SURFACE ( 'NONE', #224983, 11.80000000000000426 ) ;
#144644=DIRECTION ( 'NONE',  ( 0.000000000000000000, 1.000000000000000000, 0.000000000000000000 ) ) ;
#144659=CIRCLE ( 'NONE', #215399, 11.79999999999999893 ) ;
#144678=CARTESIAN_POINT ( 'NONE',  ( 19.94784844284954772, 11.71308993302901946, -24.70219871729859662 ) ) ;
#144684=AXIS2_PLACEMENT_3D ( 'NONE', #48551, #129376, #30289 ) ;
#144688=AXIS2_PLACEMENT_3D ( 'NONE', #17655, #97156, #176762 ) ;
#144762=CIRCLE ( 'NONE', #236935, 0.09999999999999939493 ) ;
#144794=VERTEX_POINT ( 'NONE', #74624 ) ;
#144795=ORIENTED_EDGE ( 'NONE', *, *, #82963, .F. ) ;
#144798=DIRECTION ( 'NONE',  ( 0.000000000000000000, 0.008583690987128059571, -0.9999631594459056361 ) ) ;
#144839=CARTESIAN_POINT ( 'NONE',  ( 18.50000000000000000, -9.399999999999998579, -7.297259759663296208 ) ) ;
#144849=CARTESIAN_POINT ( 'NONE',  ( -21.05000000000000071, 6.540656951701244282, 4.079310673976710433E-15 ) ) ;
#144875=CARTESIAN_POINT ( 'NONE',  ( -23.15000000000000213, 4.250000000000000000, -21.14999999999999858 ) ) ;
#144878=ORIENTED_EDGE ( 'NONE', *, *, #172376, .T. ) ;
#144887=AXIS2_PLACEMENT_3D ( 'NONE', #140810, #236051, #2958 ) ;
#144924=DIRECTION ( 'NONE',  ( 0.000000000000000000, 0.000000000000000000, -1.000000000000000000 ) ) ;
#144973=CYLINDRICAL_SURFACE ( 'NONE', #230711, 0.1000000000000010741 ) ;
#144984=DIRECTION ( 'NONE',  ( 0.000000000000000000, 0.000000000000000000, -1.000000000000000000 ) ) ;
#145023=ORIENTED_EDGE ( 'NONE', *, *, #249936, .F. ) ;
#145032=CIRCLE ( 'NONE', #49375, 11.65000000000000036 ) ;
#145060=DIRECTION ( 'NONE',  ( 1.000000000000000000, 0.000000000000000000, 0.000000000000000000 ) ) ;
#145078=CARTESIAN_POINT ( 'NONE',  ( -18.59999999999999787, 11.75000000000000000, -21.25000000000000000 ) ) ;
#145082=ORIENTED_EDGE ( 'NONE', *, *, #141677, .F. ) ;
#145083=DIRECTION ( 'NONE',  ( 1.000000000000000000, 0.000000000000000000, -0.000000000000000000 ) ) ;
#145143=LINE ( 'NONE', #43503, #162426 ) ;
#145144=ORIENTED_EDGE ( 'NONE', *, *, #160036, .T. ) ;
#145152=CARTESIAN_POINT ( 'NONE',  ( -18.54148534481894472, 10.32532329026770590, -39.06993430183596416 ) ) ;
#145163=DIRECTION ( 'NONE',  ( 0.000000000000000000, 0.000000000000000000, -1.000000000000000000 ) ) ;
#145176=DIRECTION ( 'NONE',  ( -1.000000000000000000, 0.000000000000000000, 0.000000000000000000 ) ) ;
#145222=VECTOR ( 'NONE', #250347, 1000.000000000000000 ) ;
#145230=VERTEX_POINT ( 'NONE', #109535 ) ;
#145237=EDGE_CURVE ( 'NONE', #172386, #131148, #148696, .T. ) ;
#145256=CARTESIAN_POINT ( 'NONE',  ( 22.60000000000000142, 0.1008583690987122083, 11.74956712348939192 ) ) ;
#145262=ORIENTED_EDGE ( 'NONE', *, *, #100240, .F. ) ;
#145270=ORIENTED_EDGE ( 'NONE', *, *, #195148, .T. ) ;
#145286=DIRECTION ( 'NONE',  ( -1.000000000000000000, 0.000000000000000000, 0.000000000000000000 ) ) ;
#145288=TOROIDAL_SURFACE ( 'NONE', #12048, 0.2000000000000000111, 0.1000000000000000056 ) ;
#145295=VECTOR ( 'NONE', #195853, 1000.000000000000000 ) ;
#145307=EDGE_LOOP ( 'NONE', ( #103374, #64622, #57997, #63299 ) ) ;
#145329=LINE ( 'NONE', #140182, #250854 ) ;
#145368=ORIENTED_EDGE ( 'NONE', *, *, #219105, .F. ) ;
#145397=CIRCLE ( 'NONE', #207795, 0.1000000000000008799 ) ;
#145409=ADVANCED_FACE ( 'NONE', ( #105015 ), #84157, .T. ) ;
#145414=CARTESIAN_POINT ( 'NONE',  ( 23.14999999999998437, 0.000000000000000000, 0.000000000000000000 ) ) ;
#145472=VECTOR ( 'NONE', #26248, 1000.000000000000000 ) ;
#145480=AXIS2_PLACEMENT_3D ( 'NONE', #72636, #188705, #71351 ) ;
#145482=ORIENTED_EDGE ( 'NONE', *, *, #31088, .T. ) ;
#145515=DIRECTION ( 'NONE',  ( -1.000000000000000000, 0.000000000000000000, 0.000000000000000000 ) ) ;
#145538=CARTESIAN_POINT ( 'NONE',  ( 18.59999999999999432, 1.736257131597397585, -11.56865232901749962 ) ) ;
#145544=PLANE ( 'NONE',  #115043 ) ;
#145554=ORIENTED_EDGE ( 'NONE', *, *, #167737, .F. ) ;
#145562=EDGE_CURVE ( 'NONE', #137697, #257538, #13667, .T. ) ;
#145563=CARTESIAN_POINT ( 'NONE',  ( 22.37643362114956247, 7.625789993958378865, 0.09908137368138185408 ) ) ;
#145578=CARTESIAN_POINT ( 'NONE',  ( -18.48550754432028143, -9.463399778559915987, -7.048789752415359544 ) ) ;
#145616=DIRECTION ( 'NONE',  ( 0.000000000000000000, 0.9998779222360100194, 0.01562499999998606150 ) ) ;
#145619=B_SPLINE_CURVE_WITH_KNOTS ( 'NONE', 3,
 ( #257920, #78043, #157636, #218830, #238412, #197989, #19372, #79315, #21944, #155060, #195465, #59744, #234559, #237133, #58463, #217543, #138008, #38943, #118482 ),
 .UNSPECIFIED., .F., .F.,
 ( 4, 3, 3, 3, 3, 3, 4 ),
 ( 0.000000000000000000, 1.655171619026035414E-05, 2.773500582848522787E-05, 5.941817267378589329E-05, 0.0001114174635873550078, 0.0001914169455916382733, 0.0002627181070750683224 ),
 .UNSPECIFIED. ) ;
#145691=DIRECTION ( 'NONE',  ( 0.000000000000000000, 0.000000000000000000, 1.000000000000000000 ) ) ;
#145702=ORIENTED_EDGE ( 'NONE', *, *, #180779, .T. ) ;
#145714=ORIENTED_EDGE ( 'NONE', *, *, #231246, .F. ) ;
#145715=ORIENTED_EDGE ( 'NONE', *, *, #62855, .F. ) ;
#145727=LINE ( 'NONE', #66212, #164043 ) ;
#145732=EDGE_LOOP ( 'NONE', ( #210153, #41522, #54467, #85943 ) ) ;
#145748=VERTEX_POINT ( 'NONE', #39678 ) ;
#145783=ADVANCED_FACE ( 'NONE', ( #80020 ), #176613, .F. ) ;
#145797=DIRECTION ( 'NONE',  ( 0.000000000000000000, 0.000000000000000000, 1.000000000000000000 ) ) ;
#145810=ORIENTED_EDGE ( 'NONE', *, *, #193771, .F. ) ;
#145818=CARTESIAN_POINT ( 'NONE',  ( 20.94999999999999574, -1.162701749938009677, -8.099999999999999645 ) ) ;
#145839=DIRECTION ( 'NONE',  ( 0.000000000000000000, -4.336808689942043768E-15, 1.000000000000000000 ) ) ;
#145840=EDGE_CURVE ( 'NONE', #133804, #96700, #103450, .T. ) ;
#145862=CARTESIAN_POINT ( 'NONE',  ( 21.05000000000000071, 4.999999999999997335, -21.59473398108690390 ) ) ;
#145871=DIRECTION ( 'NONE',  ( 1.000000000000000000, 0.000000000000000000, 0.000000000000000000 ) ) ;
#145905=FACE_OUTER_BOUND ( 'NONE', #64295, .T. ) ;
#145931=DIRECTION ( 'NONE',  ( 0.000000000000000000, -0.4999999999999929501, -0.8660254037844427044 ) ) ;
#145958=CIRCLE ( 'NONE', #162560, 0.1000000000000001860 ) ;
#145962=ORIENTED_EDGE ( 'NONE', *, *, #123182, .F. ) ;
#145966=CARTESIAN_POINT ( 'NONE',  ( 19.75857864376269291, 11.75000000000000533, -24.75000000000000000 ) ) ;
#145971=ORIENTED_EDGE ( 'NONE', *, *, #184376, .F. ) ;
#146005=DIRECTION ( 'NONE',  ( -1.000000000000000000, 0.000000000000000000, 0.000000000000000000 ) ) ;
#146025=CARTESIAN_POINT ( 'NONE',  ( -23.15000000000000213, 1.925233644859811521, -20.76975646687386501 ) ) ;
#146034=FACE_OUTER_BOUND ( 'NONE', #200539, .T. ) ;
#146052=CARTESIAN_POINT ( 'NONE',  ( 18.59999999999999076, 6.450000000000001066, -21.15000000000000213 ) ) ;
#146057=AXIS2_PLACEMENT_3D ( 'NONE', #25102, #241551, #26366 ) ;
#146086=CIRCLE ( 'NONE', #233592, 0.1000000000000028644 ) ;
#146094=VECTOR ( 'NONE', #152186, 1000.000000000000000 ) ;
#146109=AXIS2_PLACEMENT_3D ( 'NONE', #242071, #82969, #102531 ) ;
#146125=CARTESIAN_POINT ( 'NONE',  ( -21.05000000000000071, -0.02110330805904066936, 6.304516329263973873 ) ) ;
#146130=CARTESIAN_POINT ( 'NONE',  ( -20.85000000000000142, 0.000000000000000000, -33.50000000000000000 ) ) ;
#146139=CARTESIAN_POINT ( 'NONE',  ( -21.13435531349809082, 6.493721063592104770, 4.741518362104077497E-16 ) ) ;
#146143=EDGE_CURVE ( 'NONE', #111006, #253599, #257979, .T. ) ;
#146194=CARTESIAN_POINT ( 'NONE',  ( -20.54999999999999716, 1.999999999999998224, -13.22462192276210224 ) ) ;
#146226=ORIENTED_EDGE ( 'NONE', *, *, #178612, .F. ) ;
#146235=TOROIDAL_SURFACE ( 'NONE', #225340, 1.900000000000002576, 0.1000000000000000056 ) ;
#146246=CARTESIAN_POINT ( 'NONE',  ( -23.15000000000000213, -9.000000000000003553, -9.893969122652444881 ) ) ;
#146287=AXIS2_PLACEMENT_3D ( 'NONE', #75012, #249771, #213192 ) ;
#146322=ORIENTED_EDGE ( 'NONE', *, *, #234840, .T. ) ;
#146328=ORIENTED_EDGE ( 'NONE', *, *, #94918, .F. ) ;
#146345=DIRECTION ( 'NONE',  ( 0.000000000000000000, 1.000000000000000000, 0.000000000000000000 ) ) ;
#146393=DIRECTION ( 'NONE',  ( 0.000000000000000000, 0.000000000000000000, -1.000000000000000000 ) ) ;
#146427=EDGE_CURVE ( 'NONE', #240172, #87594, #158298, .T. ) ;
#146429=DIRECTION ( 'NONE',  ( 0.000000000000000000, 0.000000000000000000, -1.000000000000000000 ) ) ;
#146462=B_SPLINE_CURVE_WITH_KNOTS ( 'NONE', 3,
 ( #13977, #93492, #173090, #252558 ),
 .UNSPECIFIED., .F., .F.,
 ( 4, 4 ),
 ( 0.000000000000000000, 0.001767853679387130974 ),
 .UNSPECIFIED. ) ;
#146466=ORIENTED_EDGE ( 'NONE', *, *, #221273, .F. ) ;
#146508=CYLINDRICAL_SURFACE ( 'NONE', #34372, 0.09999999999999939493 ) ;
#146531=AXIS2_PLACEMENT_3D ( 'NONE', #205863, #32402, #194033 ) ;
#146581=CARTESIAN_POINT ( 'NONE',  ( 20.94999999999999929, -11.39257802170566869, -30.42605042016806394 ) ) ;
#146582=DIRECTION ( 'NONE',  ( -1.000000000000000000, -1.836970198721029934E-16, 0.000000000000000000 ) ) ;
#146587=CIRCLE ( 'NONE', #79936, 0.09999999999999939493 ) ;
#146614=CARTESIAN_POINT ( 'NONE',  ( -21.05000000000000071, -1.851028230140860487, -11.65391326942249428 ) ) ;
#146625=ADVANCED_FACE ( 'NONE', ( #41635 ), #200693, .T. ) ;
#146696=EDGE_CURVE ( 'NONE', #219800, #178493, #145958, .T. ) ;
#146732=ORIENTED_EDGE ( 'NONE', *, *, #172376, .F. ) ;
#146740=EDGE_CURVE ( 'NONE', #5738, #124163, #45462, .T. ) ;
#146745=ORIENTED_EDGE ( 'NONE', *, *, #154731, .F. ) ;
#146748=EDGE_CURVE ( 'NONE', #243446, #234900, #85838, .T. ) ;
#146767=VERTEX_POINT ( 'NONE', #88413 ) ;
#146780=CYLINDRICAL_SURFACE ( 'NONE', #117624, 0.09999999999999920064 ) ;
#146797=EDGE_CURVE ( 'NONE', #176380, #193155, #150094, .T. ) ;
#146799=LINE ( 'NONE', #185949, #245136 ) ;
#146801=DIRECTION ( 'NONE',  ( 1.000000000000000000, 0.000000000000000000, 0.000000000000000000 ) ) ;
#146802=EDGE_CURVE ( 'NONE', #94835, #113369, #29792, .T. ) ;
#146803=EDGE_CURVE ( 'NONE', #198340, #32767, #137569, .T. ) ;
#146805=CARTESIAN_POINT ( 'NONE',  ( 20.94983749550516450, 10.29766095124176850, -38.97436639332756414 ) ) ;
#146809=CARTESIAN_POINT ( 'NONE',  ( -23.15000000000000213, 0.000000000000000000, -29.50000000000000355 ) ) ;
#146832=DIRECTION ( 'NONE',  ( 0.000000000000000000, 0.000000000000000000, -1.000000000000000000 ) ) ;
#146847=LINE ( 'NONE', #6064, #61342 ) ;
#146868=DIRECTION ( 'NONE',  ( 1.000000000000000000, 7.304098846218134667E-16, -0.000000000000000000 ) ) ;
#146917=ORIENTED_EDGE ( 'NONE', *, *, #153372, .F. ) ;
#146932=CARTESIAN_POINT ( 'NONE',  ( -21.00448002041601114, 11.75000000000000000, -6.848340862310549504 ) ) ;
#146938=CARTESIAN_POINT ( 'NONE',  ( -21.05000000000000071, -1.835341550224411922, -11.55515129256297868 ) ) ;
#146941=CARTESIAN_POINT ( 'NONE',  ( -18.39999999999999858, -9.600000000000001421, -7.032069396699667685 ) ) ;
#146947=ORIENTED_EDGE ( 'NONE', *, *, #241130, .F. ) ;
#146957=DIRECTION ( 'NONE',  ( 1.000000000000000000, 0.000000000000000000, -0.000000000000000000 ) ) ;
#146959=VERTEX_POINT ( 'NONE', #144081 ) ;
#146971=CARTESIAN_POINT ( 'NONE',  ( -20.64999999999999858, 4.349999999999999645, -21.14999999999999858 ) ) ;
#146991=ORIENTED_EDGE ( 'NONE', *, *, #137013, .T. ) ;
#147008=LINE ( 'NONE', #227839, #59208 ) ;
#147016=ORIENTED_EDGE ( 'NONE', *, *, #71783, .T. ) ;
#147033=FACE_OUTER_BOUND ( 'NONE', #205033, .T. ) ;
#147053=TOROIDAL_SURFACE ( 'NONE', #34664, 0.6000000000000006439, 0.1000000000000000056 ) ;
#147079=DIRECTION ( 'NONE',  ( -1.000000000000000000, -2.952720810173289112E-16, 0.000000000000000000 ) ) ;
#147089=EDGE_CURVE ( 'NONE', #40483, #156131, #252180, .T. ) ;
#147122=AXIS2_PLACEMENT_3D ( 'NONE', #24032, #25319, #200084 ) ;
#147130=EDGE_CURVE ( 'NONE', #135192, #162626, #112832, .T. ) ;
#147138=EDGE_CURVE ( 'NONE', #87594, #63693, #254713, .T. ) ;
#147139=ORIENTED_EDGE ( 'NONE', *, *, #233995, .T. ) ;
#147191=EDGE_CURVE ( 'NONE', #170111, #170516, #255991, .T. ) ;
#147221=FACE_OUTER_BOUND ( 'NONE', #143281, .T. ) ;
#147228=CARTESIAN_POINT ( 'NONE',  ( 23.14999999999999858, -3.999999999999999112, -33.50000000000000000 ) ) ;
#147260=CARTESIAN_POINT ( 'NONE',  ( -21.05000000000000071, 1.249999999999999334, -8.000000000000000000 ) ) ;
#147351=DIRECTION ( 'NONE',  ( 1.000000000000000000, 0.000000000000000000, 0.000000000000000000 ) ) ;
#147365=CYLINDRICAL_SURFACE ( 'NONE', #148399, 0.09999999999999939493 ) ;
#147383=ORIENTED_EDGE ( 'NONE', *, *, #138194, .T. ) ;
#147401=AXIS2_PLACEMENT_3D ( 'NONE', #206899, #28297, #249876 ) ;
#147402=CIRCLE ( 'NONE', #35013, 0.09999999999999939493 ) ;
#147409=B_SPLINE_CURVE_WITH_KNOTS ( 'NONE', 3,
 ( #152730, #212680, #227082, #52285, #113567, #193119, #79554, #237372, #194415, #178713, #99111, #39195, #233533, #198229, #95285, #117423, #114849, #234803, #17055 ),
 .UNSPECIFIED., .F., .F.,
 ( 4, 3, 3, 3, 3, 3, 4 ),
 ( 0.000000000000000000, 7.110282409889887435E-05, 0.0001508797727291436692, 0.0002027344179858470120, 0.0002343294522349037394, 0.0002454816334821225830, 0.0002619873080085598845 ),
 .UNSPECIFIED. ) ;
#147415=DIRECTION ( 'NONE',  ( 1.000000000000000000, 0.000000000000000000, 0.000000000000000000 ) ) ;
#147416=CARTESIAN_POINT ( 'NONE',  ( -21.07928932188134397, 0.09889514565439470883, 6.328516656393301076 ) ) ;
#147440=CARTESIAN_POINT ( 'NONE',  ( -18.49499033040907037, -9.438148771744673482, -7.198153225923435095 ) ) ;
#147456=DIRECTION ( 'NONE',  ( -0.000000000000000000, -1.000000000000000000, -0.000000000000000000 ) ) ;
#147470=EDGE_CURVE ( 'NONE', #240969, #53603, #252229, .T. ) ;
#147478=DIRECTION ( 'NONE',  ( 0.000000000000000000, 0.000000000000000000, 1.000000000000000000 ) ) ;
#147482=AXIS2_PLACEMENT_3D ( 'NONE', #19972, #194765, #94338 ) ;
#147490=CIRCLE ( 'NONE', #5813, 0.09999999999999939493 ) ;
#147515=VERTEX_POINT ( 'NONE', #231959 ) ;
#147530=EDGE_LOOP ( 'NONE', ( #177446, #13865, #18726, #28977, #154772 ) ) ;
#147537=VECTOR ( 'NONE', #89455, 1000.000000000000000 ) ;
#147544=ORIENTED_EDGE ( 'NONE', *, *, #212414, .F. ) ;
#147552=ORIENTED_EDGE ( 'NONE', *, *, #154764, .T. ) ;
#147612=AXIS2_PLACEMENT_3D ( 'NONE', #84393, #2327, #1027 ) ;
#147616=CIRCLE ( 'NONE', #197492, 0.09999999999999761857 ) ;
#147619=ORIENTED_EDGE ( 'NONE', *, *, #194647, .F. ) ;
#147671=VERTEX_POINT ( 'NONE', #136666 ) ;
#147678=EDGE_CURVE ( 'NONE', #52039, #158841, #48232, .T. ) ;
#147706=AXIS2_PLACEMENT_3D ( 'NONE', #120652, #1941, #181892 ) ;
#147783=CARTESIAN_POINT ( 'NONE',  ( 20.94999999999999929, 11.65000000000000391, -26.71613433702190932 ) ) ;
#147791=ORIENTED_EDGE ( 'NONE', *, *, #185094, .F. ) ;
#147841=EDGE_CURVE ( 'NONE', #52704, #210905, #156616, .T. ) ;
#147847=TOROIDAL_SURFACE ( 'NONE', #189347, 0.2000000000000000111, 0.1000000000000000056 ) ;
#147849=CARTESIAN_POINT ( 'NONE',  ( -20.94999999999999929, 0.000000000000000000, -33.50000000000000000 ) ) ;
#147850=ORIENTED_EDGE ( 'NONE', *, *, #169308, .T. ) ;
#147867=CIRCLE ( 'NONE', #35462, 0.09999999999999939493 ) ;
#147891=CIRCLE ( 'NONE', #177126, 2.000000000000001776 ) ;
#147895=EDGE_CURVE ( 'NONE', #227236, #29243, #131234, .T. ) ;
#147935=ORIENTED_EDGE ( 'NONE', *, *, #208134, .F. ) ;
#147950=AXIS2_PLACEMENT_3D ( 'NONE', #128920, #45524, #6390 ) ;
#147954=CARTESIAN_POINT ( 'NONE',  ( 21.05000000000000071, 0.09779029130879170195, 6.257814610476124528 ) ) ;
#147979=CARTESIAN_POINT ( 'NONE',  ( -21.65000000000000213, 7.750000000000000000, -12.34999999999999964 ) ) ;
#147995=ADVANCED_FACE ( 'NONE', ( #133798 ), #135067, .T. ) ;
#147999=DIRECTION ( 'NONE',  ( 0.000000000000000000, 0.000000000000000000, -1.000000000000000000 ) ) ;
#148018=LINE ( 'NONE', #199342, #111102 ) ;
#148021=DIRECTION ( 'NONE',  ( 1.296989514748957922E-15, -0.9887567792719341719, 0.1495327102803664099 ) ) ;
#148054=EDGE_LOOP ( 'NONE', ( #178692, #243007, #115627, #241151 ) ) ;
#148069=ORIENTED_EDGE ( 'NONE', *, *, #58820, .F. ) ;
#148099=ORIENTED_EDGE ( 'NONE', *, *, #146803, .F. ) ;
#148151=CARTESIAN_POINT ( 'NONE',  ( -22.48970261584618058, 11.65000000000000036, 0.05536948821740890481 ) ) ;
#148159=FACE_OUTER_BOUND ( 'NONE', #167317, .T. ) ;
#148163=AXIS2_PLACEMENT_3D ( 'NONE', #133998, #213529, #75349 ) ;
#148198=CARTESIAN_POINT ( 'NONE',  ( 22.39999999999999858, 7.790779598373383408, 0.09999999999999939493 ) ) ;
#148225=CARTESIAN_POINT ( 'NONE',  ( 23.14999999999999503, 6.450000000000001066, 11.75000000000000000 ) ) ;
#148232=CARTESIAN_POINT ( 'NONE',  ( -20.94999999999999929, 11.59999999999999787, -6.928203230275557623 ) ) ;
#148270=ORIENTED_EDGE ( 'NONE', *, *, #130095, .T. ) ;
#148305=CARTESIAN_POINT ( 'NONE',  ( -20.85000000000000142, -1.164121893241208960, -41.31484808557160449 ) ) ;
#148323=CARTESIAN_POINT ( 'NONE',  ( -18.59999999999999787, 11.64999999999999680, -7.014805770653998351 ) ) ;
#148329=ORIENTED_EDGE ( 'NONE', *, *, #28283, .T. ) ;
#148392=CARTESIAN_POINT ( 'NONE',  ( 21.05095171578076574, 8.776179878771037224, -12.16587327663788187 ) ) ;
#148397=CIRCLE ( 'NONE', #160871, 11.90000000000000213 ) ;
#148399=AXIS2_PLACEMENT_3D ( 'NONE', #32595, #9144, #209923 ) ;
#148415=ORIENTED_EDGE ( 'NONE', *, *, #25635, .T. ) ;
#148417=CARTESIAN_POINT ( 'NONE',  ( 22.39999999999999503, 0.000000000000000000, 7.790779598373379855 ) ) ;
#148419=CARTESIAN_POINT ( 'NONE',  ( -18.50000000000000000, -1.164121893241208960, -41.41484808557160591 ) ) ;
#148420=CARTESIAN_POINT ( 'NONE',  ( 18.59999999999999432, 1.637172712970381694, -11.58215336547201879 ) ) ;
#148436=CARTESIAN_POINT ( 'NONE',  ( 21.04999999999999716, 10.62872031400434913, -12.15000000000000036 ) ) ;
#148467=FACE_OUTER_BOUND ( 'NONE', #115741, .T. ) ;
#148512=ORIENTED_EDGE ( 'NONE', *, *, #17181, .T. ) ;
#148537=CARTESIAN_POINT ( 'NONE',  ( -20.54999999999999716, 0.000000000000000000, -33.50000000000000000 ) ) ;
#148584=CARTESIAN_POINT ( 'NONE',  ( -22.49533356619861379, 11.65000000630418597, 0.06512258032272708053 ) ) ;
#148585=SPHERICAL_SURFACE ( 'NONE', #221785, 0.1000000000000000056 ) ;
#148594=CIRCLE ( 'NONE', #2815, 11.74999999999999645 ) ;
#148657=ORIENTED_EDGE ( 'NONE', *, *, #157742, .T. ) ;
#148682=ORIENTED_EDGE ( 'NONE', *, *, #139074, .T. ) ;
#148692=DIRECTION ( 'NONE',  ( 0.000000000000000000, 0.000000000000000000, -1.000000000000000000 ) ) ;
#148696=LINE ( 'NONE', #189094, #145222 ) ;
#148715=CARTESIAN_POINT ( 'NONE',  ( -21.05000000000000071, -0.08579911627410685693, 6.413978881488484163 ) ) ;
#148749=VECTOR ( 'NONE', #11477, 1000.000000000000000 ) ;
#148790=LINE ( 'NONE', #30137, #49320 ) ;
#148798=EDGE_LOOP ( 'NONE', ( #225478, #71618, #140057, #129584, #140998, #39916, #136610, #115492, #17481, #147016, #76495 ) ) ;
#148799=CYLINDRICAL_SURFACE ( 'NONE', #255829, 0.09999999999999939493 ) ;
#148838=VERTEX_POINT ( 'NONE', #195134 ) ;
#148879=CARTESIAN_POINT ( 'NONE',  ( 18.39999999999999858, -9.600000000000003197, -40.10018939122204529 ) ) ;
#148886=EDGE_CURVE ( 'NONE', #227165, #13242, #69649, .T. ) ;
#148903=EDGE_LOOP ( 'NONE', ( #190746, #67189, #207211, #85886 ) ) ;
#148907=CARTESIAN_POINT ( 'NONE',  ( 21.05000000000000071, -0.09999999999999939493, 11.64957080754479968 ) ) ;
#148936=ORIENTED_EDGE ( 'NONE', *, *, #227151, .F. ) ;
#148942=ORIENTED_EDGE ( 'NONE', *, *, #245976, .T. ) ;
#148950=CARTESIAN_POINT ( 'NONE',  ( -20.64999999999999858, 4.349999999999999645, -12.25000000000000000 ) ) ;
#148955=AXIS2_PLACEMENT_3D ( 'NONE', #168183, #230689, #109427 ) ;
#148985=CIRCLE ( 'NONE', #45091, 0.1000000000000000056 ) ;
#149002=TOROIDAL_SURFACE ( 'NONE', #36594, 0.2000000000000000111, 0.1000000000000000056 ) ;
#149006=DIRECTION ( 'NONE',  ( 0.000000000000000000, 0.000000000000000000, -1.000000000000000000 ) ) ;
#149010=ORIENTED_EDGE ( 'NONE', *, *, #176528, .F. ) ;
#149051=DIRECTION ( 'NONE',  ( 1.000000000000000000, -0.000000000000000000, -0.000000000000000000 ) ) ;
#149076=CARTESIAN_POINT ( 'NONE',  ( 20.99551997958397109, 11.75000000000023626, -26.65165913768949579 ) ) ;
#149127=ORIENTED_EDGE ( 'NONE', *, *, #89079, .F. ) ;
#149155=ADVANCED_FACE ( 'NONE', ( #21615 ), #44702, .T. ) ;
#149161=CARTESIAN_POINT ( 'NONE',  ( 23.24999999999999645, 0.000000000000000000, -33.50000000000000000 ) ) ;
#149189=CIRCLE ( 'NONE', #94989, 0.09999999999999939493 ) ;
#149191=EDGE_CURVE ( 'NONE', #116070, #184680, #128084, .T. ) ;
#149219=CARTESIAN_POINT ( 'NONE',  ( -20.85000000000000142, 0.1610488207187191212, -33.21581015563977957 ) ) ;
#149252=ADVANCED_FACE ( 'NONE', ( #167563 ), #185810, .T. ) ;
#149254=DIRECTION ( 'NONE',  ( 7.304098846218134667E-16, -1.000000000000000000, 0.000000000000000000 ) ) ;
#149283=DIRECTION ( 'NONE',  ( -6.938893903907222856E-15, 1.000000000000000000, 2.891205793294679805E-16 ) ) ;
#149287=CYLINDRICAL_SURFACE ( 'NONE', #164718, 3.999999999999996447 ) ;
#149288=EDGE_CURVE ( 'NONE', #174236, #248548, #130979, .T. ) ;
#149335=B_SPLINE_CURVE_WITH_KNOTS ( 'NONE', 3,
 ( #158119, #21160, #257117, #100625, #61542, #240190 ),
 .UNSPECIFIED., .F., .F.,
 ( 4, 2, 4 ),
 ( 0.000000000000000000, 0.0001497467027049230307, 0.0002994934054098460615 ),
 .UNSPECIFIED. ) ;
#149362=DIRECTION ( 'NONE',  ( -1.000000000000000000, -7.304098846218135653E-16, 4.607487905232624742E-31 ) ) ;
#149366=VECTOR ( 'NONE', #187842, 1000.000000000000000 ) ;
#149373=EDGE_CURVE ( 'NONE', #158624, #136985, #82435, .T. ) ;
#149380=DIRECTION ( 'NONE',  ( 0.000000000000000000, 0.000000000000000000, -1.000000000000000000 ) ) ;
#149384=SPHERICAL_SURFACE ( 'NONE', #87286, 0.1000000000000000056 ) ;
#149385=CARTESIAN_POINT ( 'NONE',  ( 22.39999999999999503, 11.65000000000000746, 0.09999999999999592548 ) ) ;
#149394=CARTESIAN_POINT ( 'NONE',  ( 19.58285714285715073, 10.38499851035142107, -7.629684667389950548 ) ) ;
#149397=DIRECTION ( 'NONE',  ( 0.000000000000000000, -1.000000000000000000, 0.000000000000000000 ) ) ;
#149418=CARTESIAN_POINT ( 'NONE',  ( -18.50000000000000000, 0.000000000000000000, 0.000000000000000000 ) ) ;
#149422=FACE_OUTER_BOUND ( 'NONE', #255263, .T. ) ;
#149469=DIRECTION ( 'NONE',  ( 1.000000000000000000, 0.000000000000000000, -0.000000000000000000 ) ) ;
#149476=AXIS2_PLACEMENT_3D ( 'NONE', #59922, #139469, #199480 ) ;
#149534=CARTESIAN_POINT ( 'NONE',  ( -22.39999999999999858, 7.790779598373403836, 0.09999999999999939493 ) ) ;
#149583=DIRECTION ( 'NONE',  ( 0.000000000000000000, -3.469446951953611033E-15, -1.000000000000000000 ) ) ;
#149610=TOROIDAL_SURFACE ( 'NONE', #37186, 4.149999999999999467, 0.1000000000000000056 ) ;
#149625=ORIENTED_EDGE ( 'NONE', *, *, #191687, .F. ) ;
#149632=CARTESIAN_POINT ( 'NONE',  ( -23.15000000000000213, 4.898587196589414801E-16, -37.50000000000000000 ) ) ;
#149661=FACE_OUTER_BOUND ( 'NONE', #86692, .T. ) ;
#149667=LINE ( 'NONE', #154809, #155349 ) ;
#149670=CARTESIAN_POINT ( 'NONE',  ( 18.59999999999999432, -1.835859311443640340, -45.00443916879852679 ) ) ;
#149686=ORIENTED_EDGE ( 'NONE', *, *, #212414, .T. ) ;
#149692=ADVANCED_FACE ( 'NONE', ( #5562 ), #90826, .T. ) ;
#149718=CARTESIAN_POINT ( 'NONE',  ( 21.14999999999999858, 0.000000000000000000, 6.540656951701244282 ) ) ;
#149727=CARTESIAN_POINT ( 'NONE',  ( 21.05000000000000071, 5.021051876504147385E-16, -29.40000000000000213 ) ) ;
#149738=CARTESIAN_POINT ( 'NONE',  ( -23.25000000000000000, 1.910280373831774847, -20.86863214480106166 ) ) ;
#149748=AXIS2_PLACEMENT_3D ( 'NONE', #11080, #192291, #168911 ) ;
#149764=CARTESIAN_POINT ( 'NONE',  ( -18.59999999999999787, -9.500000000000005329, -8.099999999999999645 ) ) ;
#149784=VECTOR ( 'NONE', #161529, 1000.000000000000000 ) ;
#149792=CARTESIAN_POINT ( 'NONE',  ( -18.37151313414685561, -9.571014125778372517, -40.31666290923867280 ) ) ;
#149798=CARTESIAN_POINT ( 'NONE',  ( -20.94999999999999929, -1.849153571976047239, -45.10596661979705146 ) ) ;
#149846=CARTESIAN_POINT ( 'NONE',  ( 18.48197441911561612, -9.517954794705673294, -40.39021164220778104 ) ) ;
#149857=CARTESIAN_POINT ( 'NONE',  ( 21.14999999999999858, 0.000000000000000000, -12.15000000000000036 ) ) ;
#149887=CARTESIAN_POINT ( 'NONE',  ( 21.05000000000000071, 6.649999999999999467, -10.01702717044001822 ) ) ;
#149903=DIRECTION ( 'NONE',  ( 0.000000000000000000, -1.000000000000000000, 0.000000000000000000 ) ) ;
#149922=DIRECTION ( 'NONE',  ( 0.000000000000000000, 0.000000000000000000, -1.000000000000000000 ) ) ;
#149950=( BOUNDED_CURVE ( )  B_SPLINE_CURVE ( 3, ( #7277, #149394, #108944, #45131 ),
 .UNSPECIFIED., .F., .F. ) 
 B_SPLINE_CURVE_WITH_KNOTS ( ( 4, 4 ),
 ( 0.06456096931748320222, 3.077031684272310219 ),
 .UNSPECIFIED. ) 
 CURVE ( )  GEOMETRIC_REPRESENTATION_ITEM ( )  RATIONAL_B_SPLINE_CURVE ( ( 1.000000000000000000, 0.3763440860215094830, 0.3763440860215094830, 1.000000000000000000 ) ) 
 REPRESENTATION_ITEM ( '' )  );
#149953=CARTESIAN_POINT ( 'NONE',  ( 21.14999999999999858, 0.09779029130879170195, 6.257814610476124528 ) ) ;
#149956=DIRECTION ( 'NONE',  ( 0.000000000000000000, 0.000000000000000000, -1.000000000000000000 ) ) ;
#149964=DIRECTION ( 'NONE',  ( 0.000000000000000000, 0.000000000000000000, 1.000000000000000000 ) ) ;
#149982=DIRECTION ( 'NONE',  ( -1.000000000000000000, 0.000000000000000000, 0.000000000000000000 ) ) ;
#150010=CARTESIAN_POINT ( 'NONE',  ( -21.05000000000000071, 0.03175835305540354592, 6.258847123079506858 ) ) ;
#150021=AXIS2_PLACEMENT_3D ( 'NONE', #143255, #238509, #182403 ) ;
#150024=CARTESIAN_POINT ( 'NONE',  ( -21.15000000000000213, 6.540656951701243393, 6.098637220230962441E-16 ) ) ;
#150047=FACE_OUTER_BOUND ( 'NONE', #87351, .T. ) ;
#150053=AXIS2_PLACEMENT_3D ( 'NONE', #95163, #174749, #196820 ) ;
#150075=EDGE_CURVE ( 'NONE', #141594, #4508, #94543, .T. ) ;
#150084=CARTESIAN_POINT ( 'NONE',  ( -20.64999999999999858, 7.150000000000000355, -21.15000000000000213 ) ) ;
#150093=ORIENTED_EDGE ( 'NONE', *, *, #125577, .F. ) ;
#150094=CIRCLE ( 'NONE', #4300, 0.09999999999999939493 ) ;
#150108=VERTEX_POINT ( 'NONE', #255385 ) ;
#150113=LINE ( 'NONE', #112265, #163829 ) ;
#150128=AXIS2_PLACEMENT_3D ( 'NONE', #111030, #58731, #100425 ) ;
#150148=CARTESIAN_POINT ( 'NONE',  ( 23.25000000000000000, -11.74999999999999112, -12.15000000000000036 ) ) ;
#150154=TOROIDAL_SURFACE ( 'NONE', #216761, 11.90000000000000391, 0.1000000000000000056 ) ;
#150159=EDGE_CURVE ( 'NONE', #114284, #139879, #94445, .T. ) ;
#150167=DIRECTION ( 'NONE',  ( 0.000000000000000000, 1.000000000000000000, 0.000000000000000000 ) ) ;
#150168=ORIENTED_EDGE ( 'NONE', *, *, #252743, .T. ) ;
#150186=B_SPLINE_CURVE_WITH_KNOTS ( 'NONE', 3,
 ( #84003, #226110, #22830, #1932, #163606, #82736, #166205, #47483, #220988, #25393, #206578, #222255, #184438, #27979, #81456, #5781, #161040, #42366, #181882 ),
 .UNSPECIFIED., .F., .F.,
 ( 4, 3, 3, 3, 3, 3, 4 ),
 ( -2.000416914656963086E-06, 0.000000000000000000, 4.714008503746661030E-05, 9.979203887778580651E-05, 0.0001372215519229558309, 0.0001635031576221024189, 0.0001900083748504180947 ),
 .UNSPECIFIED. ) ;
#150198=DIRECTION ( 'NONE',  ( 0.000000000000000000, 0.000000000000000000, -1.000000000000000000 ) ) ;
#150200=ORIENTED_EDGE ( 'NONE', *, *, #17698, .T. ) ;
#150204=EDGE_CURVE ( 'NONE', #106325, #62255, #36316, .T. ) ;
#150225=DIRECTION ( 'NONE',  ( -1.000000000000000000, -3.265361837132813093E-16, 0.000000000000000000 ) ) ;
#150245=DIRECTION ( 'NONE',  ( 1.000000000000000000, 0.000000000000000000, 0.000000000000000000 ) ) ;
#150254=ORIENTED_EDGE ( 'NONE', *, *, #251362, .F. ) ;
#150301=CYLINDRICAL_SURFACE ( 'NONE', #116495, 2.000000000000001776 ) ;
#150326=FACE_OUTER_BOUND ( 'NONE', #106668, .T. ) ;
#150354=AXIS2_PLACEMENT_3D ( 'NONE', #82044, #24708, #65083 ) ;
#150376=VERTEX_POINT ( 'NONE', #28427 ) ;
#150421=VECTOR ( 'NONE', #104468, 1000.000000000000000 ) ;
#150423=CIRCLE ( 'NONE', #204557, 0.09999999999999939493 ) ;
#150455=FACE_OUTER_BOUND ( 'NONE', #51126, .T. ) ;
#150460=PLANE ( 'NONE',  #13028 ) ;
#150464=DIRECTION ( 'NONE',  ( 0.000000000000000000, 0.000000000000000000, -1.000000000000000000 ) ) ;
#150524=CARTESIAN_POINT ( 'NONE',  ( 20.94999999999999574, 10.42338541491290727, -7.492051923870097774 ) ) ;
#150528=CARTESIAN_POINT ( 'NONE',  ( -18.59999999999999787, -1.162701749938009677, -8.000000000000000000 ) ) ;
#150558=AXIS2_PLACEMENT_3D ( 'NONE', #149857, #71606, #152436 ) ;
#150562=AXIS2_PLACEMENT_3D ( 'NONE', #52410, #90250, #172423 ) ;
#150594=CARTESIAN_POINT ( 'NONE',  ( 21.05000000000000071, -1.835341550224413698, -11.55515129256298046 ) ) ;
#150608=DIRECTION ( 'NONE',  ( -1.000000000000000000, -2.952720810173289112E-16, 0.000000000000000000 ) ) ;
#150614=CARTESIAN_POINT ( 'NONE',  ( 18.52928932188133970, 10.27928932188134858, -24.75000000000000000 ) ) ;
#150617=CARTESIAN_POINT ( 'NONE',  ( 23.24999999999999289, 6.550000000000000711, -21.35000000000000142 ) ) ;
#150654=CARTESIAN_POINT ( 'NONE',  ( 23.24999999999999645, 5.599999999999996980, -21.09473398108690390 ) ) ;
#150657=ORIENTED_EDGE ( 'NONE', *, *, #221247, .F. ) ;
#150680=ORIENTED_EDGE ( 'NONE', *, *, #189408, .F. ) ;
#150686=EDGE_CURVE ( 'NONE', #184931, #109469, #107388, .T. ) ;
#150696=FACE_OUTER_BOUND ( 'NONE', #65795, .T. ) ;
#150704=CARTESIAN_POINT ( 'NONE',  ( -23.15000000000000213, -11.41227409414968541, -30.50000000000000000 ) ) ;
#150711=EDGE_CURVE ( 'NONE', #129010, #110550, #98992, .T. ) ;
#150712=CARTESIAN_POINT ( 'NONE',  ( 21.07928932188134397, 6.328516656393303741, 0.09889514565439641580 ) ) ;
#150721=ORIENTED_EDGE ( 'NONE', *, *, #43814, .F. ) ;
#150755=CIRCLE ( 'NONE', #79991, 0.5000000000000004441 ) ;
#150766=CARTESIAN_POINT ( 'NONE',  ( 23.14999999999999503, 11.75000000000000711, 11.75000000000000000 ) ) ;
#150767=CARTESIAN_POINT ( 'NONE',  ( -2.995603634470884209E-16, 6.649999999999999467, -21.15000000000000213 ) ) ;
#150807=ORIENTED_EDGE ( 'NONE', *, *, #7527, .T. ) ;
#150820=DIRECTION ( 'NONE',  ( 0.000000000000000000, -0.4791956752371546169, -0.8777080977375152360 ) ) ;
#150827=VECTOR ( 'NONE', #135142, 1000.000000000000000 ) ;
#150829=AXIS2_PLACEMENT_3D ( 'NONE', #123898, #166901, #5189 ) ;
#150868=CARTESIAN_POINT ( 'NONE',  ( -21.05000000000000071, 6.400000000000003020, -9.930424630061573055 ) ) ;
#150888=ORIENTED_EDGE ( 'NONE', *, *, #11219, .T. ) ;
#150931=DIRECTION ( 'NONE',  ( 0.000000000000000000, 0.000000000000000000, 1.000000000000000000 ) ) ;
#150973=EDGE_LOOP ( 'NONE', ( #43136, #190140, #208817, #123494 ) ) ;
#150980=CARTESIAN_POINT ( 'NONE',  ( 21.56666275994539816, 0.000000000000000000, 6.957368406893324142 ) ) ;
#150986=ORIENTED_EDGE ( 'NONE', *, *, #104678, .F. ) ;
#150988=EDGE_CURVE ( 'NONE', #167418, #71227, #40971, .T. ) ;
#151000=DIRECTION ( 'NONE',  ( 0.000000000000000000, 0.9999631594459055250, 0.008583690987127922528 ) ) ;
#151047=CIRCLE ( 'NONE', #171926, 0.1000000000000000472 ) ;
#151058=CARTESIAN_POINT ( 'NONE',  ( -18.52309608778514161, -9.642476320055317629, -40.21459634116948223 ) ) ;
#151085=AXIS2_PLACEMENT_3D ( 'NONE', #242214, #103970, #101376 ) ;
#151119=CARTESIAN_POINT ( 'NONE',  ( 18.52326479938720993, -9.642364444915429544, -40.21475741340573506 ) ) ;
#151126=EDGE_CURVE ( 'NONE', #15628, #140135, #148790, .T. ) ;
#151137=ORIENTED_EDGE ( 'NONE', *, *, #53381, .T. ) ;
#151138=DIRECTION ( 'NONE',  ( -0.7071067811865389130, 8.659560562355038861E-17, -0.7071067811865561215 ) ) ;
#151150=CARTESIAN_POINT ( 'NONE',  ( -23.15000000000000213, 11.75000000000000000, 0.000000000000000000 ) ) ;
#151154=FACE_OUTER_BOUND ( 'NONE', #84088, .T. ) ;
#151178=ORIENTED_EDGE ( 'NONE', *, *, #240523, .T. ) ;
#151205=ORIENTED_EDGE ( 'NONE', *, *, #3741, .T. ) ;
#151214=CIRCLE ( 'NONE', #184498, 4.149999999999999467 ) ;
#151246=EDGE_CURVE ( 'NONE', #163009, #111888, #190990, .T. ) ;
#151247=DIRECTION ( 'NONE',  ( 0.000000000000000000, 0.000000000000000000, 1.000000000000000000 ) ) ;
#151306=ORIENTED_EDGE ( 'NONE', *, *, #240865, .T. ) ;
#151309=AXIS2_PLACEMENT_3D ( 'NONE', #249885, #9990, #126066 ) ;
#151323=EDGE_CURVE ( 'NONE', #214033, #193752, #176074, .T. ) ;
#151334=EDGE_CURVE ( 'NONE', #156131, #108803, #20289, .T. ) ;
#151353=ORIENTED_EDGE ( 'NONE', *, *, #160197, .F. ) ;
#151368=ADVANCED_FACE ( 'NONE', ( #160365 ), #18167, .F. ) ;
#151383=CARTESIAN_POINT ( 'NONE',  ( -21.45000000000000284, 7.708578643762696636, -21.25000000000000000 ) ) ;
#151413=ORIENTED_EDGE ( 'NONE', *, *, #240919, .T. ) ;
#151414=DIRECTION ( 'NONE',  ( 0.7071067811865487940, 8.659560562354918067E-17, 0.7071067811865463515 ) ) ;
#151450=VECTOR ( 'NONE', #7728, 1000.000000000000000 ) ;
#151477=AXIS2_PLACEMENT_3D ( 'NONE', #92487, #172071, #14265 ) ;
#151497=LINE ( 'NONE', #70680, #89606 ) ;
#151510=ORIENTED_EDGE ( 'NONE', *, *, #178072, .T. ) ;
#151551=ORIENTED_EDGE ( 'NONE', *, *, #158963, .T. ) ;
#151561=EDGE_CURVE ( 'NONE', #192659, #214669, #128613, .T. ) ;
#151579=CARTESIAN_POINT ( 'NONE',  ( 23.14999999999999503, 11.65000000000000746, 11.75000000000000000 ) ) ;
#151627=DIRECTION ( 'NONE',  ( -1.000000000000000000, -2.952720810173289112E-16, 0.000000000000000000 ) ) ;
#151680=EDGE_CURVE ( 'NONE', #19733, #99784, #41065, .T. ) ;
#151686=CARTESIAN_POINT ( 'NONE',  ( -21.55000000000000071, 7.349999999999998757, -12.25000000000000000 ) ) ;
#151695=DIRECTION ( 'NONE',  ( 1.000000000000000000, -0.000000000000000000, 0.000000000000000000 ) ) ;
#151735=ORIENTED_EDGE ( 'NONE', *, *, #151762, .T. ) ;
#151743=DIRECTION ( 'NONE',  ( 1.000000000000000000, 7.304098846218134667E-16, -0.000000000000000000 ) ) ;
#151762=EDGE_CURVE ( 'NONE', #239696, #113692, #239910, .T. ) ;
#151784=ORIENTED_EDGE ( 'NONE', *, *, #106095, .F. ) ;
#151788=DIRECTION ( 'NONE',  ( 0.000000000000000000, 0.000000000000000000, 1.000000000000000000 ) ) ;
#151817=FACE_OUTER_BOUND ( 'NONE', #255879, .T. ) ;
#151861=ORIENTED_EDGE ( 'NONE', *, *, #143549, .T. ) ;
#151884=CARTESIAN_POINT ( 'NONE',  ( -21.14999999999999858, 0.09779029130879170195, 6.257814610476114758 ) ) ;
#151895=SURFACE_SIDE_STYLE ('',( #253522 ) ) ;
#151899=ORIENTED_EDGE ( 'NONE', *, *, #169503, .T. ) ;
#151900=ORIENTED_EDGE ( 'NONE', *, *, #74938, .T. ) ;
#151906=DIRECTION ( 'NONE',  ( 0.000000000000000000, -0.9908441862701600211, -0.1350103645451876666 ) ) ;
#151914=DIRECTION ( 'NONE',  ( 0.000000000000000000, -1.224646799147321160E-16, 1.000000000000000000 ) ) ;
#151921=CIRCLE ( 'NONE', #152102, 0.1000000000000002554 ) ;
#151922=DIRECTION ( 'NONE',  ( 0.000000000000000000, 1.000000000000000000, 0.000000000000000000 ) ) ;
#151924=AXIS2_PLACEMENT_3D ( 'NONE', #221936, #26342, #122878 ) ;
#151938=VERTEX_POINT ( 'NONE', #201090 ) ;
#151984=CARTESIAN_POINT ( 'NONE',  ( 18.49999999999999289, 6.450000000000001066, -21.15000000000000213 ) ) ;
#152000=ORIENTED_EDGE ( 'NONE', *, *, #131163, .T. ) ;
#152032=AXIS2_PLACEMENT_3D ( 'NONE', #248338, #30598, #69719 ) ;
#152033=CARTESIAN_POINT ( 'NONE',  ( -22.48660254037843487, 11.65000000000000036, 0.04999999999998061551 ) ) ;
#152066=CARTESIAN_POINT ( 'NONE',  ( 20.94999999999999574, -11.41227409414968719, -2.900000000000003464 ) ) ;
#152102=AXIS2_PLACEMENT_3D ( 'NONE', #167868, #11334, #145691 ) ;
#152108=CIRCLE ( 'NONE', #18797, 0.09999999999999939493 ) ;
#152147=CARTESIAN_POINT ( 'NONE',  ( -21.07928932188134041, 0.09889514565439468108, 6.328516656393293083 ) ) ;
#152160=ORIENTED_EDGE ( 'NONE', *, *, #138834, .F. ) ;
#152164=CARTESIAN_POINT ( 'NONE',  ( 20.95512820512820440, 10.62384868371188062, -21.25000000000000000 ) ) ;
#152180=LINE ( 'NONE', #8793, #41290 ) ;
#152186=DIRECTION ( 'NONE',  ( -1.000000000000000000, -0.000000000000000000, -0.000000000000000000 ) ) ;
#152193=ORIENTED_EDGE ( 'NONE', *, *, #230123, .T. ) ;
#152282=DIRECTION ( 'NONE',  ( 0.000000000000000000, 0.3738317757009225195, 0.9274965247785541544 ) ) ;
#152294=FACE_OUTER_BOUND ( 'NONE', #25528, .T. ) ;
#152299=VECTOR ( 'NONE', #126293, 1000.000000000000000 ) ;
#152314=ORIENTED_EDGE ( 'NONE', *, *, #97773, .F. ) ;
#152345=ORIENTED_EDGE ( 'NONE', *, *, #119400, .T. ) ;
#152347=AXIS2_PLACEMENT_3D ( 'NONE', #162940, #217736, #121268 ) ;
#152349=DIRECTION ( 'NONE',  ( 0.000000000000000000, 0.000000000000000000, 1.000000000000000000 ) ) ;
#152360=DIRECTION ( 'NONE',  ( -0.000000000000000000, 0.1350103645451876666, -0.9908441862701600211 ) ) ;
#152362=CARTESIAN_POINT ( 'NONE',  ( -18.46919391072058758, -9.670724388277745831, -40.17380353179954255 ) ) ;
#152388=CARTESIAN_POINT ( 'NONE',  ( 20.94999999999999574, 0.000000000000000000, 0.000000000000000000 ) ) ;
#152425=CARTESIAN_POINT ( 'NONE',  ( 18.33683296300432986, -9.511149971132869752, -40.40570741271005062 ) ) ;
#152436=DIRECTION ( 'NONE',  ( 0.000000000000000000, 0.000000000000000000, -1.000000000000000000 ) ) ;
#152509=CARTESIAN_POINT ( 'NONE',  ( -18.59999999999999787, 0.000000000000000000, -33.50000000000000000 ) ) ;
#152538=DIRECTION ( 'NONE',  ( 0.000000000000000000, 0.1568667991644863147, 0.9876197685951252359 ) ) ;
#152566=CARTESIAN_POINT ( 'NONE',  ( 20.94999999999999929, 5.850000000000001421, -23.36750277572207679 ) ) ;
#152577=ORIENTED_EDGE ( 'NONE', *, *, #199555, .F. ) ;
#152588=ORIENTED_EDGE ( 'NONE', *, *, #72815, .F. ) ;
#152590=CIRCLE ( 'NONE', #19267, 0.1999999999999987899 ) ;
#152611=CARTESIAN_POINT ( 'NONE',  ( 23.14999999999998437, -11.75000000000000000, 3.469446951953614189E-15 ) ) ;
#152658=CYLINDRICAL_SURFACE ( 'NONE', #182063, 0.5000000000000004441 ) ;
#152671=DIRECTION ( 'NONE',  ( 0.000000000000000000, -1.000000000000000000, 0.000000000000000000 ) ) ;
#152673=CARTESIAN_POINT ( 'NONE',  ( -18.59999999999999787, 9.250000000000001776, -12.34999999999999964 ) ) ;
#152730=CARTESIAN_POINT ( 'NONE',  ( 21.14999999999999858, 6.540656951701244282, 0.000000000000000000 ) ) ;
#152733=ORIENTED_EDGE ( 'NONE', *, *, #15585, .F. ) ;
#152741=DIRECTION ( 'NONE',  ( 1.000000000000000000, 0.000000000000000000, 0.000000000000000000 ) ) ;
#152748=DIRECTION ( 'NONE',  ( -6.938893903907224433E-15, 1.000000000000000000, 0.000000000000000000 ) ) ;
#152767=CYLINDRICAL_SURFACE ( 'NONE', #88315, 0.1000000000000000472 ) ;
#152788=CIRCLE ( 'NONE', #240260, 0.09999999999999939493 ) ;
#152794=ORIENTED_EDGE ( 'NONE', *, *, #222483, .F. ) ;
#152808=ORIENTED_EDGE ( 'NONE', *, *, #36215, .T. ) ;
#152837=ORIENTED_EDGE ( 'NONE', *, *, #39739, .F. ) ;
#152840=VERTEX_POINT ( 'NONE', #63511 ) ;
#152850=ADVANCED_FACE ( 'NONE', ( #244713 ), #24429, .T. ) ;
#152875=CYLINDRICAL_SURFACE ( 'NONE', #88891, 0.1000000000000028644 ) ;
#152893=DIRECTION ( 'NONE',  ( -1.000000000000000000, 0.000000000000000000, 0.000000000000000000 ) ) ;
#152896=CIRCLE ( 'NONE', #23894, 0.09999999999999939493 ) ;
#152930=CIRCLE ( 'NONE', #86231, 0.09999999999999939493 ) ;
#152937=CARTESIAN_POINT ( 'NONE',  ( 20.94999999999999574, 0.000000000000000000, 0.000000000000000000 ) ) ;
#152965=DIRECTION ( 'NONE',  ( 1.000000000000000000, -0.000000000000000000, -0.000000000000000000 ) ) ;
#152969=ADVANCED_FACE ( 'NONE', ( #165196 ), #166796, .F. ) ;
#153055=DIRECTION ( 'NONE',  ( 0.000000000000000000, -1.000000000000000000, 0.000000000000000000 ) ) ;
#153059=ORIENTED_EDGE ( 'NONE', *, *, #232248, .F. ) ;
#153076=ORIENTED_EDGE ( 'NONE', *, *, #35424, .F. ) ;
#153085=FACE_OUTER_BOUND ( 'NONE', #87338, .T. ) ;
#153115=VERTEX_POINT ( 'NONE', #154648 ) ;
#153119=ORIENTED_EDGE ( 'NONE', *, *, #141896, .T. ) ;
#153156=EDGE_CURVE ( 'NONE', #197965, #11636, #116866, .T. ) ;
#153163=CIRCLE ( 'NONE', #240598, 0.5000000000000004441 ) ;
#153187=ORIENTED_EDGE ( 'NONE', *, *, #39113, .T. ) ;
#153203=ORIENTED_EDGE ( 'NONE', *, *, #104562, .F. ) ;
#153214=CARTESIAN_POINT ( 'NONE',  ( 20.85000000000000142, -1.835859311443637010, -45.00443916879852679 ) ) ;
#153240=DIRECTION ( 'NONE',  ( 1.000000000000000000, 0.000000000000000000, -0.000000000000000000 ) ) ;
#153261=DIRECTION ( 'NONE',  ( 1.000000000000000000, -0.000000000000000000, -0.000000000000000000 ) ) ;
#153265=ORIENTED_EDGE ( 'NONE', *, *, #130343, .F. ) ;
#153274=CYLINDRICAL_SURFACE ( 'NONE', #200279, 0.1000000000000028644 ) ;
#153276=LINE ( 'NONE', #11162, #166550 ) ;
#153308=ORIENTED_EDGE ( 'NONE', *, *, #169002, .F. ) ;
#153325=ADVANCED_FACE ( 'NONE', ( #80178 ), #216988, .T. ) ;
#153335=EDGE_CURVE ( 'NONE', #24291, #197777, #33716, .T. ) ;
#153372=EDGE_CURVE ( 'NONE', #44201, #71370, #52302, .T. ) ;
#153373=FACE_OUTER_BOUND ( 'NONE', #37495, .T. ) ;
#153381=CARTESIAN_POINT ( 'NONE',  ( 20.94999999999999929, 5.499999999999998224, -21.09473398108690390 ) ) ;
#153455=CIRCLE ( 'NONE', #24243, 4.099999999999999645 ) ;
#153466=EDGE_CURVE ( 'NONE', #242536, #17057, #251806, .T. ) ;
#153511=TOROIDAL_SURFACE ( 'NONE', #245040, 11.70000000000000639, 0.1000000000000000056 ) ;
#153512=ORIENTED_EDGE ( 'NONE', *, *, #251385, .F. ) ;
#153513=CARTESIAN_POINT ( 'NONE',  ( 0.000000000000000000, 0.000000000000000000, 0.000000000000000000 ) ) ;
#153517=ORIENTED_EDGE ( 'NONE', *, *, #106129, .F. ) ;
#153518=ORIENTED_EDGE ( 'NONE', *, *, #73530, .F. ) ;
#153538=CIRCLE ( 'NONE', #253426, 11.75000000000000000 ) ;
#153576=ORIENTED_EDGE ( 'NONE', *, *, #240373, .T. ) ;
#153600=CARTESIAN_POINT ( 'NONE',  ( 20.94999999999999929, 10.29270135740183179, -38.95736188715193293 ) ) ;
#153601=EDGE_LOOP ( 'NONE', ( #218454, #60077, #197113, #94145 ) ) ;
#153619=CIRCLE ( 'NONE', #45414, 0.09999999999999993616 ) ;
#153713=ORIENTED_EDGE ( 'NONE', *, *, #124593, .F. ) ;
#153720=CARTESIAN_POINT ( 'NONE',  ( 18.59999999999999787, -9.321008403361304318, -7.235938249077860540 ) ) ;
#153735=CARTESIAN_POINT ( 'NONE',  ( 18.50000000000000355, -9.421074344987191651, -40.32447205943020663 ) ) ;
#153736=CIRCLE ( 'NONE', #162068, 0.1000000000000000472 ) ;
#153754=ORIENTED_EDGE ( 'NONE', *, *, #223064, .F. ) ;
#153804=ADVANCED_FACE ( 'NONE', ( #172013 ), #72902, .T. ) ;
#153820=CIRCLE ( 'NONE', #257759, 11.70000000000000639 ) ;
#153831=CARTESIAN_POINT ( 'NONE',  ( 21.05000000000000071, 8.776282895292474961, -8.488000721584361585 ) ) ;
#153845=ORIENTED_EDGE ( 'NONE', *, *, #52722, .T. ) ;
#153854=FACE_OUTER_BOUND ( 'NONE', #236660, .T. ) ;
#153910=CARTESIAN_POINT ( 'NONE',  ( -21.05000000000000071, 11.65000000000000036, -0.1000000000000028644 ) ) ;
#153911=CARTESIAN_POINT ( 'NONE',  ( -22.43310005002225438, 0.005636942140875567109, 11.64966212713439830 ) ) ;
#153947=CARTESIAN_POINT ( 'NONE',  ( -22.50000000000000000, 0.000000000000000000, 0.000000000000000000 ) ) ;
#153948=DIRECTION ( 'NONE',  ( 1.000000000000000000, 0.000000000000000000, 0.000000000000000000 ) ) ;
#153950=DIRECTION ( 'NONE',  ( -1.000000000000000000, 0.000000000000000000, 0.000000000000000000 ) ) ;
#153971=VERTEX_POINT ( 'NONE', #234498 ) ;
#154027=DIRECTION ( 'NONE',  ( 0.000000000000000000, 0.000000000000000000, -1.000000000000000000 ) ) ;
#154061=CARTESIAN_POINT ( 'NONE',  ( -21.09610168723072832, 6.378955715224779333, 0.03358950689149174662 ) ) ;
#154062=DIRECTION ( 'NONE',  ( 1.000000000000000000, 3.265361837132813093E-16, -0.000000000000000000 ) ) ;
#154071=AXIS2_PLACEMENT_3D ( 'NONE', #201749, #206893, #145616 ) ;
#154076=ORIENTED_EDGE ( 'NONE', *, *, #218792, .F. ) ;
#154080=DIRECTION ( 'NONE',  ( 0.000000000000000000, -1.000000000000000000, -1.897661533703519897E-16 ) ) ;
#154098=APPLICATION_CONTEXT ( 'automotive_design' ) ;
#154116=DIRECTION ( 'NONE',  ( 0.000000000000000000, 0.000000000000000000, 1.000000000000000000 ) ) ;
#154127=DIRECTION ( 'NONE',  ( 0.000000000000000000, 0.000000000000000000, -1.000000000000000000 ) ) ;
#154128=ORIENTED_EDGE ( 'NONE', *, *, #196554, .F. ) ;
#154135=AXIS2_PLACEMENT_3D ( 'NONE', #235934, #95149, #217637 ) ;
#154161=CYLINDRICAL_SURFACE ( 'NONE', #15008, 0.09999999999999939493 ) ;
#154166=DIRECTION ( 'NONE',  ( 0.000000000000000000, 0.000000000000000000, -1.000000000000000000 ) ) ;
#154192=ORIENTED_EDGE ( 'NONE', *, *, #14460, .F. ) ;
#154215=CARTESIAN_POINT ( 'NONE',  ( -22.48660254037843487, 11.65000000000000036, 0.04999999999998061551 ) ) ;
#154247=ORIENTED_EDGE ( 'NONE', *, *, #157854, .T. ) ;
#154267=CARTESIAN_POINT ( 'NONE',  ( 18.50000000000000000, -9.499999999999998224, -7.032069396699667685 ) ) ;
#154281=CARTESIAN_POINT ( 'NONE',  ( 22.59066674512251183, 11.75000000000000000, 0.03050412363060323040 ) ) ;
#154299=CARTESIAN_POINT ( 'NONE',  ( -20.94999999999999929, 1.360870587192041681, -8.072997927090961312 ) ) ;
#154329=ORIENTED_EDGE ( 'NONE', *, *, #21758, .T. ) ;
#154333=ORIENTED_EDGE ( 'NONE', *, *, #178167, .F. ) ;
#154338=EDGE_CURVE ( 'NONE', #219800, #137417, #84040, .T. ) ;
#154351=CIRCLE ( 'NONE', #41897, 12.87500000000000000 ) ;
#154352=FACE_OUTER_BOUND ( 'NONE', #17644, .T. ) ;
#154375=CYLINDRICAL_SURFACE ( 'NONE', #64054, 0.09999999999999811817 ) ;
#154386=AXIS2_PLACEMENT_3D ( 'NONE', #187530, #145797, #8871 ) ;
#154387=ORIENTED_EDGE ( 'NONE', *, *, #37072, .T. ) ;
#154433=DIRECTION ( 'NONE',  ( 0.000000000000000000, 0.000000000000000000, -1.000000000000000000 ) ) ;
#154471=ORIENTED_EDGE ( 'NONE', *, *, #119533, .F. ) ;
#154509=DIRECTION ( 'NONE',  ( 0.000000000000000000, 6.938893903907270030E-14, 1.000000000000000000 ) ) ;
#154513=EDGE_CURVE ( 'NONE', #252270, #156138, #205060, .T. ) ;
#154523=AXIS2_PLACEMENT_3D ( 'NONE', #15012, #117931, #98331 ) ;
#154552=ORIENTED_EDGE ( 'NONE', *, *, #59474, .F. ) ;
#154580=FACE_OUTER_BOUND ( 'NONE', #139501, .T. ) ;
#154625=DIRECTION ( 'NONE',  ( 0.000000000000000000, 0.000000000000000000, -1.000000000000000000 ) ) ;
#154633=EDGE_LOOP ( 'NONE', ( #122320, #80337, #91667, #198297 ) ) ;
#154648=CARTESIAN_POINT ( 'NONE',  ( -23.15000000000000213, -11.75000000000000000, -30.39999999999999503 ) ) ;
#154657=DIRECTION ( 'NONE',  ( 1.000000000000000000, -0.000000000000000000, -0.000000000000000000 ) ) ;
#154668=CARTESIAN_POINT ( 'NONE',  ( 21.05000000000000071, 11.65000000000000746, 0.000000000000000000 ) ) ;
#154685=DIRECTION ( 'NONE',  ( 3.616040088954497272E-32, -1.224646799147352961E-16, 1.000000000000000000 ) ) ;
#154692=CARTESIAN_POINT ( 'NONE',  ( 20.12500000000000000, 9.749999999999998224, -21.15000000000000213 ) ) ;
#154699=CIRCLE ( 'NONE', #88176, 0.09999999999999939493 ) ;
#154718=CARTESIAN_POINT ( 'NONE',  ( -20.64999999999999858, 2.499999999999998668, -20.27537807723789953 ) ) ;
#154726=ORIENTED_EDGE ( 'NONE', *, *, #41117, .T. ) ;
#154731=EDGE_CURVE ( 'NONE', #94704, #143019, #233646, .T. ) ;
#154764=EDGE_CURVE ( 'NONE', #103887, #52039, #137858, .T. ) ;
#154771=EDGE_CURVE ( 'NONE', #16494, #255303, #57940, .T. ) ;
#154772=ORIENTED_EDGE ( 'NONE', *, *, #30824, .F. ) ;
#154776=ADVANCED_FACE ( 'NONE', ( #136178 ), #187967, .T. ) ;
#154809=CARTESIAN_POINT ( 'NONE',  ( -21.14999999999999858, -11.75000000000000000, 3.469446951953614189E-15 ) ) ;
#154820=ORIENTED_EDGE ( 'NONE', *, *, #54179, .F. ) ;
#154870=CARTESIAN_POINT ( 'NONE',  ( 21.09793522318410552, 10.72462451021277730, -12.23929087097709356 ) ) ;
#154876=CARTESIAN_POINT ( 'NONE',  ( 18.59999999999999076, 6.649999999999999467, -21.15000000000000213 ) ) ;
#154916=DIRECTION ( 'NONE',  ( 1.000000000000000000, -7.304098846218134667E-16, -0.000000000000000000 ) ) ;
#154927=ADVANCED_FACE ( 'NONE', ( #26558 ), #186481, .T. ) ;
#154957=VECTOR ( 'NONE', #132607, 1000.000000000000000 ) ;
#154964=CYLINDRICAL_SURFACE ( 'NONE', #43648, 0.1000000000000008105 ) ;
#154965=VERTEX_POINT ( 'NONE', #169952 ) ;
#154986=CARTESIAN_POINT ( 'NONE',  ( 18.48413544395645047, -9.664304033627754364, -40.18310499303830596 ) ) ;
#155025=AXIS2_PLACEMENT_3D ( 'NONE', #117353, #258091, #216439 ) ;
#155050=AXIS2_PLACEMENT_3D ( 'NONE', #238037, #135073, #257546 ) ;
#155060=CARTESIAN_POINT ( 'NONE',  ( -21.08884785362073089, 0.04978309506672475016, 6.357193367425618469 ) ) ;
#155071=TOROIDAL_SURFACE ( 'NONE', #225755, 0.2000000000000000111, 0.1000000000000000056 ) ;
#155076=ADVANCED_FACE ( 'NONE', ( #77208 ), #208810, .F. ) ;
#155088=CARTESIAN_POINT ( 'NONE',  ( -20.54999999999999716, 2.500000000000000444, -13.22462192276210224 ) ) ;
#155096=ORIENTED_EDGE ( 'NONE', *, *, #41161, .F. ) ;
#155121=DIRECTION ( 'NONE',  ( 1.000000000000000000, -0.000000000000000000, -0.000000000000000000 ) ) ;
#155147=CARTESIAN_POINT ( 'NONE',  ( -23.25000000000000000, -8.596261682242989366, -24.04987248284972168 ) ) ;
#155165=ORIENTED_EDGE ( 'NONE', *, *, #53357, .F. ) ;
#155175=AXIS2_PLACEMENT_3D ( 'NONE', #210650, #8604, #32041 ) ;
#155214=DIRECTION ( 'NONE',  ( 0.000000000000000000, 0.000000000000000000, -1.000000000000000000 ) ) ;
#155228=EDGE_CURVE ( 'NONE', #112457, #168131, #213069, .T. ) ;
#155234=CARTESIAN_POINT ( 'NONE',  ( -18.59999999999999787, 11.64999999999999680, -12.14999999999999858 ) ) ;
#155238=FACE_OUTER_BOUND ( 'NONE', #181627, .T. ) ;
#155250=CARTESIAN_POINT ( 'NONE',  ( 21.30000000000002558, 0.000000000000000000, 4.049999999999998934 ) ) ;
#155261=DIRECTION ( 'NONE',  ( 0.000000000000000000, 0.000000000000000000, 1.000000000000000000 ) ) ;
#155282=DIRECTION ( 'NONE',  ( -4.801466763864313332E-15, -0.2605042016806672911, -0.9654727137038716656 ) ) ;
#155332=EDGE_LOOP ( 'NONE', ( #151137, #39945, #245688, #101047 ) ) ;
#155336=CARTESIAN_POINT ( 'NONE',  ( 20.95539060131842746, 10.62386215765564579, -7.653733813656191209 ) ) ;
#155347=ORIENTED_EDGE ( 'NONE', *, *, #30394, .F. ) ;
#155349=VECTOR ( 'NONE', #190059, 1000.000000000000000 ) ;
#155371=DIRECTION ( 'NONE',  ( -0.000000000000000000, -1.000000000000000000, 6.308085367188393199E-16 ) ) ;
#155443=DIRECTION ( 'NONE',  ( -1.000000000000000000, -0.000000000000000000, -0.000000000000000000 ) ) ;
#155514=CARTESIAN_POINT ( 'NONE',  ( -21.05000000000000071, -0.09999999999999939493, 11.65000000000000036 ) ) ;
#155532=AXIS2_PLACEMENT_3D ( 'NONE', #157927, #100437, #18366 ) ;
#155535=DIRECTION ( 'NONE',  ( -0.000000000000000000, -0.000000000000000000, -1.000000000000000000 ) ) ;
#155568=CARTESIAN_POINT ( 'NONE',  ( -18.41418431465368144, -9.500000000000223821, -40.10018939122146264 ) ) ;
#155592=DIRECTION ( 'NONE',  ( -1.000000000000000000, 0.000000000000000000, 0.000000000000000000 ) ) ;
#155607=ADVANCED_FACE ( 'NONE', ( #239854 ), #847, .F. ) ;
#155648=CARTESIAN_POINT ( 'NONE',  ( -18.39999999999999858, -9.682403433476396870, -40.15684337741279109 ) ) ;
#155674=DIRECTION ( 'NONE',  ( 0.000000000000000000, -0.000000000000000000, 1.000000000000000000 ) ) ;
#155691=DIRECTION ( 'NONE',  ( -0.000000000000000000, 1.000000000000000000, 0.000000000000000000 ) ) ;
#155692=CARTESIAN_POINT ( 'NONE',  ( 18.59999999999999076, 11.75000000000000355, -24.85000000000000142 ) ) ;
#155718=DIRECTION ( 'NONE',  ( 0.000000000000000000, 0.000000000000000000, -1.000000000000000000 ) ) ;
#155728=EDGE_CURVE ( 'NONE', #224530, #56955, #127603, .T. ) ;
#155733=CARTESIAN_POINT ( 'NONE',  ( -21.06715728752538297, 11.74999999999999467, -7.014805770654001904 ) ) ;
#155737=DIRECTION ( 'NONE',  ( 4.408576920032447355E-17, -0.1350103645451876666, 0.9908441862701600211 ) ) ;
#155796=AXIS2_PLACEMENT_3D ( 'NONE', #208200, #247295, #126058 ) ;
#155798=VERTEX_POINT ( 'NONE', #252662 ) ;
#155812=CYLINDRICAL_SURFACE ( 'NONE', #187436, 0.09999999999999939493 ) ;
#155819=AXIS2_PLACEMENT_3D ( 'NONE', #36628, #156578, #237365 ) ;
#155824=ORIENTED_EDGE ( 'NONE', *, *, #214699, .F. ) ;
#155861=TOROIDAL_SURFACE ( 'NONE', #243301, 0.4000000000000012990, 0.1000000000000000056 ) ;
#155874=TOROIDAL_SURFACE ( 'NONE', #47684, 12.97499999999999609, 0.1000000000000000056 ) ;
#155881=CIRCLE ( 'NONE', #68566, 0.1000000000000016986 ) ;
#155950=AXIS2_PLACEMENT_3D ( 'NONE', #41026, #137511, #235336 ) ;
#155953=ORIENTED_EDGE ( 'NONE', *, *, #30268, .T. ) ;
#155962=CARTESIAN_POINT ( 'NONE',  ( -18.50000000000000000, -1.835341550224411922, -11.55515129256297868 ) ) ;
#155997=DIRECTION ( 'NONE',  ( -1.000000000000000000, 0.000000000000000000, 0.000000000000000000 ) ) ;
#156020=CIRCLE ( 'NONE', #181148, 2.000000000000002665 ) ;
#156027=DIRECTION ( 'NONE',  ( 1.875376730785737719E-16, -1.000000000000000000, 0.000000000000000000 ) ) ;
#156051=CARTESIAN_POINT ( 'NONE',  ( 20.94999999999999574, 8.926614585087095932, -8.471683019223121391 ) ) ;
#156060=ADVANCED_FACE ( 'NONE', ( #67307 ), #3477, .F. ) ;
#156100=ORIENTED_EDGE ( 'NONE', *, *, #95501, .F. ) ;
#156121=EDGE_LOOP ( 'NONE', ( #76521, #223302, #24412 ) ) ;
#156130=DIRECTION ( 'NONE',  ( 1.000000000000000000, 0.000000000000000000, 0.000000000000000000 ) ) ;
#156131=VERTEX_POINT ( 'NONE', #64740 ) ;
#156138=VERTEX_POINT ( 'NONE', #63451 ) ;
#156140=SPHERICAL_SURFACE ( 'NONE', #236158, 0.1000000000000000056 ) ;
#156152=ORIENTED_EDGE ( 'NONE', *, *, #41161, .T. ) ;
#156197=DIRECTION ( 'NONE',  ( -1.000000000000000000, -3.265361837132813093E-16, 0.000000000000000000 ) ) ;
#156202=EDGE_CURVE ( 'NONE', #249634, #116906, #105068, .T. ) ;
#156221=VERTEX_POINT ( 'NONE', #88124 ) ;
#156233=CARTESIAN_POINT ( 'NONE',  ( 21.05000000000000071, -0.02138556593762391128, 6.304961112684640767 ) ) ;
#156241=CARTESIAN_POINT ( 'NONE',  ( 18.50000000000000000, -10.35479209692539548, -27.25654098307376216 ) ) ;
#156283=EDGE_CURVE ( 'NONE', #16503, #214669, #69907, .T. ) ;
#156321=ORIENTED_EDGE ( 'NONE', *, *, #237608, .T. ) ;
#156328=DIRECTION ( 'NONE',  ( 0.000000000000000000, 0.000000000000000000, 1.000000000000000000 ) ) ;
#156332=CARTESIAN_POINT ( 'NONE',  ( -21.05000000000000071, 4.898587196589414801E-16, -37.50000000000000000 ) ) ;
#156333=EDGE_CURVE ( 'NONE', #16525, #38380, #114322, .T. ) ;
#156352=CIRCLE ( 'NONE', #2178, 0.2000000000000005107 ) ;
#156383=CARTESIAN_POINT ( 'NONE',  ( 18.59999999999999432, 5.699452464321598910, 12.54227395656983290 ) ) ;
#156397=AXIS2_PLACEMENT_3D ( 'NONE', #164963, #90550, #65858 ) ;
#156402=AXIS2_PLACEMENT_3D ( 'NONE', #56356, #65040, #198453 ) ;
#156433=AXIS2_PLACEMENT_3D ( 'NONE', #146246, #244065, #184097 ) ;
#156435=CARTESIAN_POINT ( 'NONE',  ( 20.30466543256828160, 9.304236939255389416, -8.253662651392039251 ) ) ;
#156464=CARTESIAN_POINT ( 'NONE',  ( -22.50000000000000000, 0.09999999999999939493, 11.64957080754479968 ) ) ;
#156516=FACE_OUTER_BOUND ( 'NONE', #257960, .T. ) ;
#156522=CARTESIAN_POINT ( 'NONE',  ( -18.50000000000000000, -1.736257131597395809, -11.56865232901749785 ) ) ;
#156531=CARTESIAN_POINT ( 'NONE',  ( 18.59999999999999076, 10.49142135623730709, -24.75000000000000000 ) ) ;
#156565=DIRECTION ( 'NONE',  ( 0.000000000000000000, 0.000000000000000000, -1.000000000000000000 ) ) ;
#156578=DIRECTION ( 'NONE',  ( 0.000000000000000000, 0.1298341882520022972, 0.9915357197604853789 ) ) ;
#156601=ADVANCED_FACE ( 'NONE', ( #114805 ), #92664, .T. ) ;
#156616=CIRCLE ( 'NONE', #235664, 0.09999999999999939493 ) ;
#156648=EDGE_LOOP ( 'NONE', ( #59157, #219691, #10777, #228826 ) ) ;
#156671=VERTEX_POINT ( 'NONE', #113519 ) ;
#156680=EDGE_LOOP ( 'NONE', ( #85665, #2373, #185892 ) ) ;
#156683=ADVANCED_FACE ( 'NONE', ( #53547 ), #147847, .T. ) ;
#156685=ORIENTED_EDGE ( 'NONE', *, *, #131242, .T. ) ;
#156717=CARTESIAN_POINT ( 'NONE',  ( -20.94999999999999929, 5.849999999999949019, -10.13249722427797117 ) ) ;
#156737=DIRECTION ( 'NONE',  ( 0.000000000000000000, 0.000000000000000000, -1.000000000000000000 ) ) ;
#156746=CARTESIAN_POINT ( 'NONE',  ( 20.85000000000000142, -1.835859311443637010, -45.00443916879852679 ) ) ;
#156752=DIRECTION ( 'NONE',  ( 0.000000000000000000, 0.000000000000000000, -1.000000000000000000 ) ) ;
#156756=CYLINDRICAL_SURFACE ( 'NONE', #22632, 0.09999999999999939493 ) ;
#156800=PLANE ( 'NONE',  #212576 ) ;
#156830=CARTESIAN_POINT ( 'NONE',  ( 22.59999999999999432, 11.74956712348939192, 0.1008583690987083364 ) ) ;
#156896=EDGE_CURVE ( 'NONE', #227165, #146767, #169378, .T. ) ;
#156981=TOROIDAL_SURFACE ( 'NONE', #44539, 0.4000000000000005773, 0.1000000000000000056 ) ;
#156983=DIRECTION ( 'NONE',  ( 1.000000000000000000, 0.000000000000000000, 0.000000000000000000 ) ) ;
#157022=DIRECTION ( 'NONE',  ( 0.000000000000000000, -0.000000000000000000, 1.000000000000000000 ) ) ;
#157029=ORIENTED_EDGE ( 'NONE', *, *, #50517, .F. ) ;
#157037=EDGE_LOOP ( 'NONE', ( #42206, #51343, #231742, #12866 ) ) ;
#157044=CARTESIAN_POINT ( 'NONE',  ( -20.54999999999999716, 9.350000000000001421, -21.15000000000000213 ) ) ;
#157066=CIRCLE ( 'NONE', #211225, 0.09999999999999939493 ) ;
#157091=DIRECTION ( 'NONE',  ( 0.000000000000000000, -1.000000000000000000, 0.000000000000000000 ) ) ;
#157136=LINE ( 'NONE', #57990, #216788 ) ;
#157137=ADVANCED_FACE ( 'NONE', ( #220003 ), #133172, .T. ) ;
#157140=FACE_OUTER_BOUND ( 'NONE', #61064, .T. ) ;
#157144=CIRCLE ( 'NONE', #190469, 4.000000000000000000 ) ;
#157159=TOROIDAL_SURFACE ( 'NONE', #7287, 12.77500000000000036, 0.1000000000000000056 ) ;
#157189=CARTESIAN_POINT ( 'NONE',  ( -23.25000000000000000, 4.959819536546777642E-16, 4.049999999999998934 ) ) ;
#157204=ADVANCED_FACE ( 'NONE', ( #184717 ), #127327, .T. ) ;
#157212=DIRECTION ( 'NONE',  ( 0.000000000000000000, -0.5907332058517320572, 0.8068669527896995541 ) ) ;
#157218=CARTESIAN_POINT ( 'NONE',  ( 18.59999999999999076, 6.450000000000001066, -21.25000000000000000 ) ) ;
#157226=VERTEX_POINT ( 'NONE', #244687 ) ;
#157233=EDGE_CURVE ( 'NONE', #225538, #185736, #68723, .T. ) ;
#157235=DIRECTION ( 'NONE',  ( 0.000000000000000000, 0.000000000000000000, -1.000000000000000000 ) ) ;
#157236=DIRECTION ( 'NONE',  ( -1.000000000000000000, -0.000000000000000000, 0.000000000000000000 ) ) ;
#157240=CONICAL_SURFACE ( 'NONE', #28065, 6.250000000000000000, 0.7853981633974431720 ) ;
#157286=FACE_OUTER_BOUND ( 'NONE', #43185, .T. ) ;
#157290=VERTEX_POINT ( 'NONE', #225116 ) ;
#157300=EDGE_LOOP ( 'NONE', ( #113712, #39716, #170462, #250551 ) ) ;
#157328=ADVANCED_BREP_SHAPE_REPRESENTATION ( '', ( #104549, #2425 ), #114299 ) ;
#157339=CARTESIAN_POINT ( 'NONE',  ( 20.95392731769792150, 8.883061479188762988, -8.522227979571306733 ) ) ;
#157346=ORIENTED_EDGE ( 'NONE', *, *, #106884, .T. ) ;
#157421=DIRECTION ( 'NONE',  ( 1.000000000000000000, -0.000000000000000000, -0.000000000000000000 ) ) ;
#157488=CARTESIAN_POINT ( 'NONE',  ( -18.59999999999999787, -1.164121893241208960, -41.41484808557160591 ) ) ;
#157502=AXIS2_PLACEMENT_3D ( 'NONE', #74819, #72228, #55174 ) ;
#157510=CARTESIAN_POINT ( 'NONE',  ( 21.05000000000000426, 6.300183336267740408, 0.05132743234154404921 ) ) ;
#157521=EDGE_CURVE ( 'NONE', #63488, #55509, #10272, .T. ) ;
#157525=CIRCLE ( 'NONE', #115790, 0.09999999999999939493 ) ;
#157532=AXIS2_PLACEMENT_3D ( 'NONE', #206952, #150820, #6165 ) ;
#157555=CARTESIAN_POINT ( 'NONE',  ( 18.58703555225010362, -9.406336740788765027, -7.124944641246808708 ) ) ;
#157565=ORIENTED_EDGE ( 'NONE', *, *, #133171, .F. ) ;
#157606=ORIENTED_EDGE ( 'NONE', *, *, #241587, .T. ) ;
#157636=CARTESIAN_POINT ( 'NONE',  ( -21.07971444708686093, 0.08782343631782563165, 6.329792081626551159 ) ) ;
#157643=AXIS2_PLACEMENT_3D ( 'NONE', #69303, #165842, #127984 ) ;
#157662=CARTESIAN_POINT ( 'NONE',  ( -23.25000000000000000, -9.600000000000004974, -9.893969122652444881 ) ) ;
#157681=AXIS2_PLACEMENT_3D ( 'NONE', #203634, #164524, #144924 ) ;
#157726=CARTESIAN_POINT ( 'NONE',  ( -21.05000000000000071, -0.09999999999999939493, 6.540656951701240729 ) ) ;
#157742=EDGE_CURVE ( 'NONE', #153971, #31072, #104848, .T. ) ;
#157772=EDGE_CURVE ( 'NONE', #22057, #245427, #156020, .T. ) ;
#157773=FACE_OUTER_BOUND ( 'NONE', #98881, .T. ) ;
#157797=PRODUCT_CONTEXT ( 'NONE', #154098, 'mechanical' ) ;
#157800=CARTESIAN_POINT ( 'NONE',  ( -23.25000000000000000, -1.164121893241208960, -41.41484808557160591 ) ) ;
#157832=ORIENTED_EDGE ( 'NONE', *, *, #214888, .F. ) ;
#157834=CARTESIAN_POINT ( 'NONE',  ( -20.07928932188135107, 9.220710678118654968, -21.15000000000000213 ) ) ;
#157854=EDGE_CURVE ( 'NONE', #72182, #72309, #29253, .T. ) ;
#157898=AXIS2_PLACEMENT_3D ( 'NONE', #256525, #76658, #113223 ) ;
#157927=CARTESIAN_POINT ( 'NONE',  ( -21.64999999999999858, 7.249999999999992895, -21.15000000000000213 ) ) ;
#157933=FACE_OUTER_BOUND ( 'NONE', #121275, .T. ) ;
#157943=ORIENTED_EDGE ( 'NONE', *, *, #135744, .T. ) ;
#157949=ORIENTED_EDGE ( 'NONE', *, *, #246065, .T. ) ;
#157957=CIRCLE ( 'NONE', #37301, 0.09999999999999993616 ) ;
#157958=ORIENTED_EDGE ( 'NONE', *, *, #158656, .F. ) ;
#157972=DIRECTION ( 'NONE',  ( 2.952720810173289112E-16, -1.000000000000000000, 0.000000000000000000 ) ) ;
#157985=VERTEX_POINT ( 'NONE', #30078 ) ;
#157995=CARTESIAN_POINT ( 'NONE',  ( -20.94999999999999929, -11.41227409414968541, -30.59999999999999432 ) ) ;
#157996=CIRCLE ( 'NONE', #45521, 0.09999999999999939493 ) ;
#158017=CYLINDRICAL_SURFACE ( 'NONE', #8034, 0.09999999999999939493 ) ;
#158018=CIRCLE ( 'NONE', #45543, 0.09999999999999939493 ) ;
#158038=ORIENTED_EDGE ( 'NONE', *, *, #98384, .T. ) ;
#158081=AXIS2_PLACEMENT_3D ( 'NONE', #222538, #123464, #13785 ) ;
#158092=VERTEX_POINT ( 'NONE', #91314 ) ;
#158093=DIRECTION ( 'NONE',  ( 0.000000000000000000, -0.9876197685951252359, -0.1568667991644863424 ) ) ;
#158095=CIRCLE ( 'NONE', #53809, 0.8750000000000007772 ) ;
#158115=DIRECTION ( 'NONE',  ( 0.000000000000000000, 1.000000000000000000, 0.000000000000000000 ) ) ;
#158119=CARTESIAN_POINT ( 'NONE',  ( 21.13461538461538325, 10.61458296202553697, -12.35000000000000320 ) ) ;
#158123=DIRECTION ( 'NONE',  ( -0.000000000000000000, -0.000000000000000000, -1.000000000000000000 ) ) ;
#158135=VERTEX_POINT ( 'NONE', #160505 ) ;
#158154=EDGE_CURVE ( 'NONE', #125216, #251836, #214429, .T. ) ;
#158172=VERTEX_POINT ( 'NONE', #234892 ) ;
#158177=ORIENTED_EDGE ( 'NONE', *, *, #110604, .T. ) ;
#158203=AXIS2_PLACEMENT_3D ( 'NONE', #123384, #163801, #106356 ) ;
#158225=CARTESIAN_POINT ( 'NONE',  ( -2.995603634470884209E-16, -11.75000000000000000, -24.75000000000000000 ) ) ;
#158250=ADVANCED_FACE ( 'NONE', ( #99193 ), #37988, .T. ) ;
#158257=ORIENTED_EDGE ( 'NONE', *, *, #46920, .T. ) ;
#158267=CARTESIAN_POINT ( 'NONE',  ( 18.59999999999999787, 0.000000000000000000, 0.000000000000000000 ) ) ;
#158275=DIRECTION ( 'NONE',  ( -4.408576920032448588E-17, 0.1350103645451876666, -0.9908441862701600211 ) ) ;
#158290=LINE ( 'NONE', #440, #110412 ) ;
#158298=CIRCLE ( 'NONE', #237376, 0.09999999999999939493 ) ;
#158303=AXIS2_PLACEMENT_3D ( 'NONE', #34336, #95558, #73465 ) ;
#158318=FACE_OUTER_BOUND ( 'NONE', #77042, .T. ) ;
#158342=CARTESIAN_POINT ( 'NONE',  ( 21.14999999999999858, 10.71339244339988461, -12.25000000000000000 ) ) ;
#158344=DIRECTION ( 'NONE',  ( -0.000000000000000000, -0.000000000000000000, -1.000000000000000000 ) ) ;
#158364=EDGE_LOOP ( 'NONE', ( #115517, #235886, #185532, #145554 ) ) ;
#158367=DIRECTION ( 'NONE',  ( 0.000000000000000000, -0.8700118002898359348, 0.4930308989875165082 ) ) ;
#158375=EDGE_LOOP ( 'NONE', ( #133338, #69179, #17448, #230498 ) ) ;
#158379=DIRECTION ( 'NONE',  ( 0.000000000000000000, 0.000000000000000000, -1.000000000000000000 ) ) ;
#158392=ORIENTED_EDGE ( 'NONE', *, *, #246065, .F. ) ;
#158531=DIRECTION ( 'NONE',  ( 0.000000000000000000, -0.1455152366551522025, -0.9893560106964505163 ) ) ;
#158537=ADVANCED_FACE ( 'NONE', ( #29981 ), #77413, .T. ) ;
#158561=AXIS2_PLACEMENT_3D ( 'NONE', #101351, #195404, #98805 ) ;
#158624=VERTEX_POINT ( 'NONE', #76771 ) ;
#158656=EDGE_CURVE ( 'NONE', #250352, #47156, #185764, .T. ) ;
#158712=ORIENTED_EDGE ( 'NONE', *, *, #45576, .F. ) ;
#158727=DIRECTION ( 'NONE',  ( 0.000000000000000000, 0.000000000000000000, -1.000000000000000000 ) ) ;
#158732=AXIS2_PLACEMENT_3D ( 'NONE', #149764, #164179, #66355 ) ;
#158746=DIRECTION ( 'NONE',  ( -0.000000000000000000, -1.000000000000000000, -0.000000000000000000 ) ) ;
#158763=CARTESIAN_POINT ( 'NONE',  ( -20.94999999999999929, 11.59999999999999609, -6.928203230275558511 ) ) ;
#158777=LINE ( 'NONE', #102588, #212123 ) ;
#158793=AXIS2_PLACEMENT_3D ( 'NONE', #137516, #198788, #117974 ) ;
#158813=CARTESIAN_POINT ( 'NONE',  ( 22.49999999999999645, 0.09999999999999939493, 11.64957080754480323 ) ) ;
#158831=EDGE_LOOP ( 'NONE', ( #174624, #152837, #68086, #21611 ) ) ;
#158841=VERTEX_POINT ( 'NONE', #167899 ) ;
#158861=DIRECTION ( 'NONE',  ( 0.000000000000000000, 1.000000000000000000, 0.000000000000000000 ) ) ;
#158892=CARTESIAN_POINT ( 'NONE',  ( 21.05000000000000071, -11.64999999999999147, -30.59999999999999432 ) ) ;
#158914=DIRECTION ( 'NONE',  ( 0.000000000000000000, 0.000000000000000000, 1.000000000000000000 ) ) ;
#158940=VERTEX_POINT ( 'NONE', #174338 ) ;
#158948=CARTESIAN_POINT ( 'NONE',  ( -18.50000000000000355, -1.263275465217258198, -41.40186466674640542 ) ) ;
#158963=EDGE_CURVE ( 'NONE', #125216, #222808, #218517, .T. ) ;
#159000=ORIENTED_EDGE ( 'NONE', *, *, #187147, .F. ) ;
#159021=CARTESIAN_POINT ( 'NONE',  ( -20.54999999999999716, -11.75000000000000178, -12.35000000000000675 ) ) ;
#159028=LINE ( 'NONE', #220271, #120405 ) ;
#159051=EDGE_LOOP ( 'NONE', ( #96097, #175936, #4613, #159166, #162206, #77551, #151861, #89476, #221610, #93007, #32257, #202199, #255135, #4280 ) ) ;
#159055=CARTESIAN_POINT ( 'NONE',  ( -23.24999999999999645, -9.600000000000003197, -40.10018939122204529 ) ) ;
#159091=ORIENTED_EDGE ( 'NONE', *, *, #22064, .T. ) ;
#159108=CARTESIAN_POINT ( 'NONE',  ( 23.25000000000000000, -11.74999999999999112, -30.39999999999999858 ) ) ;
#159112=CARTESIAN_POINT ( 'NONE',  ( -23.25000000000000000, 0.000000000000000000, -4.149999999999999467 ) ) ;
#159124=DIRECTION ( 'NONE',  ( 0.000000000000000000, -1.000000000000000000, 0.000000000000000000 ) ) ;
#159152=( BOUNDED_SURFACE ( )  B_SPLINE_SURFACE ( 3, 2, ( 
 ( #247581, #213579, #51919 ),
 ( #53231, #118008, #228021 ),
 ( #173229, #212327, #70262 ),
 ( #34992, #149792, #229313 ),
 ( #72826, #192754, #151058 ),
 ( #170667, #230596, #113202 ),
 ( #168090, #91075, #152362 ),
 ( #188893, #31143, #252697 ),
 ( #88478, #131482, #231892 ),
 ( #32421, #89776, #169373 ) ),
 .UNSPECIFIED., .F., .F., .F. ) 
 B_SPLINE_SURFACE_WITH_KNOTS ( ( 4, 2, 2, 2, 4 ),
 ( 3, 3 ),
 ( 0.0001836757140119128328, 0.0004000170051583585109, 0.0005081876507315813635, 0.0005622729735181927627, 0.0006163582963048041619 ),
 ( 0.000000000000000000, 1.000000000000000000 ),
 .UNSPECIFIED. ) 
 GEOMETRIC_REPRESENTATION_ITEM ( )  RATIONAL_B_SPLINE_SURFACE ( (
 ( 1.000000000000000000, 0.7071067811865475727, 1.000000000000000000),
 ( 1.000000000000000000, 0.6461995200029642117, 1.000000000000000000),
 ( 1.000000000000000000, 0.5776453529549738786, 1.000000000000000000),
 ( 1.000000000000000000, 0.4585233068351608487, 1.000000000000000000),
 ( 1.000000000000000000, 0.4154092989935744829, 1.000000000000000000),
 ( 1.000000000000000000, 0.3550093145838208453, 1.000000000000000000),
 ( 1.000000000000000000, 0.3354498651685166033, 1.000000000000000000),
 ( 1.000000000000000000, 0.3060347992257089755, 1.000000000000000000),
 ( 1.000000000000000000, 0.2963555829625726945, 1.000000000000000000),
 ( 1.000000000000000000, 0.2966190024560417804, 1.000000000000000000) ) ) 
 REPRESENTATION_ITEM ( '' )  SURFACE ( )  );
#159155=CARTESIAN_POINT ( 'NONE',  ( -21.14999999999999858, 0.000000000000000000, 6.258578643762700011 ) ) ;
#159156=AXIS2_PLACEMENT_3D ( 'NONE', #242196, #44002, #163961 ) ;
#159166=ORIENTED_EDGE ( 'NONE', *, *, #107989, .F. ) ;
#159171=ADVANCED_FACE ( 'NONE', ( #128436 ), #185835, .T. ) ;
#159172=ORIENTED_EDGE ( 'NONE', *, *, #147089, .T. ) ;
#159182=DIRECTION ( 'NONE',  ( 0.000000000000000000, 0.000000000000000000, -1.000000000000000000 ) ) ;
#159220=ORIENTED_EDGE ( 'NONE', *, *, #114190, .T. ) ;
#159254=DIRECTION ( 'NONE',  ( -0.000000000000000000, 1.000000000000000000, -0.000000000000000000 ) ) ;
#159265=FACE_OUTER_BOUND ( 'NONE', #37910, .T. ) ;
#159286=CIRCLE ( 'NONE', #238363, 0.09999999999999939493 ) ;
#159307=DIRECTION ( 'NONE',  ( -5.603264701231743991E-32, 1.897661533703519897E-16, -1.000000000000000000 ) ) ;
#159312=DIRECTION ( 'NONE',  ( 1.000000000000000000, 0.000000000000000000, 0.000000000000000000 ) ) ;
#159317=CARTESIAN_POINT ( 'NONE',  ( -23.25000000000000000, 11.75000000000000000, -12.15000000000000036 ) ) ;
#159331=EDGE_LOOP ( 'NONE', ( #102759, #244452, #104424, #232453 ) ) ;
#159356=CARTESIAN_POINT ( 'NONE',  ( -21.44999999999999929, 7.349999999999998757, -21.25000000000000000 ) ) ;
#159380=DIRECTION ( 'NONE',  ( 0.000000000000000000, -0.3738317757009225195, 0.9274965247785541544 ) ) ;
#159391=ORIENTED_EDGE ( 'NONE', *, *, #13825, .T. ) ;
#159411=AXIS2_PLACEMENT_3D ( 'NONE', #214393, #213107, #231405 ) ;
#159432=CARTESIAN_POINT ( 'NONE',  ( 18.49999999999999289, 10.24999999999999822, -21.35000000000000142 ) ) ;
#159438=CARTESIAN_POINT ( 'NONE',  ( -20.94788355080264353, 10.30207779524867462, -38.98955207167824000 ) ) ;
#159454=CIRCLE ( 'NONE', #46997, 0.09999999999999961697 ) ;
#159479=DIRECTION ( 'NONE',  ( -0.000000000000000000, 0.9274965247785350586, 0.3738317757009704811 ) ) ;
#159484=VECTOR ( 'NONE', #198142, 1000.000000000000000 ) ;
#159535=DIRECTION ( 'NONE',  ( 0.000000000000000000, 1.000000000000000000, -0.000000000000000000 ) ) ;
#159536=ORIENTED_EDGE ( 'NONE', *, *, #245643, .T. ) ;
#159538=CARTESIAN_POINT ( 'NONE',  ( 21.14999999999999503, 0.000000000000000000, 0.000000000000000000 ) ) ;
#159584=CARTESIAN_POINT ( 'NONE',  ( -22.39999999999999858, 0.09999999999999939493, 0.000000000000000000 ) ) ;
#159587=FACE_OUTER_BOUND ( 'NONE', #173605, .T. ) ;
#159625=ORIENTED_EDGE ( 'NONE', *, *, #202221, .F. ) ;
#159627=CARTESIAN_POINT ( 'NONE',  ( -21.53752568622134689, 0.09897446126636658126, 6.786807874548587804 ) ) ;
#159654=AXIS2_PLACEMENT_3D ( 'NONE', #129644, #209176, #219429 ) ;
#159679=DIRECTION ( 'NONE',  ( 0.000000000000000000, 0.000000000000000000, -1.000000000000000000 ) ) ;
#159684=CARTESIAN_POINT ( 'NONE',  ( -18.59999999999999787, 11.60000000000000320, -6.928203230275554958 ) ) ;
#159811=ORIENTED_EDGE ( 'NONE', *, *, #229025, .F. ) ;
#159881=CARTESIAN_POINT ( 'NONE',  ( 20.94999999999999929, -9.000000000000000000, -23.60603087734755690 ) ) ;
#159903=CARTESIAN_POINT ( 'NONE',  ( 21.30000000000002558, 0.000000000000000000, 0.000000000000000000 ) ) ;
#159910=DIRECTION ( 'NONE',  ( 1.000000000000000000, 0.000000000000000000, 0.000000000000000000 ) ) ;
#159943=EDGE_CURVE ( 'NONE', #72309, #224010, #214735, .T. ) ;
#159947=DIRECTION ( 'NONE',  ( 0.000000000000000000, 0.000000000000000000, -1.000000000000000000 ) ) ;
#159961=DIRECTION ( 'NONE',  ( 1.000000000000000000, -0.000000000000000000, -0.000000000000000000 ) ) ;
#159975=VERTEX_POINT ( 'NONE', #15278 ) ;
#159988=CARTESIAN_POINT ( 'NONE',  ( -20.94999999999999929, 7.120270961697594103, -37.15956304183931991 ) ) ;
#160000=VERTEX_POINT ( 'NONE', #223706 ) ;
#160002=ADVANCED_FACE ( 'NONE', ( #182038 ), #219619, .T. ) ;
#160018=ORIENTED_EDGE ( 'NONE', *, *, #75518, .F. ) ;
#160036=EDGE_CURVE ( 'NONE', #184931, #93175, #177952, .T. ) ;
#160058=AXIS2_PLACEMENT_3D ( 'NONE', #34143, #112370, #255669 ) ;
#160061=CARTESIAN_POINT ( 'NONE',  ( 21.05000000000000071, 6.496686585767979416, -0.01465611851322024678 ) ) ;
#160078=CARTESIAN_POINT ( 'NONE',  ( 21.04999999999999716, 0.01471785652413675274, 6.344723404090222729 ) ) ;
#160087=CARTESIAN_POINT ( 'NONE',  ( -23.15000000000000213, 11.65000000000000036, -21.34999999999999787 ) ) ;
#160092=DIRECTION ( 'NONE',  ( 1.000000000000000000, -0.000000000000000000, -0.000000000000000000 ) ) ;
#160191=CIRCLE ( 'NONE', #126846, 0.1000000000000001305 ) ;
#160197=EDGE_CURVE ( 'NONE', #11112, #67142, #111482, .T. ) ;
#160211=CARTESIAN_POINT ( 'NONE',  ( -22.59999999999999787, 11.74956712348939192, 0.1008583690987087389 ) ) ;
#160219=DIRECTION ( 'NONE',  ( 0.000000000000000000, -1.000000000000000000, -0.000000000000000000 ) ) ;
#160225=ORIENTED_EDGE ( 'NONE', *, *, #35631, .T. ) ;
#160239=LINE ( 'NONE', #241042, #22570 ) ;
#160258=DIRECTION ( 'NONE',  ( 0.000000000000000000, 0.000000000000000000, -1.000000000000000000 ) ) ;
#160266=CARTESIAN_POINT ( 'NONE',  ( -23.25000000000000000, 1.999999999999998224, -20.87537807723790095 ) ) ;
#160270=ORIENTED_EDGE ( 'NONE', *, *, #124467, .T. ) ;
#160279=CARTESIAN_POINT ( 'NONE',  ( 20.97250901189795513, 10.62456803370188041, -7.664545716966992828 ) ) ;
#160295=ORIENTED_EDGE ( 'NONE', *, *, #25811, .F. ) ;
#160308=CIRCLE ( 'NONE', #193594, 0.09999999999999939493 ) ;
#160332=VERTEX_POINT ( 'NONE', #252260 ) ;
#160347=DIRECTION ( 'NONE',  ( -1.000000000000000000, -7.304098846218134667E-16, 4.217023435051678980E-16 ) ) ;
#160353=VECTOR ( 'NONE', #245980, 1000.000000000000000 ) ;
#160354=ORIENTED_EDGE ( 'NONE', *, *, #58089, .F. ) ;
#160365=FACE_OUTER_BOUND ( 'NONE', #118500, .T. ) ;
#160456=ORIENTED_EDGE ( 'NONE', *, *, #107950, .F. ) ;
#160466=ADVANCED_FACE ( 'NONE', ( #23958 ), #248114, .T. ) ;
#160492=ORIENTED_EDGE ( 'NONE', *, *, #191753, .F. ) ;
#160505=CARTESIAN_POINT ( 'NONE',  ( 18.49999999999999645, 5.949999999999945111, -10.30570230503485796 ) ) ;
#160534=CIRCLE ( 'NONE', #68946, 0.1999999999999987899 ) ;
#160551=EDGE_CURVE ( 'NONE', #158841, #141135, #210292, .T. ) ;
#160561=ADVANCED_FACE ( 'NONE', ( #109879 ), #190749, .F. ) ;
#160580=EDGE_CURVE ( 'NONE', #108404, #5236, #70197, .T. ) ;
#160593=EDGE_CURVE ( 'NONE', #66484, #210865, #215875, .T. ) ;
#160603=DIRECTION ( 'NONE',  ( 1.000000000000000000, 0.000000000000000000, 0.000000000000000000 ) ) ;
#160608=DIRECTION ( 'NONE',  ( 9.044546369203339308E-15, -0.7397360091702694929, -0.6728971962616898672 ) ) ;
#160618=AXIS2_PLACEMENT_3D ( 'NONE', #130782, #193346, #113787 ) ;
#160685=( BOUNDED_SURFACE ( )  B_SPLINE_SURFACE ( 3, 2, ( 
 ( #210659, #91988, #90701 ),
 ( #170298, #249788, #32052 ),
 ( #191125, #13746, #28208 ),
 ( #251055, #72452, #67294 ),
 ( #231521, #107703, #187265 ),
 ( #39757, #35897, #218337 ) ),
 .UNSPECIFIED., .F., .F., .T. ) 
 B_SPLINE_SURFACE_WITH_KNOTS ( ( 4, 2, 4 ),
 ( 3, 3 ),
 ( 0.0001381104793128061785, 0.0002947094729387687547, 0.0004513084665647313309 ),
 ( 0.000000000000000000, 1.000000000000000000 ),
 .UNSPECIFIED. ) 
 GEOMETRIC_REPRESENTATION_ITEM ( )  RATIONAL_B_SPLINE_SURFACE ( (
 ( 1.000000000000000000, 0.7071067811865494601, 1.000000000000000000),
 ( 1.000000000000000000, 0.6919563088099097703, 1.000000000000000000),
 ( 1.000000000000000000, 0.6959445945717440685, 1.000000000000000000),
 ( 1.000000000000000000, 0.7137882985313291906, 1.000000000000000000),
 ( 1.000000000000000000, 0.7257496306096434813, 1.000000000000000000),
 ( 1.000000000000000000, 0.7250110520819876836, 1.000000000000000000) ) ) 
 REPRESENTATION_ITEM ( '' )  SURFACE ( )  );
#160703=CIRCLE ( 'NONE', #131436, 0.1999999999999987899 ) ;
#160704=ORIENTED_EDGE ( 'NONE', *, *, #198695, .T. ) ;
#160735=AXIS2_PLACEMENT_3D ( 'NONE', #41703, #62537, #39143 ) ;
#160758=EDGE_CURVE ( 'NONE', #111888, #109469, #120209, .T. ) ;
#160795=CIRCLE ( 'NONE', #144002, 2.000000000000002665 ) ;
#160827=DIRECTION ( 'NONE',  ( -0.7071067811865474617, 0.7071067811865474617, 0.000000000000000000 ) ) ;
#160840=CARTESIAN_POINT ( 'NONE',  ( 20.94999999999999929, 0.000000000000000000, -33.50000000000000000 ) ) ;
#160845=ORIENTED_EDGE ( 'NONE', *, *, #151334, .T. ) ;
#160869=SPHERICAL_SURFACE ( 'NONE', #103345, 0.1000000000000000056 ) ;
#160871=AXIS2_PLACEMENT_3D ( 'NONE', #214914, #57098, #256552 ) ;
#160896=LINE ( 'NONE', #137439, #144308 ) ;
#160937=ORIENTED_EDGE ( 'NONE', *, *, #231207, .F. ) ;
#160951=AXIS2_PLACEMENT_3D ( 'NONE', #30641, #232688, #110148 ) ;
#160963=EDGE_CURVE ( 'NONE', #230288, #219800, #232675, .T. ) ;
#160965=ORIENTED_EDGE ( 'NONE', *, *, #112499, .T. ) ;
#160971=EDGE_CURVE ( 'NONE', #143516, #174236, #252369, .T. ) ;
#160977=DIRECTION ( 'NONE',  ( 0.000000000000000000, 0.000000000000000000, -1.000000000000000000 ) ) ;
#160986=AXIS2_PLACEMENT_3D ( 'NONE', #12230, #30507, #232567 ) ;
#161001=CARTESIAN_POINT ( 'NONE',  ( -20.94999999999999929, 7.031312794755200102, -37.10915093822730881 ) ) ;
#161021=ORIENTED_EDGE ( 'NONE', *, *, #80195, .F. ) ;
#161040=CARTESIAN_POINT ( 'NONE',  ( 18.58222699835054570, 10.33200063079656772, -39.09316749566428939 ) ) ;
#161041=DIRECTION ( 'NONE',  ( 0.000000000000000000, 0.000000000000000000, -1.000000000000000000 ) ) ;
#161044=LINE ( 'NONE', #220992, #44852 ) ;
#161053=ORIENTED_EDGE ( 'NONE', *, *, #14446, .F. ) ;
#161060=LINE ( 'NONE', #240586, #51611 ) ;
#161067=DIRECTION ( 'NONE',  ( -0.000000000000000000, -1.000000000000000000, 6.308085367188393199E-16 ) ) ;
#161077=VERTEX_POINT ( 'NONE', #36505 ) ;
#161107=DIRECTION ( 'NONE',  ( 0.000000000000000000, 0.000000000000000000, -1.000000000000000000 ) ) ;
#161140=CARTESIAN_POINT ( 'NONE',  ( -23.15000000000000213, 0.000000000000000000, -33.50000000000000000 ) ) ;
#161146=EDGE_CURVE ( 'NONE', #176380, #26537, #253491, .T. ) ;
#161151=LINE ( 'NONE', #3327, #128451 ) ;
#161159=AXIS2_PLACEMENT_3D ( 'NONE', #38530, #118056, #649 ) ;
#161180=CARTESIAN_POINT ( 'NONE',  ( -20.54999999999999716, 1.925233644859811521, -20.76975646687386501 ) ) ;
#161225=FACE_OUTER_BOUND ( 'NONE', #240665, .T. ) ;
#161247=EDGE_CURVE ( 'NONE', #56184, #112707, #45398, .T. ) ;
#161279=CARTESIAN_POINT ( 'NONE',  ( -23.15000000000000213, 0.000000000000000000, -33.50000000000000000 ) ) ;
#161291=CARTESIAN_POINT ( 'NONE',  ( -22.39999999999999858, -1.124859753953710850E-15, 11.64957080754479968 ) ) ;
#161360=CARTESIAN_POINT ( 'NONE',  ( 23.15000000000000213, -11.64999999999999147, 11.75000000000000000 ) ) ;
#161361=DIRECTION ( 'NONE',  ( -1.000000000000000000, 0.000000000000000000, 0.000000000000000000 ) ) ;
#161448=VECTOR ( 'NONE', #173736, 1000.000000000000000 ) ;
#161460=CIRCLE ( 'NONE', #253201, 0.4000000000000010214 ) ;
#161461=CARTESIAN_POINT ( 'NONE',  ( 18.59999999999999432, -1.162701749938009677, -8.099999999999999645 ) ) ;
#161471=CIRCLE ( 'NONE', #86406, 0.09999999999999939493 ) ;
#161473=CYLINDRICAL_SURFACE ( 'NONE', #233597, 0.09999999999999939493 ) ;
#161486=CARTESIAN_POINT ( 'NONE',  ( -21.07094088545303734, 6.320167221916481282, 0.09889370255222133810 ) ) ;
#161496=ORIENTED_EDGE ( 'NONE', *, *, #250511, .F. ) ;
#161501=VERTEX_POINT ( 'NONE', #215744 ) ;
#161513=CARTESIAN_POINT ( 'NONE',  ( -18.50000000000000000, -1.135018845910178431, -41.21697688343231647 ) ) ;
#161529=DIRECTION ( 'NONE',  ( 1.000000000000000000, -0.000000000000000000, -0.000000000000000000 ) ) ;
#161574=VERTEX_POINT ( 'NONE', #121813 ) ;
#161622=AXIS2_PLACEMENT_3D ( 'NONE', #257559, #162389, #219764 ) ;
#161659=CARTESIAN_POINT ( 'NONE',  ( 21.05000000000000071, 0.000000000000000000, 0.000000000000000000 ) ) ;
#161679=SPHERICAL_SURFACE ( 'NONE', #109718, 0.1000000000000000056 ) ;
#161695=ORIENTED_EDGE ( 'NONE', *, *, #104678, .T. ) ;
#161731=CARTESIAN_POINT ( 'NONE',  ( -21.45000000000000284, 7.708578643762696636, -12.25000000000000000 ) ) ;
#161763=ORIENTED_EDGE ( 'NONE', *, *, #61792, .F. ) ;
#161766=VECTOR ( 'NONE', #87743, 1000.000000000000000 ) ;
#161801=EDGE_CURVE ( 'NONE', #91362, #161574, #224070, .T. ) ;
#161802=ORIENTED_EDGE ( 'NONE', *, *, #161801, .T. ) ;
#161840=DIRECTION ( 'NONE',  ( 0.000000000000000000, 0.9887567792719341719, -0.1495327102803664099 ) ) ;
#161853=DIRECTION ( 'NONE',  ( 0.000000000000000000, 0.5000000000000209832, 0.8660254037844264952 ) ) ;
#161868=EDGE_CURVE ( 'NONE', #168114, #227236, #53389, .T. ) ;
#161896=TOROIDAL_SURFACE ( 'NONE', #124466, 0.6000000000000013101, 0.1000000000000000056 ) ;
#161921=CARTESIAN_POINT ( 'NONE',  ( -18.59999999999999787, 1.162701749938009677, -8.000000000000000000 ) ) ;
#161929=AXIS2_PLACEMENT_3D ( 'NONE', #191078, #249744, #188479 ) ;
#161946=CARTESIAN_POINT ( 'NONE',  ( -18.59999999999999787, -9.480686695278977894, -40.44111516875783963 ) ) ;
#161980=DIRECTION ( 'NONE',  ( 0.000000000000000000, 0.000000000000000000, -1.000000000000000000 ) ) ;
#161982=AXIS2_PLACEMENT_3D ( 'NONE', #200648, #122394, #221461 ) ;
#161995=DIRECTION ( 'NONE',  ( 0.000000000000000000, 0.000000000000000000, 1.000000000000000000 ) ) ;
#162006=LINE ( 'NONE', #5447, #113914 ) ;
#162046=CARTESIAN_POINT ( 'NONE',  ( -21.59142135623730852, 7.850000000000003197, -12.25000000000000000 ) ) ;
#162053=DIRECTION ( 'NONE',  ( 0.000000000000000000, -0.000000000000000000, 1.000000000000000000 ) ) ;
#162067=ORIENTED_EDGE ( 'NONE', *, *, #235110, .T. ) ;
#162068=AXIS2_PLACEMENT_3D ( 'NONE', #121509, #139737, #43234 ) ;
#162106=CARTESIAN_POINT ( 'NONE',  ( 21.97500000000000497, 9.749999999999998224, -12.25000000000000178 ) ) ;
#162171=SPHERICAL_SURFACE ( 'NONE', #58928, 0.1000000000000000056 ) ;
#162176=ORIENTED_EDGE ( 'NONE', *, *, #153156, .F. ) ;
#162192=CARTESIAN_POINT ( 'NONE',  ( -18.56579813702275672, 10.33025634371521662, -39.08709292826389259 ) ) ;
#162193=LINE ( 'NONE', #242979, #110294 ) ;
#162206=ORIENTED_EDGE ( 'NONE', *, *, #175617, .T. ) ;
#162211=EDGE_CURVE ( 'NONE', #150376, #75474, #174434, .T. ) ;
#162225=EDGE_LOOP ( 'NONE', ( #130849, #129854, #256219, #228279 ) ) ;
#162247=LINE ( 'NONE', #241753, #107690 ) ;
#162251=CARTESIAN_POINT ( 'NONE',  ( -18.50000000000000000, 11.75000000000000000, -12.14999999999999680 ) ) ;
#162320=CARTESIAN_POINT ( 'NONE',  ( -20.85000000000000142, -1.249999999999999334, -41.30048075441508360 ) ) ;
#162360=AXIS2_PLACEMENT_3D ( 'NONE', #178408, #60986, #76698 ) ;
#162362=DIRECTION ( 'NONE',  ( -0.000000000000000000, 0.8660254037844411501, 0.4999999999999956701 ) ) ;
#162383=DIRECTION ( 'NONE',  ( 1.000000000000000000, 2.952720810173289112E-16, -0.000000000000000000 ) ) ;
#162384=ORIENTED_EDGE ( 'NONE', *, *, #40912, .F. ) ;
#162389=DIRECTION ( 'NONE',  ( -1.000000000000000000, 0.000000000000000000, 0.000000000000000000 ) ) ;
#162390=ORIENTED_EDGE ( 'NONE', *, *, #183769, .T. ) ;
#162391=DIRECTION ( 'NONE',  ( 8.673617379884087537E-15, -0.000000000000000000, 1.000000000000000000 ) ) ;
#162406=ORIENTED_EDGE ( 'NONE', *, *, #169165, .T. ) ;
#162407=DIRECTION ( 'NONE',  ( 1.000000000000000000, 0.000000000000000000, -0.000000000000000000 ) ) ;
#162411=ORIENTED_EDGE ( 'NONE', *, *, #29329, .F. ) ;
#162418=CARTESIAN_POINT ( 'NONE',  ( 20.94999999999999929, 0.000000000000000000, -33.50000000000000000 ) ) ;
#162426=VECTOR ( 'NONE', #163447, 1000.000000000000000 ) ;
#162495=VERTEX_POINT ( 'NONE', #251763 ) ;
#162506=DIRECTION ( 'NONE',  ( -0.000000000000000000, 1.000000000000000000, 1.626303258728266709E-15 ) ) ;
#162551=EDGE_CURVE ( 'NONE', #6193, #62328, #71864, .T. ) ;
#162560=AXIS2_PLACEMENT_3D ( 'NONE', #44195, #81985, #182425 ) ;
#162565=DIRECTION ( 'NONE',  ( -1.000000000000000000, 0.000000000000000000, 0.000000000000000000 ) ) ;
#162595=CARTESIAN_POINT ( 'NONE',  ( 21.05000000000000426, 0.03486800301310592765, 6.270085863689147665 ) ) ;
#162596=DIRECTION ( 'NONE',  ( 0.000000000000000000, 0.1350103645451876666, -0.9908441862701600211 ) ) ;
#162613=CARTESIAN_POINT ( 'NONE',  ( 21.05000000000000426, 6.299230910086890844, 0.09843749999999837352 ) ) ;
#162626=VERTEX_POINT ( 'NONE', #169707 ) ;
#162662=ORIENTED_EDGE ( 'NONE', *, *, #565, .F. ) ;
#162712=EDGE_CURVE ( 'NONE', #14945, #199652, #119991, .T. ) ;
#162776=ORIENTED_EDGE ( 'NONE', *, *, #234230, .T. ) ;
#162799=ORIENTED_EDGE ( 'NONE', *, *, #25832, .F. ) ;
#162808=CARTESIAN_POINT ( 'NONE',  ( 20.94999999999999929, -9.400000000000000355, -23.60603087734755690 ) ) ;
#162809=CARTESIAN_POINT ( 'NONE',  ( -21.64999999999999858, 7.349999999999998757, -12.34999999999999964 ) ) ;
#162818=AXIS2_PLACEMENT_3D ( 'NONE', #106746, #28561, #49356 ) ;
#162832=DIRECTION ( 'NONE',  ( 2.952720810173289112E-16, -1.000000000000000000, 0.000000000000000000 ) ) ;
#162847=CARTESIAN_POINT ( 'NONE',  ( 21.04999999999999716, 6.304455821947667182, -0.02103547654011554344 ) ) ;
#162848=LINE ( 'NONE', #183684, #233445 ) ;
#162851=TOROIDAL_SURFACE ( 'NONE', #158561, 0.2000000000000000111, 0.1000000000000000056 ) ;
#162861=CARTESIAN_POINT ( 'NONE',  ( -18.59999999999999787, 9.250000000000001776, -21.25000000000000000 ) ) ;
#162890=DIRECTION ( 'NONE',  ( 2.952720810173289112E-16, -1.000000000000000000, 0.000000000000000000 ) ) ;
#162899=ORIENTED_EDGE ( 'NONE', *, *, #145237, .T. ) ;
#162940=CARTESIAN_POINT ( 'NONE',  ( -18.59999999999999787, 11.64999999999999680, -7.014805770654001016 ) ) ;
#162975=VERTEX_POINT ( 'NONE', #192773 ) ;
#163009=VERTEX_POINT ( 'NONE', #91097 ) ;
#163026=DIRECTION ( 'NONE',  ( 0.000000000000000000, -1.000000000000000000, 0.000000000000000000 ) ) ;
#163039=VERTEX_POINT ( 'NONE', #53260 ) ;
#163078=LINE ( 'NONE', #197025, #111847 ) ;
#163102=EDGE_LOOP ( 'NONE', ( #168570, #144878, #91546, #20703 ) ) ;
#163104=EDGE_LOOP ( 'NONE', ( #89057, #54132, #201155, #225190, #217969 ) ) ;
#163105=DIRECTION ( 'NONE',  ( 1.000000000000000000, 0.000000000000000000, 0.000000000000000000 ) ) ;
#163109=EDGE_CURVE ( 'NONE', #106103, #37010, #135338, .T. ) ;
#163113=ORIENTED_EDGE ( 'NONE', *, *, #188454, .T. ) ;
#163119=ORIENTED_EDGE ( 'NONE', *, *, #81221, .F. ) ;
#163134=ORIENTED_EDGE ( 'NONE', *, *, #257779, .F. ) ;
#163150=DIRECTION ( 'NONE',  ( 0.000000000000000000, -0.9915357197604882655, 0.1298341882519793711 ) ) ;
#163155=CARTESIAN_POINT ( 'NONE',  ( -20.64999999999999858, 7.249999999999999112, -21.25000000000000000 ) ) ;
#163161=ADVANCED_FACE ( 'NONE', ( #136624 ), #236698, .T. ) ;
#163191=CARTESIAN_POINT ( 'NONE',  ( 21.10257677756356287, 0.02495074956798263091, 6.398381742532735394 ) ) ;
#163199=LINE ( 'NONE', #242711, #114910 ) ;
#163200=VERTEX_POINT ( 'NONE', #84303 ) ;
#163232=CIRCLE ( 'NONE', #71650, 0.09999999999999939493 ) ;
#163264=PRODUCT_DEFINITION ( 'UNKNOWN', '', #257000, #204299 ) ;
#163285=CARTESIAN_POINT ( 'NONE',  ( -20.94983749550516450, 10.29766095124176850, -38.97436639332756414 ) ) ;
#163286=DIRECTION ( 'NONE',  ( -1.000000000000000000, 0.000000000000000000, 0.000000000000000000 ) ) ;
#163291=DIRECTION ( 'NONE',  ( 1.000000000000000000, 0.000000000000000000, 0.000000000000000000 ) ) ;
#163327=EDGE_CURVE ( 'NONE', #77399, #249368, #71243, .T. ) ;
#163332=CARTESIAN_POINT ( 'NONE',  ( -21.14999999999999858, 11.64999999999999680, 0.000000000000000000 ) ) ;
#163398=ORIENTED_EDGE ( 'NONE', *, *, #186775, .F. ) ;
#163426=VERTEX_POINT ( 'NONE', #78897 ) ;
#163427=ORIENTED_EDGE ( 'NONE', *, *, #195148, .F. ) ;
#163428=FACE_OUTER_BOUND ( 'NONE', #191337, .T. ) ;
#163432=SHAPE_REPRESENTATION_RELATIONSHIP ( 'NONE' , 'NONE' ,  #168659, #157328 ) ;
#163447=DIRECTION ( 'NONE',  ( 1.000000000000000000, -0.000000000000000000, -0.000000000000000000 ) ) ;
#163492=ORIENTED_EDGE ( 'NONE', *, *, #171322, .F. ) ;
#163505=ORIENTED_EDGE ( 'NONE', *, *, #151561, .T. ) ;
#163531=ORIENTED_EDGE ( 'NONE', *, *, #174718, .T. ) ;
#163576=DIRECTION ( 'NONE',  ( 1.000000000000000000, 0.000000000000000000, 0.000000000000000000 ) ) ;
#163583=DIRECTION ( 'NONE',  ( 1.000000000000000000, 0.000000000000000000, -0.000000000000000000 ) ) ;
#163589=CIRCLE ( 'NONE', #85003, 0.1000000000000000472 ) ;
#163602=AXIS2_PLACEMENT_3D ( 'NONE', #33847, #212448, #12978 ) ;
#163606=CARTESIAN_POINT ( 'NONE',  ( 18.50016250449482413, 10.29766095124067249, -38.97436639332788388 ) ) ;
#163616=EDGE_CURVE ( 'NONE', #71227, #83974, #106172, .T. ) ;
#163627=CARTESIAN_POINT ( 'NONE',  ( -23.15000000000000213, 11.75000000000000000, -21.35000000000000142 ) ) ;
#163632=CARTESIAN_POINT ( 'NONE',  ( 21.14999999999999858, 11.65000000000000391, -0.1000000000000028644 ) ) ;
#163657=EDGE_CURVE ( 'NONE', #217421, #89621, #71070, .T. ) ;
#163676=DIRECTION ( 'NONE',  ( -0.000000000000000000, -0.4791956752371546724, -0.8777080977375153470 ) ) ;
#163679=CARTESIAN_POINT ( 'NONE',  ( 23.14999999999999858, 3.999999999999999112, -33.50000000000000000 ) ) ;
#163711=DIRECTION ( 'NONE',  ( 1.000000000000000000, 0.000000000000000000, 0.000000000000000000 ) ) ;
#163748=DIRECTION ( 'NONE',  ( -1.000000000000000000, 0.000000000000000000, 0.000000000000000000 ) ) ;
#163762=VECTOR ( 'NONE', #246436, 1000.000000000000000 ) ;
#163780=DIRECTION ( 'NONE',  ( 1.000000000000000000, 0.000000000000000000, 0.000000000000000000 ) ) ;
#163801=DIRECTION ( 'NONE',  ( -1.000000000000000000, 0.000000000000000000, 0.000000000000000000 ) ) ;
#163813=CARTESIAN_POINT ( 'NONE',  ( 21.05000000000000071, 0.000000000000000000, -33.50000000000000000 ) ) ;
#163829=VECTOR ( 'NONE', #109661, 1000.000000000000114 ) ;
#163833=CARTESIAN_POINT ( 'NONE',  ( 20.94999999999999929, 0.000000000000000000, -33.50000000000000000 ) ) ;
#163856=CARTESIAN_POINT ( 'NONE',  ( 22.49436431346199683, 11.64995094765345840, 0.06690352972225574457 ) ) ;
#163873=DIRECTION ( 'NONE',  ( 0.000000000000000000, 1.000000000000000000, -6.308085367188393199E-16 ) ) ;
#163922=ORIENTED_EDGE ( 'NONE', *, *, #184979, .F. ) ;
#163939=DIRECTION ( 'NONE',  ( -1.000000000000000000, 0.000000000000000000, 0.000000000000000000 ) ) ;
#163953=EDGE_CURVE ( 'NONE', #180993, #174426, #241912, .T. ) ;
#163960=ORIENTED_EDGE ( 'NONE', *, *, #8759, .F. ) ;
#163961=DIRECTION ( 'NONE',  ( 0.000000000000000000, 0.000000000000000000, -1.000000000000000000 ) ) ;
#163965=ORIENTED_EDGE ( 'NONE', *, *, #17806, .T. ) ;
#163970=CARTESIAN_POINT ( 'NONE',  ( 21.00000000000000000, 9.749999999999998224, -12.35000000000000320 ) ) ;
#163991=B_SPLINE_CURVE_WITH_KNOTS ( 'NONE', 3,
 ( #123590, #23231, #238397, #4892, #79304, #223954 ),
 .UNSPECIFIED., .F., .F.,
 ( 4, 2, 4 ),
 ( 0.000000000000000000, 0.0001496588209255839358, 0.0002993176418511678716 ),
 .UNSPECIFIED. ) ;
#164006=CYLINDRICAL_SURFACE ( 'NONE', #226537, 0.1000000000000000056 ) ;
#164009=CIRCLE ( 'NONE', #5570, 0.09999999999999939493 ) ;
#164043=VECTOR ( 'NONE', #122333, 1000.000000000000000 ) ;
#164047=CARTESIAN_POINT ( 'NONE',  ( -20.94999999999999929, 14.05000000000000071, -27.98630492923908619 ) ) ;
#164055=CIRCLE ( 'NONE', #255581, 0.2000000000000005107 ) ;
#164091=ORIENTED_EDGE ( 'NONE', *, *, #172204, .F. ) ;
#164155=FACE_OUTER_BOUND ( 'NONE', #108840, .T. ) ;
#164158=AXIS2_PLACEMENT_3D ( 'NONE', #224247, #48182, #105556 ) ;
#164179=DIRECTION ( 'NONE',  ( 0.000000000000000000, -1.000000000000000000, 0.000000000000000000 ) ) ;
#164201=VECTOR ( 'NONE', #1357, 1000.000000000000000 ) ;
#164216=ADVANCED_FACE ( 'NONE', ( #197929 ), #162851, .F. ) ;
#164217=ADVANCED_FACE ( 'NONE', ( #221331 ), #3664, .T. ) ;
#164261=AXIS2_PLACEMENT_3D ( 'NONE', #183141, #41074, #4476 ) ;
#164273=EDGE_CURVE ( 'NONE', #123641, #118795, #58918, .T. ) ;
#164301=CARTESIAN_POINT ( 'NONE',  ( 22.24259225415828567, 0.09906588345283645625, 7.491937870565415380 ) ) ;
#164305=AXIS2_PLACEMENT_3D ( 'NONE', #29418, #54073, #151922 ) ;
#164332=CARTESIAN_POINT ( 'NONE',  ( -23.25000000000000000, 11.65000000000000036, -21.25000000000000000 ) ) ;
#164346=ORIENTED_EDGE ( 'NONE', *, *, #60837, .F. ) ;
#164389=VERTEX_POINT ( 'NONE', #132530 ) ;
#164395=CARTESIAN_POINT ( 'NONE',  ( -18.50000000000000000, 9.250000000000001776, -21.35000000000000142 ) ) ;
#164415=CARTESIAN_POINT ( 'NONE',  ( 21.70464131381650219, 7.095358018967851343, 0.000000000000000000 ) ) ;
#164424=DIRECTION ( 'NONE',  ( 0.000000000000000000, 0.000000000000000000, -1.000000000000000000 ) ) ;
#164458=CARTESIAN_POINT ( 'NONE',  ( -20.05000000000000426, 9.250000000000001776, -21.15000000000000213 ) ) ;
#164475=DIRECTION ( 'NONE',  ( -1.000000000000000000, 0.000000000000000000, 0.000000000000000000 ) ) ;
#164477=EDGE_CURVE ( 'NONE', #22057, #214167, #108823, .T. ) ;
#164478=ORIENTED_EDGE ( 'NONE', *, *, #5267, .F. ) ;
#164510=EDGE_CURVE ( 'NONE', #126171, #63693, #96340, .T. ) ;
#164511=AXIS2_PLACEMENT_3D ( 'NONE', #99859, #179452, #80292 ) ;
#164524=DIRECTION ( 'NONE',  ( 1.000000000000000000, -0.000000000000000000, -0.000000000000000000 ) ) ;
#164570=EDGE_CURVE ( 'NONE', #216880, #208882, #79598, .T. ) ;
#164573=ORIENTED_EDGE ( 'NONE', *, *, #203042, .T. ) ;
#164580=FACE_OUTER_BOUND ( 'NONE', #126504, .T. ) ;
#164589=AXIS2_PLACEMENT_3D ( 'NONE', #16845, #238441, #134192 ) ;
#164604=AXIS2_PLACEMENT_3D ( 'NONE', #121619, #101992, #347 ) ;
#164616=EDGE_LOOP ( 'NONE', ( #133122, #56685, #75469, #159811 ) ) ;
#164630=DIRECTION ( 'NONE',  ( -1.000000000000000000, 0.000000000000000000, 0.000000000000000000 ) ) ;
#164665=LINE ( 'NONE', #145078, #242951 ) ;
#164692=DIRECTION ( 'NONE',  ( 0.000000000000000000, 0.000000000000000000, -1.000000000000000000 ) ) ;
#164718=AXIS2_PLACEMENT_3D ( 'NONE', #108844, #12346, #207973 ) ;
#164721=DIRECTION ( 'NONE',  ( -1.000000000000000000, 0.000000000000000000, 0.000000000000000000 ) ) ;
#164751=CARTESIAN_POINT ( 'NONE',  ( -20.87155475150660777, 11.74999999999999645, -26.59558652915735522 ) ) ;
#164754=ORIENTED_EDGE ( 'NONE', *, *, #243784, .T. ) ;
#164759=VECTOR ( 'NONE', #42439, 1000.000000000000000 ) ;
#164778=CARTESIAN_POINT ( 'NONE',  ( 18.59999999999999076, 10.20857864376269575, -21.35000000000000142 ) ) ;
#164785=ORIENTED_EDGE ( 'NONE', *, *, #70932, .T. ) ;
#164880=ORIENTED_EDGE ( 'NONE', *, *, #251111, .T. ) ;
#164900=DIRECTION ( 'NONE',  ( -7.304098846218201720E-16, 1.000000000000000000, 0.000000000000000000 ) ) ;
#164927=ADVANCED_FACE ( 'NONE', ( #11854 ), #13352, .T. ) ;
#164951=CARTESIAN_POINT ( 'NONE',  ( 23.14999999999999858, 0.000000000000000000, -12.87500000000000178 ) ) ;
#164961=AXIS2_PLACEMENT_3D ( 'NONE', #199141, #239554, #204256 ) ;
#164963=CARTESIAN_POINT ( 'NONE',  ( -20.94999999999999929, -1.835341550224411922, -11.55515129256298046 ) ) ;
#164994=CIRCLE ( 'NONE', #127403, 0.1000000000000028644 ) ;
#165039=TOROIDAL_SURFACE ( 'NONE', #181793, 2.100000000000002309, 0.1000000000000000056 ) ;
#165057=CARTESIAN_POINT ( 'NONE',  ( 20.94999999999999574, -1.349084418627015447, -7.986498963545480834 ) ) ;
#165094=DIRECTION ( 'NONE',  ( 1.000000000000000000, -0.000000000000000000, -0.000000000000000000 ) ) ;
#165127=VECTOR ( 'NONE', #155535, 1000.000000000000000 ) ;
#165134=AXIS2_PLACEMENT_3D ( 'NONE', #30687, #230140, #51470 ) ;
#165143=ADVANCED_FACE ( 'NONE', ( #135613 ), #234089, .T. ) ;
#165156=CARTESIAN_POINT ( 'NONE',  ( 22.59999999999999432, 0.09999999999999939493, 11.64957080754479968 ) ) ;
#165162=DIRECTION ( 'NONE',  ( 0.000000000000000000, 0.000000000000000000, 1.000000000000000000 ) ) ;
#165196=FACE_OUTER_BOUND ( 'NONE', #110791, .T. ) ;
#165206=VERTEX_POINT ( 'NONE', #254269 ) ;
#165215=DIRECTION ( 'NONE',  ( 0.000000000000000000, 0.4999999999999799605, -0.8660254037844502539 ) ) ;
#165218=DIRECTION ( 'NONE',  ( 0.000000000000000000, 0.000000000000000000, 1.000000000000000000 ) ) ;
#165287=DIRECTION ( 'NONE',  ( 1.000000000000000000, -7.304098846218134667E-16, 0.000000000000000000 ) ) ;
#165289=LINE ( 'NONE', #124884, #67907 ) ;
#165300=FACE_OUTER_BOUND ( 'NONE', #96042, .T. ) ;
#165327=DIRECTION ( 'NONE',  ( 0.000000000000000000, -0.5000000000000004441, -0.8660254037844384856 ) ) ;
#165333=ORIENTED_EDGE ( 'NONE', *, *, #75123, .T. ) ;
#165360=FACE_OUTER_BOUND ( 'NONE', #116600, .T. ) ;
#165367=CARTESIAN_POINT ( 'NONE',  ( -21.05000000000000071, 1.851028230140860487, -11.65391326942249606 ) ) ;
#165398=CARTESIAN_POINT ( 'NONE',  ( 21.05000000000000071, 0.000000000000000000, 0.000000000000000000 ) ) ;
#165400=CARTESIAN_POINT ( 'NONE',  ( 23.14999999999999503, 11.75000000000000711, -12.15000000000000036 ) ) ;
#165403=CARTESIAN_POINT ( 'NONE',  ( 21.05000000000000071, 4.850467289719620823, -21.46573259099832498 ) ) ;
#165405=VECTOR ( 'NONE', #142695, 1000.000000000000227 ) ;
#165422=CARTESIAN_POINT ( 'NONE',  ( 21.05000000000000071, -1.736257131597395809, -11.56865232901749785 ) ) ;
#165431=EDGE_CURVE ( 'NONE', #5236, #156221, #87343, .T. ) ;
#165456=ORIENTED_EDGE ( 'NONE', *, *, #222477, .T. ) ;
#165460=ORIENTED_EDGE ( 'NONE', *, *, #236139, .F. ) ;
#165467=AXIS2_PLACEMENT_3D ( 'NONE', #3043, #166021, #4329 ) ;
#165487=CIRCLE ( 'NONE', #194537, 0.1000000000000017958 ) ;
#165540=CARTESIAN_POINT ( 'NONE',  ( -18.59999999999999787, 11.64999999999999680, -7.014805770654001016 ) ) ;
#165555=CARTESIAN_POINT ( 'NONE',  ( 19.97071067811864609, 11.72071067811865674, -21.35000000000000142 ) ) ;
#165611=VECTOR ( 'NONE', #183382, 1000.000000000000000 ) ;
#165718=CARTESIAN_POINT ( 'NONE',  ( -21.09096482362056690, 0.03944827877415432726, 6.363544365404331771 ) ) ;
#165721=ORIENTED_EDGE ( 'NONE', *, *, #14037, .T. ) ;
#165725=DIRECTION ( 'NONE',  ( 0.000000000000000000, 0.000000000000000000, 1.000000000000000000 ) ) ;
#165738=CIRCLE ( 'NONE', #111543, 0.4000000000000010214 ) ;
#165758=AXIS2_PLACEMENT_3D ( 'NONE', #73527, #213001, #192178 ) ;
#165765=CARTESIAN_POINT ( 'NONE',  ( 18.59999999999998721, 6.933893972126341509, -37.28564583437357527 ) ) ;
#165766=ORIENTED_EDGE ( 'NONE', *, *, #69756, .F. ) ;
#165778=ADVANCED_FACE ( 'NONE', ( #235845 ), #42745, .T. ) ;
#165780=LINE ( 'NONE', #218315, #150421 ) ;
#165842=DIRECTION ( 'NONE',  ( 1.000000000000000000, 0.000000000000000000, 0.000000000000000000 ) ) ;
#165887=CIRCLE ( 'NONE', #136817, 0.09999999999999867328 ) ;
#165915=DIRECTION ( 'NONE',  ( 0.000000000000000000, 0.000000000000000000, -1.000000000000000000 ) ) ;
#165952=CARTESIAN_POINT ( 'NONE',  ( 21.05000000000000071, -11.74999999999999112, -30.39999999999999858 ) ) ;
#165987=AXIS2_PLACEMENT_3D ( 'NONE', #99541, #179143, #454 ) ;
#165989=VECTOR ( 'NONE', #37163, 1000.000000000000000 ) ;
#166014=DIRECTION ( 'NONE',  ( -1.000000000000000000, -0.000000000000000000, -0.000000000000000000 ) ) ;
#166021=DIRECTION ( 'NONE',  ( 1.000000000000000000, 2.952720810173289112E-16, -0.000000000000000000 ) ) ;
#166055=DIRECTION ( 'NONE',  ( -1.000000000000000000, 0.000000000000000000, 0.000000000000000000 ) ) ;
#166084=FACE_OUTER_BOUND ( 'NONE', #136635, .T. ) ;
#166115=CARTESIAN_POINT ( 'NONE',  ( 21.05000000000000426, 10.72371710470752149, -7.594417391613111690 ) ) ;
#166116=DIRECTION ( 'NONE',  ( -1.000000000000000000, 0.000000000000000000, 0.000000000000000000 ) ) ;
#166149=CARTESIAN_POINT ( 'NONE',  ( 23.14999999999999858, 4.999999999999997335, -21.09473398108690390 ) ) ;
#166168=ORIENTED_EDGE ( 'NONE', *, *, #24957, .F. ) ;
#166188=DIRECTION ( 'NONE',  ( 1.000000000000000000, 0.000000000000000000, 0.000000000000000000 ) ) ;
#166205=CARTESIAN_POINT ( 'NONE',  ( 18.50596464788227280, 10.30632246270533159, -39.00418367788959273 ) ) ;
#166251=DIRECTION ( 'NONE',  ( 1.000000000000000000, -0.000000000000000000, 0.000000000000000000 ) ) ;
#166253=EDGE_LOOP ( 'NONE', ( #51358, #97438, #175069, #123734 ) ) ;
#166267=EDGE_CURVE ( 'NONE', #84692, #184180, #167474, .T. ) ;
#166342=ORIENTED_EDGE ( 'NONE', *, *, #169503, .F. ) ;
#166401=ORIENTED_EDGE ( 'NONE', *, *, #198069, .T. ) ;
#166402=DIRECTION ( 'NONE',  ( 0.000000000000000000, 0.000000000000000000, -1.000000000000000000 ) ) ;
#166427=EDGE_LOOP ( 'NONE', ( #158038, #47864, #101486, #205718 ) ) ;
#166435=DIRECTION ( 'NONE',  ( -1.000000000000000000, -2.952720810173289112E-16, 0.000000000000000000 ) ) ;
#166458=CARTESIAN_POINT ( 'NONE',  ( 21.30740335185486245, 6.556657922028002794, 0.09893452577585087893 ) ) ;
#166465=DIRECTION ( 'NONE',  ( 0.000000000000000000, 6.308085367188394185E-16, 1.000000000000000000 ) ) ;
#166469=DIRECTION ( 'NONE',  ( 1.000000000000000000, 0.000000000000000000, -0.000000000000000000 ) ) ;
#166477=CARTESIAN_POINT ( 'NONE',  ( 18.41416235934318735, -9.499999999999998224, -40.10018939122204529 ) ) ;
#166478=CARTESIAN_POINT ( 'NONE',  ( 23.14999999999999858, 4.999999999999997335, -12.40526601891309788 ) ) ;
#166490=DIRECTION ( 'NONE',  ( 0.000000000000000000, 0.000000000000000000, -1.000000000000000000 ) ) ;
#166512=ORIENTED_EDGE ( 'NONE', *, *, #16461, .F. ) ;
#166515=CARTESIAN_POINT ( 'NONE',  ( 20.94999999999999929, 8.776282895292474961, -12.15000000000000036 ) ) ;
#166547=CARTESIAN_POINT ( 'NONE',  ( -21.00250684356850783, 11.74999999999999645, -7.014805768759292626 ) ) ;
#166550=VECTOR ( 'NONE', #94531, 1000.000000000000000 ) ;
#166580=VERTEX_POINT ( 'NONE', #89960 ) ;
#166597=DIRECTION ( 'NONE',  ( 0.000000000000000000, 0.000000000000000000, -1.000000000000000000 ) ) ;
#166618=CARTESIAN_POINT ( 'NONE',  ( -21.45000000000000284, 7.708578643762696636, -12.34999999999999964 ) ) ;
#166638=VERTEX_POINT ( 'NONE', #45708 ) ;
#166659=ORIENTED_EDGE ( 'NONE', *, *, #138023, .T. ) ;
#166668=PLANE ( 'NONE',  #134788 ) ;
#166678=DIRECTION ( 'NONE',  ( 1.000000000000000000, -0.000000000000000000, -0.000000000000000000 ) ) ;
#166708=DIRECTION ( 'NONE',  ( 0.000000000000000000, 0.000000000000000000, -1.000000000000000000 ) ) ;
#166723=FACE_OUTER_BOUND ( 'NONE', #195349, .T. ) ;
#166741=EDGE_CURVE ( 'NONE', #209763, #227236, #7889, .T. ) ;
#166760=ORIENTED_EDGE ( 'NONE', *, *, #35184, .T. ) ;
#166796=TOROIDAL_SURFACE ( 'NONE', #212573, 1.900000000000002576, 0.1000000000000000056 ) ;
#166852=VECTOR ( 'NONE', #80587, 1000.000000000000000 ) ;
#166871=EDGE_CURVE ( 'NONE', #156138, #167773, #75575, .T. ) ;
#166882=AXIS2_PLACEMENT_3D ( 'NONE', #10144, #213470, #131365 ) ;
#166896=CIRCLE ( 'NONE', #208575, 0.09999999999999939493 ) ;
#166901=DIRECTION ( 'NONE',  ( -0.7070776581709311559, 0.000000000000000000, 0.7071359030027479786 ) ) ;
#166915=CARTESIAN_POINT ( 'NONE',  ( 20.94999999999999929, 4.898587196589411843E-16, -29.50000000000000355 ) ) ;
#166917=ORIENTED_EDGE ( 'NONE', *, *, #250128, .F. ) ;
#166952=AXIS2_PLACEMENT_3D ( 'NONE', #184661, #8607, #6018 ) ;
#166967=EDGE_CURVE ( 'NONE', #177256, #113573, #147616, .T. ) ;
#166975=EDGE_LOOP ( 'NONE', ( #154471, #28713, #123188, #48151, #58188, #32536, #150888 ) ) ;
#167023=FACE_OUTER_BOUND ( 'NONE', #219920, .T. ) ;
#167091=CARTESIAN_POINT ( 'NONE',  ( 23.14999999999999858, 4.999999999999997335, -21.09473398108690390 ) ) ;
#167169=AXIS2_PLACEMENT_3D ( 'NONE', #72458, #189826, #247215 ) ;
#167187=ORIENTED_EDGE ( 'NONE', *, *, #177525, .F. ) ;
#167199=ORIENTED_EDGE ( 'NONE', *, *, #5267, .T. ) ;
#167207=DIRECTION ( 'NONE',  ( 1.000000000000000000, 0.000000000000000000, 0.000000000000000000 ) ) ;
#167261=ORIENTED_EDGE ( 'NONE', *, *, #125653, .F. ) ;
#167273=AXIS2_PLACEMENT_3D ( 'NONE', #228578, #49922, #186892 ) ;
#167317=EDGE_LOOP ( 'NONE', ( #127175, #201295, #174381, #125491 ) ) ;
#167327=DIRECTION ( 'NONE',  ( 0.000000000000000000, 0.000000000000000000, -1.000000000000000000 ) ) ;
#167331=DIRECTION ( 'NONE',  ( -1.000000000000000000, -3.265361837132813093E-16, 0.000000000000000000 ) ) ;
#167333=CARTESIAN_POINT ( 'NONE',  ( -20.94999999999999929, -11.48912529307605901, -3.100000000000000533 ) ) ;
#167356=DIRECTION ( 'NONE',  ( 0.000000000000000000, 0.000000000000000000, -1.000000000000000000 ) ) ;
#167357=FACE_OUTER_BOUND ( 'NONE', #127395, .T. ) ;
#167365=CARTESIAN_POINT ( 'NONE',  ( 21.05000000000000071, 11.75000000000000355, -26.65839931010293995 ) ) ;
#167379=DIRECTION ( 'NONE',  ( 0.000000000000000000, 0.000000000000000000, -1.000000000000000000 ) ) ;
#167401=CARTESIAN_POINT ( 'NONE',  ( -23.15000000000000213, 0.000000000000000000, 0.000000000000000000 ) ) ;
#167418=VERTEX_POINT ( 'NONE', #217290 ) ;
#167432=CARTESIAN_POINT ( 'NONE',  ( 22.39999999999999503, -0.1008583690987139431, 11.74956712348939192 ) ) ;
#167456=AXIS2_PLACEMENT_3D ( 'NONE', #128987, #111997, #188955 ) ;
#167474=CIRCLE ( 'NONE', #201332, 0.09999999999999939493 ) ;
#167515=( BOUNDED_SURFACE ( )  B_SPLINE_SURFACE ( 3, 2, ( 
 ( #49474, #186432, #7791 ),
 ( #69059, #45631, #106865 ),
 ( #148584, #26074, #207284 ),
 ( #129023, #28679, #87300 ) ),
 .UNSPECIFIED., .F., .F., .F. ) 
 B_SPLINE_SURFACE_WITH_KNOTS ( ( 4, 4 ),
 ( 3, 3 ),
 ( 0.0006461284895273937097, 0.0007503702773986277094 ),
 ( 0.000000000000000000, 1.000000000000000000 ),
 .UNSPECIFIED. ) 
 GEOMETRIC_REPRESENTATION_ITEM ( )  RATIONAL_B_SPLINE_SURFACE ( (
 ( 1.000000000000000000, 0.7071067811865475727, 1.000000000000000000),
 ( 1.000000000000000000, 0.7076476444648727160, 1.000000000000000000),
 ( 1.000000000000000000, 0.7075727925191928058, 1.000000000000000000),
 ( 1.000000000000000000, 0.7071067811865471286, 1.000000000000000000) ) ) 
 REPRESENTATION_ITEM ( '' )  SURFACE ( )  );
#167563=FACE_OUTER_BOUND ( 'NONE', #7081, .T. ) ;
#167564=EDGE_LOOP ( 'NONE', ( #6224, #23898, #192099, #70118 ) ) ;
#167566=ORIENTED_EDGE ( 'NONE', *, *, #74192, .F. ) ;
#167576=AXIS2_PLACEMENT_3D ( 'NONE', #166149, #245648, #22768 ) ;
#167588=CARTESIAN_POINT ( 'NONE',  ( 23.14999999999999503, 6.649999999999999467, -12.15000000000000036 ) ) ;
#167596=ORIENTED_EDGE ( 'NONE', *, *, #29137, .T. ) ;
#167639=EDGE_LOOP ( 'NONE', ( #163965, #40384, #111165, #132429, #246775, #58535, #43937, #14476, #29711, #158177, #27718 ) ) ;
#167652=ORIENTED_EDGE ( 'NONE', *, *, #235089, .F. ) ;
#167710=CARTESIAN_POINT ( 'NONE',  ( 23.15000000000000213, -11.48912529307605546, -30.39999999999999503 ) ) ;
#167717=DIRECTION ( 'NONE',  ( 0.000000000000000000, -1.000000000000000000, 0.000000000000000000 ) ) ;
#167737=EDGE_CURVE ( 'NONE', #256663, #43421, #126181, .T. ) ;
#167746=EDGE_CURVE ( 'NONE', #3631, #172600, #253551, .T. ) ;
#167760=DIRECTION ( 'NONE',  ( -1.000000000000000000, 0.000000000000000000, 0.000000000000000000 ) ) ;
#167763=DIRECTION ( 'NONE',  ( 1.000000000000000000, 0.000000000000000000, 0.000000000000000000 ) ) ;
#167766=ORIENTED_EDGE ( 'NONE', *, *, #72597, .T. ) ;
#167773=VERTEX_POINT ( 'NONE', #207415 ) ;
#167844=DIRECTION ( 'NONE',  ( -0.7071067811865475727, -0.7071067811865475727, -0.000000000000000000 ) ) ;
#167868=CARTESIAN_POINT ( 'NONE',  ( 20.94999999999999929, -1.162701749938009677, -7.900000000000000355 ) ) ;
#167870=ORIENTED_EDGE ( 'NONE', *, *, #200286, .T. ) ;
#167888=AXIS2_PLACEMENT_3D ( 'NONE', #33027, #72117, #168687 ) ;
#167893=VERTEX_POINT ( 'NONE', #252930 ) ;
#167899=CARTESIAN_POINT ( 'NONE',  ( 23.14999999999999503, 6.649999999999999467, -21.25000000000000000 ) ) ;
#167921=CYLINDRICAL_SURFACE ( 'NONE', #118989, 0.09999999999999939493 ) ;
#167922=DIRECTION ( 'NONE',  ( 1.000000000000000000, 0.000000000000000000, 0.000000000000000000 ) ) ;
#167931=TOROIDAL_SURFACE ( 'NONE', #130295, 11.70000000000000107, 0.1000000000000000056 ) ;
#167968=ORIENTED_EDGE ( 'NONE', *, *, #205494, .T. ) ;
#167987=ORIENTED_EDGE ( 'NONE', *, *, #181744, .T. ) ;
#167995=CARTESIAN_POINT ( 'NONE',  ( 23.24999999999999289, 6.649999999999999467, -12.15000000000000036 ) ) ;
#168051=TOROIDAL_SURFACE ( 'NONE', #226218, 11.65000000000000036, 0.1000000000000000056 ) ;
#168059=AXIS2_PLACEMENT_3D ( 'NONE', #97424, #180858, #177030 ) ;
#168079=CARTESIAN_POINT ( 'NONE',  ( 20.94999999999999929, 8.876614585087098774, -8.385080478844676222 ) ) ;
#168090=CARTESIAN_POINT ( 'NONE',  ( -18.43459694179558639, -9.494210124998035738, -40.11700520266107617 ) ) ;
#168114=VERTEX_POINT ( 'NONE', #118589 ) ;
#168122=DIRECTION ( 'NONE',  ( -0.7071067811865388020, 0.7071067811865561215, 0.000000000000000000 ) ) ;
#168130=DIRECTION ( 'NONE',  ( 1.000000000000000000, 0.000000000000000000, 0.000000000000000000 ) ) ;
#168131=VERTEX_POINT ( 'NONE', #83260 ) ;
#168180=DIRECTION ( 'NONE',  ( 0.000000000000000000, 0.000000000000000000, -1.000000000000000000 ) ) ;
#168183=CARTESIAN_POINT ( 'NONE',  ( -18.59999999999999787, 9.150000000000002132, -21.15000000000000213 ) ) ;
#168190=ORIENTED_EDGE ( 'NONE', *, *, #142834, .T. ) ;
#168216=ORIENTED_EDGE ( 'NONE', *, *, #250511, .T. ) ;
#168256=CARTESIAN_POINT ( 'NONE',  ( 20.94999999999999929, -11.64999999999999147, -33.49999999999998579 ) ) ;
#168278=ORIENTED_EDGE ( 'NONE', *, *, #184921, .T. ) ;
#168279=DIRECTION ( 'NONE',  ( 0.000000000000000000, 0.000000000000000000, -1.000000000000000000 ) ) ;
#168281=ORIENTED_EDGE ( 'NONE', *, *, #134483, .F. ) ;
#168325=LINE ( 'NONE', #232119, #119598 ) ;
#168333=CARTESIAN_POINT ( 'NONE',  ( -20.94999999999999929, 14.05000000000000071, -5.513695070760990191 ) ) ;
#168338=FACE_OUTER_BOUND ( 'NONE', #8573, .T. ) ;
#168347=ADVANCED_FACE ( 'NONE', ( #222783 ), #155071, .F. ) ;
#168358=DIRECTION ( 'NONE',  ( 1.000000000000000000, 0.000000000000000000, 0.000000000000000000 ) ) ;
#168359=AXIS2_PLACEMENT_3D ( 'NONE', #37342, #191295, #252502 ) ;
#168387=AXIS2_PLACEMENT_3D ( 'NONE', #67, #163026, #159182 ) ;
#168390=AXIS2_PLACEMENT_3D ( 'NONE', #245390, #105839, #181573 ) ;
#168391=AXIS2_PLACEMENT_3D ( 'NONE', #123457, #163873, #166465 ) ;
#168437=CARTESIAN_POINT ( 'NONE',  ( 19.97071067811864609, 11.72071067811865674, -24.65000000000000213 ) ) ;
#168469=AXIS2_PLACEMENT_3D ( 'NONE', #94064, #236154, #172381 ) ;
#168496=LINE ( 'NONE', #111039, #115331 ) ;
#168519=ORIENTED_EDGE ( 'NONE', *, *, #131049, .F. ) ;
#168520=( GEOMETRIC_REPRESENTATION_CONTEXT ( 3 ) GLOBAL_UNCERTAINTY_ASSIGNED_CONTEXT ( ( #29565 ) ) GLOBAL_UNIT_ASSIGNED_CONTEXT ( ( #3045, #102129, #137422 ) ) REPRESENTATION_CONTEXT ( 'NONE', 'WORKASPACE' ) );
#168530=ORIENTED_EDGE ( 'NONE', *, *, #227717, .T. ) ;
#168540=AXIS2_PLACEMENT_3D ( 'NONE', #227131, #207599, #9366 ) ;
#168547=DIRECTION ( 'NONE',  ( 1.000000000000000000, 0.000000000000000000, 0.000000000000000000 ) ) ;
#168548=CYLINDRICAL_SURFACE ( 'NONE', #90788, 0.09999999999999939493 ) ;
#168570=ORIENTED_EDGE ( 'NONE', *, *, #125824, .T. ) ;
#168578=CARTESIAN_POINT ( 'NONE',  ( -23.25000000000000000, -1.851617760468904805, -45.10318971960366241 ) ) ;
#168604=AXIS2_PLACEMENT_3D ( 'NONE', #193484, #233879, #72247 ) ;
#168625=DIRECTION ( 'NONE',  ( 1.000000000000000000, -7.304098846218134667E-16, 0.000000000000000000 ) ) ;
#168659=SHAPE_REPRESENTATION ( 'Injection Molded Chain Links', ( #2425 ), #114299 ) ;
#168661=ADVANCED_FACE ( 'NONE', ( #107673 ), #146780, .T. ) ;
#168687=DIRECTION ( 'NONE',  ( 0.000000000000000000, -1.000000000000000000, 0.000000000000000000 ) ) ;
#168688=LINE ( 'NONE', #129513, #232747 ) ;
#168698=CARTESIAN_POINT ( 'NONE',  ( -22.39999999999999858, 11.75000000000000000, -0.1000000000000028644 ) ) ;
#168735=B_SPLINE_CURVE_WITH_KNOTS ( 'NONE', 3,
 ( #57668, #18568, #82350, #198478, #100627, #77235, #180219, #161946 ),
 .UNSPECIFIED., .F., .F.,
 ( 4, 2, 2, 4 ),
 ( 0.000000000000000000, 0.0001094981963948484779, 0.0002189963927896969558, 0.0004379927855793939117 ),
 .UNSPECIFIED. ) ;
#168745=DIRECTION ( 'NONE',  ( 0.000000000000000000, 0.000000000000000000, 1.000000000000000000 ) ) ;
#168803=DIRECTION ( 'NONE',  ( 1.000000000000000000, 0.000000000000000000, 0.000000000000000000 ) ) ;
#168822=ORIENTED_EDGE ( 'NONE', *, *, #172679, .F. ) ;
#168829=EDGE_CURVE ( 'NONE', #140958, #41654, #210630, .T. ) ;
#168835=ORIENTED_EDGE ( 'NONE', *, *, #9684, .F. ) ;
#168879=AXIS2_PLACEMENT_3D ( 'NONE', #242388, #57643, #162890 ) ;
#168882=DIRECTION ( 'NONE',  ( 1.000000000000000000, 3.265361837132813093E-16, -0.000000000000000000 ) ) ;
#168892=CARTESIAN_POINT ( 'NONE',  ( 22.60000000000000142, 11.74956712348939192, 0.1008583690987087389 ) ) ;
#168911=DIRECTION ( 'NONE',  ( 1.000000000000000000, 0.000000000000000000, 0.000000000000000000 ) ) ;
#168933=DIRECTION ( 'NONE',  ( -0.7071067811865474617, -0.7071067811865474617, -0.000000000000000000 ) ) ;
#168954=ORIENTED_EDGE ( 'NONE', *, *, #116270, .F. ) ;
#168961=DIRECTION ( 'NONE',  ( 0.000000000000000000, -1.000000000000000000, 6.308085367188393199E-16 ) ) ;
#168993=FACE_OUTER_BOUND ( 'NONE', #176554, .T. ) ;
#169002=EDGE_CURVE ( 'NONE', #147671, #17816, #138618, .T. ) ;
#169008=DIRECTION ( 'NONE',  ( -0.1538461538461510236, 0.9880948137434718559, 0.000000000000000000 ) ) ;
#169013=ORIENTED_EDGE ( 'NONE', *, *, #199764, .T. ) ;
#169025=CIRCLE ( 'NONE', #48176, 0.09999999999999939493 ) ;
#169035=VECTOR ( 'NONE', #207805, 1000.000000000000000 ) ;
#169042=CARTESIAN_POINT ( 'NONE',  ( -22.50000000000000000, 11.64976291803192154, 0.08880997638692984808 ) ) ;
#169096=VERTEX_POINT ( 'NONE', #140582 ) ;
#169150=ORIENTED_EDGE ( 'NONE', *, *, #211954, .T. ) ;
#169152=ORIENTED_EDGE ( 'NONE', *, *, #140332, .T. ) ;
#169165=EDGE_CURVE ( 'NONE', #144794, #58858, #145619, .T. ) ;
#169172=AXIS2_PLACEMENT_3D ( 'NONE', #126711, #212677, #253064 ) ;
#169215=EDGE_CURVE ( 'NONE', #160332, #158841, #104005, .T. ) ;
#169224=CARTESIAN_POINT ( 'NONE',  ( 23.24999999999999645, 0.000000000000000000, 0.000000000000000000 ) ) ;
#169227=DIRECTION ( 'NONE',  ( 1.000000000000000000, -0.000000000000000000, -0.000000000000000000 ) ) ;
#169267=CARTESIAN_POINT ( 'NONE',  ( 20.94999999999999929, 4.999999999999997335, -21.09473398108690390 ) ) ;
#169273=CARTESIAN_POINT ( 'NONE',  ( 21.12802099929860944, 8.780552590222212572, -12.24818998493161892 ) ) ;
#169298=CYLINDRICAL_SURFACE ( 'NONE', #140451, 0.1000000000000002554 ) ;
#169308=EDGE_CURVE ( 'NONE', #191070, #115218, #88935, .T. ) ;
#169331=DIRECTION ( 'NONE',  ( -0.000000000000000000, 0.1350103645451876666, 0.9908441862701600211 ) ) ;
#169349=ORIENTED_EDGE ( 'NONE', *, *, #85126, .T. ) ;
#169351=TOROIDAL_SURFACE ( 'NONE', #256743, 3.899999999999999467, 0.1000000000000000056 ) ;
#169352=ORIENTED_EDGE ( 'NONE', *, *, #86375, .F. ) ;
#169357=DIRECTION ( 'NONE',  ( 0.000000000000000000, 0.000000000000000000, -1.000000000000000000 ) ) ;
#169368=AXIS2_PLACEMENT_3D ( 'NONE', #244283, #173809, #212883 ) ;
#169373=CARTESIAN_POINT ( 'NONE',  ( -18.40000000000000213, -9.682403433476402199, -40.15684337741277687 ) ) ;
#169378=LINE ( 'NONE', #203330, #118630 ) ;
#169389=TOROIDAL_SURFACE ( 'NONE', #86104, 0.4000000000000009104, 0.1000000000000000056 ) ;
#169395=EDGE_CURVE ( 'NONE', #74587, #113723, #5540, .T. ) ;
#169464=DIRECTION ( 'NONE',  ( 0.000000000000000000, 0.000000000000000000, -1.000000000000000000 ) ) ;
#169470=VERTEX_POINT ( 'NONE', #71348 ) ;
#169503=EDGE_CURVE ( 'NONE', #113723, #94186, #22345, .T. ) ;
#169519=DIRECTION ( 'NONE',  ( 0.000000000000000000, 0.000000000000000000, -1.000000000000000000 ) ) ;
#169542=VERTEX_POINT ( 'NONE', #217232 ) ;
#169558=AXIS2_PLACEMENT_3D ( 'NONE', #110205, #128502, #50224 ) ;
#169568=ORIENTED_EDGE ( 'NONE', *, *, #180986, .F. ) ;
#169582=VECTOR ( 'NONE', #211635, 1000.000000000000000 ) ;
#169595=ORIENTED_EDGE ( 'NONE', *, *, #110945, .F. ) ;
#169596=FACE_OUTER_BOUND ( 'NONE', #173287, .T. ) ;
#169603=VECTOR ( 'NONE', #32946, 1000.000000000000000 ) ;
#169614=CARTESIAN_POINT ( 'NONE',  ( -21.11825140030074621, 6.445407565420032014, 0.007203620632664132876 ) ) ;
#169625=VECTOR ( 'NONE', #214599, 1000.000000000000000 ) ;
#169661=CIRCLE ( 'NONE', #82277, 0.1000000000000000472 ) ;
#169694=ORIENTED_EDGE ( 'NONE', *, *, #65832, .F. ) ;
#169699=EDGE_CURVE ( 'NONE', #197777, #90989, #84822, .T. ) ;
#169700=ORIENTED_EDGE ( 'NONE', *, *, #37427, .T. ) ;
#169707=CARTESIAN_POINT ( 'NONE',  ( -20.00857864376270001, 9.250000000000001776, -21.15000000000000213 ) ) ;
#169782=DIRECTION ( 'NONE',  ( 0.000000000000000000, 0.000000000000000000, -1.000000000000000000 ) ) ;
#169811=ADVANCED_FACE ( 'NONE', ( #11048 ), #248377, .F. ) ;
#169812=DIRECTION ( 'NONE',  ( 0.000000000000000000, -0.000000000000000000, 1.000000000000000000 ) ) ;
#169831=EDGE_LOOP ( 'NONE', ( #226476, #169150, #160456, #151510 ) ) ;
#169875=DIRECTION ( 'NONE',  ( 0.000000000000000000, 0.000000000000000000, -1.000000000000000000 ) ) ;
#169903=ORIENTED_EDGE ( 'NONE', *, *, #88156, .T. ) ;
#169914=LINE ( 'NONE', #224683, #204087 ) ;
#169917=CYLINDRICAL_SURFACE ( 'NONE', #198515, 0.09999999999999939493 ) ;
#169919=CARTESIAN_POINT ( 'NONE',  ( 20.94999999999999929, 0.000000000000000000, -33.50000000000000000 ) ) ;
#169927=DIRECTION ( 'NONE',  ( 0.000000000000000000, 0.000000000000000000, -1.000000000000000000 ) ) ;
#169932=EDGE_CURVE ( 'NONE', #27728, #122573, #147402, .T. ) ;
#169952=CARTESIAN_POINT ( 'NONE',  ( 23.24999999999999289, 11.65000000000000746, -21.35000000000000142 ) ) ;
#169964=CIRCLE ( 'NONE', #178317, 0.09999999999999939493 ) ;
#169965=AXIS2_PLACEMENT_3D ( 'NONE', #110620, #152349, #14110 ) ;
#170014=CIRCLE ( 'NONE', #136618, 0.1000000000000028644 ) ;
#170064=AXIS2_PLACEMENT_3D ( 'NONE', #249449, #209025, #51198 ) ;
#170075=LINE ( 'NONE', #146581, #257351 ) ;
#170111=VERTEX_POINT ( 'NONE', #60431 ) ;
#170139=VECTOR ( 'NONE', #179521, 1000.000000000000000 ) ;
#170166=AXIS2_PLACEMENT_3D ( 'NONE', #32409, #12836, #110626 ) ;
#170167=CARTESIAN_POINT ( 'NONE',  ( 18.49999999999999289, 11.65000000000000391, 11.75000000000000000 ) ) ;
#170175=DIRECTION ( 'NONE',  ( 1.000000000000000000, -0.000000000000000000, -0.000000000000000000 ) ) ;
#170200=ORIENTED_EDGE ( 'NONE', *, *, #105721, .F. ) ;
#170221=AXIS2_PLACEMENT_3D ( 'NONE', #245588, #86472, #202602 ) ;
#170232=LINE ( 'NONE', #150617, #97616 ) ;
#170279=CARTESIAN_POINT ( 'NONE',  ( -23.25000000000000000, -1.835859311443637010, -45.00443916879852679 ) ) ;
#170293=DIRECTION ( 'NONE',  ( -3.265361837132813093E-16, 1.000000000000000000, 0.000000000000000000 ) ) ;
#170296=DIRECTION ( 'NONE',  ( 0.000000000000000000, 0.000000000000000000, 1.000000000000000000 ) ) ;
#170298=CARTESIAN_POINT ( 'NONE',  ( 21.08804582317332077, 8.878166167091915639, -12.34999982940562191 ) ) ;
#170299=LINE ( 'NONE', #231522, #180170 ) ;
#170305=CIRCLE ( 'NONE', #99309, 2.000000000000002665 ) ;
#170323=CARTESIAN_POINT ( 'NONE',  ( 22.42357213249528769, 7.672932386359915924, 0.09908696400155941886 ) ) ;
#170327=VECTOR ( 'NONE', #212653, 1000.000000000000114 ) ;
#170328=CARTESIAN_POINT ( 'NONE',  ( 21.05000000000000071, 5.399999999999998579, -12.40526601891309788 ) ) ;
#170350=LINE ( 'NONE', #249838, #78923 ) ;
#170368=AXIS2_PLACEMENT_3D ( 'NONE', #63688, #102795, #4976 ) ;
#170371=ORIENTED_EDGE ( 'NONE', *, *, #177704, .T. ) ;
#170397=EDGE_CURVE ( 'NONE', #16494, #213315, #72788, .T. ) ;
#170418=CARTESIAN_POINT ( 'NONE',  ( 20.94999999999999929, 10.72371710470752504, -12.15000000000000036 ) ) ;
#170462=ORIENTED_EDGE ( 'NONE', *, *, #119533, .T. ) ;
#170470=CARTESIAN_POINT ( 'NONE',  ( 18.59999999999999432, 1.728086936794463346, 13.11556499483223348 ) ) ;
#170474=AXIS2_PLACEMENT_3D ( 'NONE', #73658, #180132, #1470 ) ;
#170492=LINE ( 'NONE', #150868, #146094 ) ;
#170516=VERTEX_POINT ( 'NONE', #242623 ) ;
#170529=DIRECTION ( 'NONE',  ( 2.715809747126116508E-16, -1.000000000000000000, 0.000000000000000000 ) ) ;
#170549=CARTESIAN_POINT ( 'NONE',  ( 20.95429402530546170, 8.876194151102188457, -8.523086697937838352 ) ) ;
#170552=CARTESIAN_POINT ( 'NONE',  ( -21.05000000000000071, 0.000000000000000000, -21.69999999999999929 ) ) ;
#170591=FACE_OUTER_BOUND ( 'NONE', #128111, .T. ) ;
#170595=DIRECTION ( 'NONE',  ( 1.000000000000000000, -0.000000000000000000, -0.000000000000000000 ) ) ;
#170600=DIRECTION ( 'NONE',  ( 0.000000000000000000, 0.000000000000000000, -1.000000000000000000 ) ) ;
#170612=CARTESIAN_POINT ( 'NONE',  ( 21.12400247839510214, 10.72148804403030198, -12.25000000000000178 ) ) ;
#170667=CARTESIAN_POINT ( 'NONE',  ( -18.44204374631835819, -9.491036389598342282, -40.12620127022106686 ) ) ;
#170673=CARTESIAN_POINT ( 'NONE',  ( 18.59999999999999787, 1.851028230140860487, -11.65391326942249250 ) ) ;
#170691=DIRECTION ( 'NONE',  ( 1.000000000000000000, 0.000000000000000000, 0.000000000000000000 ) ) ;
#170705=ADVANCED_FACE ( 'NONE', ( #195202 ), #58204, .F. ) ;
#170767=DIRECTION ( 'NONE',  ( 1.000000000000000000, 0.000000000000000000, 0.000000000000000000 ) ) ;
#170820=ORIENTED_EDGE ( 'NONE', *, *, #143512, .F. ) ;
#170822=TOROIDAL_SURFACE ( 'NONE', #129079, 0.2000000000000000111, 0.1000000000000000056 ) ;
#170824=DIRECTION ( 'NONE',  ( -1.000000000000000000, 0.000000000000000000, 0.000000000000000000 ) ) ;
#170846=AXIS2_PLACEMENT_3D ( 'NONE', #149161, #128305, #29237 ) ;
#170867=CARTESIAN_POINT ( 'NONE',  ( -18.50000000000000000, 0.000000000000000000, 0.000000000000000000 ) ) ;
#170881=CARTESIAN_POINT ( 'NONE',  ( -21.05000000000000071, 14.05000000000000071, -5.513695070760990191 ) ) ;
#170911=CARTESIAN_POINT ( 'NONE',  ( -18.41353343127311959, -9.500000000000005329, -7.032069396699669461 ) ) ;
#170934=CIRCLE ( 'NONE', #187457, 0.09999999999999982514 ) ;
#171026=VECTOR ( 'NONE', #116140, 1000.000000000000000 ) ;
#171103=EDGE_CURVE ( 'NONE', #65265, #241989, #156352, .T. ) ;
#171149=SPHERICAL_SURFACE ( 'NONE', #229202, 0.1000000000000000056 ) ;
#171201=DIRECTION ( 'NONE',  ( -1.000000000000000000, -0.000000000000000000, -0.000000000000000000 ) ) ;
#171271=LINE ( 'NONE', #128247, #169035 ) ;
#171274=ORIENTED_EDGE ( 'NONE', *, *, #80279, .F. ) ;
#171276=CARTESIAN_POINT ( 'NONE',  ( 18.39999999999999858, -9.600000000000003197, -40.10018939122204529 ) ) ;
#171322=EDGE_CURVE ( 'NONE', #134956, #136601, #210667, .T. ) ;
#171334=DIRECTION ( 'NONE',  ( 0.000000000000000000, -0.8660254037844384856, 0.5000000000000003331 ) ) ;
#171343=AXIS2_PLACEMENT_3D ( 'NONE', #57932, #220866, #119223 ) ;
#171346=CARTESIAN_POINT ( 'NONE',  ( -20.94999999999999929, 1.835341550224413698, -11.55515129256298046 ) ) ;
#171359=ORIENTED_EDGE ( 'NONE', *, *, #144500, .F. ) ;
#171368=LINE ( 'NONE', #189609, #53188 ) ;
#171382=ORIENTED_EDGE ( 'NONE', *, *, #77192, .T. ) ;
#171385=ORIENTED_EDGE ( 'NONE', *, *, #17947, .F. ) ;
#171399=LINE ( 'NONE', #210491, #22344 ) ;
#171408=CARTESIAN_POINT ( 'NONE',  ( 20.46382478191414833, 10.59862044129738123, -7.677814469345459969 ) ) ;
#171425=CARTESIAN_POINT ( 'NONE',  ( 23.24999999999999289, 6.649999999999999467, -21.15000000000000213 ) ) ;
#171457=ADVANCED_FACE ( 'NONE', ( #246819 ), #49907, .F. ) ;
#171470=( NAMED_UNIT ( * ) SI_UNIT ( $, .STERADIAN. ) SOLID_ANGLE_UNIT ( ) );
#171522=DIRECTION ( 'NONE',  ( 1.000000000000000000, -7.304098846218133681E-16, 4.217023435051677994E-16 ) ) ;
#171532=ADVANCED_FACE ( 'NONE', ( #197118 ), #176309, .T. ) ;
#171547=EDGE_LOOP ( 'NONE', ( #75004, #239073, #216499, #105479 ) ) ;
#171595=FACE_OUTER_BOUND ( 'NONE', #91694, .T. ) ;
#171601=ORIENTED_EDGE ( 'NONE', *, *, #226737, .T. ) ;
#171603=CARTESIAN_POINT ( 'NONE',  ( 20.95595624212412389, 10.62389120309414992, -7.629632914126892373 ) ) ;
#171605=SPHERICAL_SURFACE ( 'NONE', #194816, 0.1000000000000000056 ) ;
#171659=DIRECTION ( 'NONE',  ( 0.000000000000000000, 0.000000000000000000, 1.000000000000000000 ) ) ;
#171676=FACE_OUTER_BOUND ( 'NONE', #42398, .T. ) ;
#171693=DIRECTION ( 'NONE',  ( 2.952720810173289112E-16, -1.000000000000000000, -0.000000000000000000 ) ) ;
#171707=CARTESIAN_POINT ( 'NONE',  ( -20.54999999999999716, 2.399999999999999467, -20.27537807723789953 ) ) ;
#171717=VERTEX_POINT ( 'NONE', #107004 ) ;
#171732=LINE ( 'NONE', #152164, #247734 ) ;
#171742=EDGE_CURVE ( 'NONE', #193752, #251409, #108312, .T. ) ;
#171745=DIRECTION ( 'NONE',  ( -1.000000000000000000, 0.000000000000000000, 0.000000000000000000 ) ) ;
#171768=ORIENTED_EDGE ( 'NONE', *, *, #142886, .T. ) ;
#171812=CIRCLE ( 'NONE', #142530, 0.5000000000000004441 ) ;
#171827=AXIS2_PLACEMENT_3D ( 'NONE', #91746, #171334, #145931 ) ;
#171834=CARTESIAN_POINT ( 'NONE',  ( -20.85000000000000142, -1.164121893241208960, -41.21484808557161017 ) ) ;
#171867=LINE ( 'NONE', #130122, #9240 ) ;
#171874=LINE ( 'NONE', #250093, #119829 ) ;
#171877=CARTESIAN_POINT ( 'NONE',  ( 21.04116576186320486, 10.62466307875135563, -12.32858176862772126 ) ) ;
#171926=AXIS2_PLACEMENT_3D ( 'NONE', #154299, #233796, #2856 ) ;
#171953=ADVANCED_FACE ( 'NONE', ( #116024 ), #169389, .F. ) ;
#171963=VECTOR ( 'NONE', #38421, 1000.000000000000000 ) ;
#171982=DIRECTION ( 'NONE',  ( -1.000000000000000000, 0.000000000000000000, 0.000000000000000000 ) ) ;
#171985=CARTESIAN_POINT ( 'NONE',  ( 18.41789779300683705, -9.500000000000000000, -7.032069666360214022 ) ) ;
#172005=CIRCLE ( 'NONE', #213652, 0.9750000000000036415 ) ;
#172013=FACE_OUTER_BOUND ( 'NONE', #3789, .T. ) ;
#172031=CARTESIAN_POINT ( 'NONE',  ( -21.05000000000000071, -1.261786168565025568, -8.086498963545480478 ) ) ;
#172032=ORIENTED_EDGE ( 'NONE', *, *, #257492, .F. ) ;
#172037=FACE_OUTER_BOUND ( 'NONE', #185709, .T. ) ;
#172071=DIRECTION ( 'NONE',  ( -1.000000000000000000, 0.000000000000000000, 0.000000000000000000 ) ) ;
#172101=ORIENTED_EDGE ( 'NONE', *, *, #141432, .T. ) ;
#172103=CYLINDRICAL_SURFACE ( 'NONE', #26011, 0.09999999999999892308 ) ;
#172104=CARTESIAN_POINT ( 'NONE',  ( -20.64999999999999858, 1.925233644859811521, -20.76975646687386501 ) ) ;
#172116=EDGE_CURVE ( 'NONE', #38660, #209135, #81813, .T. ) ;
#172121=ORIENTED_EDGE ( 'NONE', *, *, #218099, .T. ) ;
#172162=LINE ( 'NONE', #213809, #91823 ) ;
#172182=DIRECTION ( 'NONE',  ( -1.000000000000000000, 0.000000000000000000, 0.000000000000000000 ) ) ;
#172188=CARTESIAN_POINT ( 'NONE',  ( -22.45372860728439690, 0.01492061954848863947, 11.64979713470387424 ) ) ;
#172189=CARTESIAN_POINT ( 'NONE',  ( -20.85000000000000142, 0.000000000000000000, -33.50000000000000000 ) ) ;
#172202=AXIS2_PLACEMENT_3D ( 'NONE', #42616, #86854, #146832 ) ;
#172203=CARTESIAN_POINT ( 'NONE',  ( -22.50000000000000000, 0.000000000000000000, 0.000000000000000000 ) ) ;
#172204=EDGE_CURVE ( 'NONE', #90335, #113100, #85023, .T. ) ;
#172210=AXIS2_PLACEMENT_3D ( 'NONE', #137968, #197950, #3602 ) ;
#172227=CARTESIAN_POINT ( 'NONE',  ( -21.05000000000000071, -11.48912529307605546, -30.39999999999999503 ) ) ;
#172229=DIRECTION ( 'NONE',  ( 0.000000000000000000, 0.000000000000000000, -1.000000000000000000 ) ) ;
#172236=CARTESIAN_POINT ( 'NONE',  ( -20.94999999999999929, 4.898587196589411843E-16, -37.50000000000000000 ) ) ;
#172248=CARTESIAN_POINT ( 'NONE',  ( -22.50000000000000000, 0.000000000000000000, 6.249999999999998224 ) ) ;
#172273=CIRCLE ( 'NONE', #126235, 0.1999999999999996503 ) ;
#172326=CARTESIAN_POINT ( 'NONE',  ( 20.94999999999999574, 1.249999999999999334, -8.000000000000000000 ) ) ;
#172327=CARTESIAN_POINT ( 'NONE',  ( -21.64999999999999858, 7.249999999999992895, -21.25000000000000000 ) ) ;
#172348=DIRECTION ( 'NONE',  ( 0.000000000000000000, -0.1350103645451876944, 0.9908441862701601321 ) ) ;
#172362=DIRECTION ( 'NONE',  ( 1.000000000000000000, 0.000000000000000000, 0.000000000000000000 ) ) ;
#172376=EDGE_CURVE ( 'NONE', #44715, #221017, #136522, .T. ) ;
#172381=DIRECTION ( 'NONE',  ( 0.000000000000000000, 0.000000000000000000, 1.000000000000000000 ) ) ;
#172386=VERTEX_POINT ( 'NONE', #14048 ) ;
#172417=EDGE_LOOP ( 'NONE', ( #102168, #195300, #587, #115904 ) ) ;
#172422=ADVANCED_FACE ( 'NONE', ( #114417 ), #156140, .T. ) ;
#172423=DIRECTION ( 'NONE',  ( -2.952720810173288619E-16, 1.000000000000000000, 0.000000000000000000 ) ) ;
#172444=CARTESIAN_POINT ( 'NONE',  ( -23.25000000000000000, -1.835859311443637010, -45.00443916879852679 ) ) ;
#172521=CIRCLE ( 'NONE', #14269, 0.1999999999999987899 ) ;
#172540=ORIENTED_EDGE ( 'NONE', *, *, #160963, .F. ) ;
#172553=DIRECTION ( 'NONE',  ( 1.000000000000000000, 1.875376730785737719E-16, 0.000000000000000000 ) ) ;
#172600=VERTEX_POINT ( 'NONE', #190790 ) ;
#172611=DIRECTION ( 'NONE',  ( 0.000000000000000000, -1.000000000000000000, 0.000000000000000000 ) ) ;
#172615=VERTEX_POINT ( 'NONE', #68242 ) ;
#172646=EDGE_CURVE ( 'NONE', #11036, #62328, #185719, .T. ) ;
#172662=AXIS2_PLACEMENT_3D ( 'NONE', #44031, #122287, #81829 ) ;
#172666=AXIS2_PLACEMENT_3D ( 'NONE', #23489, #3889, #224207 ) ;
#172668=DIRECTION ( 'NONE',  ( 0.000000000000000000, 0.000000000000000000, -1.000000000000000000 ) ) ;
#172677=ORIENTED_EDGE ( 'NONE', *, *, #245411, .F. ) ;
#172679=EDGE_CURVE ( 'NONE', #220385, #22057, #160795, .T. ) ;
#172683=ORIENTED_EDGE ( 'NONE', *, *, #243784, .F. ) ;
#172715=CARTESIAN_POINT ( 'NONE',  ( 18.59999999999999076, 6.400000000000003020, -9.930424630061574831 ) ) ;
#172725=FACE_OUTER_BOUND ( 'NONE', #205454, .T. ) ;
#172761=DIRECTION ( 'NONE',  ( -0.000000000000000000, -0.000000000000000000, 1.000000000000000000 ) ) ;
#172783=EDGE_CURVE ( 'NONE', #13860, #146959, #31620, .T. ) ;
#172823=CARTESIAN_POINT ( 'NONE',  ( -22.60000000000080789, 0.04781698046536793367, 11.75002243115275036 ) ) ;
#172841=ORIENTED_EDGE ( 'NONE', *, *, #163327, .T. ) ;
#172894=DIRECTION ( 'NONE',  ( 1.000000000000000000, 0.000000000000000000, 0.000000000000000000 ) ) ;
#172900=CARTESIAN_POINT ( 'NONE',  ( 20.95512820512820085, 10.62384868371188062, -7.664913569087606682 ) ) ;
#172916=CIRCLE ( 'NONE', #77190, 7.900000000000003908 ) ;
#172935=DIRECTION ( 'NONE',  ( 1.000000000000000000, 0.000000000000000000, 0.000000000000000000 ) ) ;
#172936=ADVANCED_FACE ( 'NONE', ( #53436 ), #132989, .F. ) ;
#172953=ORIENTED_EDGE ( 'NONE', *, *, #32660, .F. ) ;
#172955=DIRECTION ( 'NONE',  ( 0.000000000000000000, -1.000000000000000000, 0.000000000000000000 ) ) ;
#172963=EDGE_LOOP ( 'NONE', ( #78508, #70154, #51900, #13275 ) ) ;
#172965=SPHERICAL_SURFACE ( 'NONE', #244016, 0.1000000000000000056 ) ;
#172978=EDGE_CURVE ( 'NONE', #166638, #194720, #136811, .T. ) ;
#172993=VERTEX_POINT ( 'NONE', #22023 ) ;
#172995=VERTEX_POINT ( 'NONE', #160266 ) ;
#173037=EDGE_LOOP ( 'NONE', ( #27796, #82233, #45617, #254941, #177013 ) ) ;
#173081=CARTESIAN_POINT ( 'NONE',  ( -21.55000000000000426, 7.750000000000003553, -21.15000000000000213 ) ) ;
#173090=CARTESIAN_POINT ( 'NONE',  ( -21.98333005346336932, 0.000000000000000000, 7.374075329056680950 ) ) ;
#173092=CYLINDRICAL_SURFACE ( 'NONE', #212528, 0.09999999999999939493 ) ;
#173102=DIRECTION ( 'NONE',  ( -1.000000000000000000, 0.000000000000000000, 0.000000000000000000 ) ) ;
#173124=ORIENTED_EDGE ( 'NONE', *, *, #29263, .T. ) ;
#173149=AXIS2_PLACEMENT_3D ( 'NONE', #160840, #176552, #155718 ) ;
#173166=CYLINDRICAL_SURFACE ( 'NONE', #228884, 0.09999999999999939493 ) ;
#173170=TOROIDAL_SURFACE ( 'NONE', #148163, 0.4000000000000017431, 0.1000000000000000056 ) ;
#173172=ORIENTED_EDGE ( 'NONE', *, *, #78356, .F. ) ;
#173187=DIRECTION ( 'NONE',  ( 1.000000000000000000, 0.000000000000000000, 0.000000000000000000 ) ) ;
#173191=( BOUNDED_SURFACE ( )  B_SPLINE_SURFACE ( 3, 2, ( 
 ( #121796, #20123, #235296 ),
 ( #120525, #38393, #176639 ),
 ( #159627, #37131, #77485 ),
 ( #175365, #39704, #99614 ) ),
 .UNSPECIFIED., .F., .F., .T. ) 
 B_SPLINE_SURFACE_WITH_KNOTS ( ( 4, 4 ),
 ( 3, 3 ),
 ( 0.000000000000000000, 0.001979672783031562362 ),
 ( 0.000000000000000000, 1.000000000000000000 ),
 .UNSPECIFIED. ) 
 GEOMETRIC_REPRESENTATION_ITEM ( )  RATIONAL_B_SPLINE_SURFACE ( (
 ( 1.000000000000000000, 0.7103081912008196719, 1.000000000000000000),
 ( 1.000000000000000000, 0.7104998333558700807, 1.000000000000000000),
 ( 1.000000000000000000, 0.7107238315755209923, 1.000000000000000000),
 ( 1.000000000000000000, 0.7110073749539376209, 1.000000000000000000) ) ) 
 REPRESENTATION_ITEM ( '' )  SURFACE ( )  );
#173229=CARTESIAN_POINT ( 'NONE',  ( -18.49372193242250972, -9.442484523357896009, -40.26478126003478764 ) ) ;
#173281=DIRECTION ( 'NONE',  ( 2.952720810173289112E-16, -1.000000000000000000, -0.000000000000000000 ) ) ;
#173287=EDGE_LOOP ( 'NONE', ( #145482, #240585, #116201, #51310 ) ) ;
#173296=CARTESIAN_POINT ( 'NONE',  ( 18.58725287972291795, -9.566626910691692132, -40.32250480576551865 ) ) ;
#173308=CARTESIAN_POINT ( 'NONE',  ( -20.94999999999999929, 0.000000000000000000, -33.50000000000000000 ) ) ;
#173343=EDGE_CURVE ( 'NONE', #108404, #191917, #48513, .T. ) ;
#173348=DIRECTION ( 'NONE',  ( 0.000000000000000000, 0.000000000000000000, -1.000000000000000000 ) ) ;
#173417=ADVANCED_FACE ( 'NONE', ( #183346 ), #124656, .F. ) ;
#173418=DIRECTION ( 'NONE',  ( -1.000000000000000000, -2.952720810173289112E-16, 0.000000000000000000 ) ) ;
#173465=CARTESIAN_POINT ( 'NONE',  ( 21.05000000000000071, 0.000000000000000000, -12.15000000000000036 ) ) ;
#173480=CARTESIAN_POINT ( 'NONE',  ( -22.44366136229477249, 0.009341569486069218817, 11.64971855747391061 ) ) ;
#173494=EDGE_CURVE ( 'NONE', #212474, #225666, #223649, .T. ) ;
#173528=FACE_OUTER_BOUND ( 'NONE', #53552, .T. ) ;
#173547=CARTESIAN_POINT ( 'NONE',  ( 21.05000000000000071, -11.64999999999999147, -30.59999999999999432 ) ) ;
#173577=ORIENTED_EDGE ( 'NONE', *, *, #180845, .T. ) ;
#173589=CIRCLE ( 'NONE', #73601, 0.9750000000000036415 ) ;
#173605=EDGE_LOOP ( 'NONE', ( #154076, #23168, #49778 ) ) ;
#173611=VECTOR ( 'NONE', #5533, 1000.000000000000000 ) ;
#173622=DIRECTION ( 'NONE',  ( -3.265361837132813093E-16, 1.000000000000000000, 0.000000000000000000 ) ) ;
#173623=FACE_OUTER_BOUND ( 'NONE', #245501, .T. ) ;
#173659=CIRCLE ( 'NONE', #98536, 0.1000000000000001305 ) ;
#173697=ORIENTED_EDGE ( 'NONE', *, *, #131816, .T. ) ;
#173701=ORIENTED_EDGE ( 'NONE', *, *, #256549, .F. ) ;
#173732=CARTESIAN_POINT ( 'NONE',  ( -18.59999999999999787, -1.164121893241208960, -41.41484808557160591 ) ) ;
#173734=FACE_OUTER_BOUND ( 'NONE', #103657, .T. ) ;
#173736=DIRECTION ( 'NONE',  ( 1.000000000000000000, -0.000000000000000000, -0.000000000000000000 ) ) ;
#173754=LINE ( 'NONE', #13345, #44657 ) ;
#173809=DIRECTION ( 'NONE',  ( -1.000000000000000000, -2.952720810173289112E-16, 0.000000000000000000 ) ) ;
#173816=DIRECTION ( 'NONE',  ( 1.000000000000000000, 0.000000000000000000, 0.000000000000000000 ) ) ;
#173821=EDGE_LOOP ( 'NONE', ( #206347, #49897, #25580, #71476 ) ) ;
#173837=CIRCLE ( 'NONE', #248816, 0.1000000000000000611 ) ;
#173889=CARTESIAN_POINT ( 'NONE',  ( 22.59080734064468032, 11.75000000000000000, 0.03074970809707019623 ) ) ;
#173913=DIRECTION ( 'NONE',  ( 0.000000000000000000, 0.000000000000000000, -1.000000000000000000 ) ) ;
#173920=CIRCLE ( 'NONE', #182256, 0.09999999999999939493 ) ;
#173929=DIRECTION ( 'NONE',  ( -0.000000000000000000, -0.000000000000000000, 1.000000000000000000 ) ) ;
#173930=CYLINDRICAL_SURFACE ( 'NONE', #86595, 11.74999999999999645 ) ;
#173945=EDGE_CURVE ( 'NONE', #216320, #158092, #244508, .T. ) ;
#173949=DIRECTION ( 'NONE',  ( 0.000000000000000000, 0.8700118002898322711, -0.4930308989875231140 ) ) ;
#173976=ORIENTED_EDGE ( 'NONE', *, *, #166267, .T. ) ;
#173978=AXIS2_PLACEMENT_3D ( 'NONE', #234140, #157212, #214575 ) ;
#173987=CARTESIAN_POINT ( 'NONE',  ( 20.94999999999999929, 4.813084112149524252, -11.94151775652382419 ) ) ;
#174006=CARTESIAN_POINT ( 'NONE',  ( -18.59999999999999787, 0.000000000000000000, -33.50000000000000000 ) ) ;
#174017=FACE_OUTER_BOUND ( 'NONE', #86535, .T. ) ;
#174023=CARTESIAN_POINT ( 'NONE',  ( -20.54999999999999716, 7.249999999999999112, -12.25000000000000000 ) ) ;
#174024=DIRECTION ( 'NONE',  ( 0.000000000000000000, 1.000000000000000000, 0.000000000000000000 ) ) ;
#174041=LINE ( 'NONE', #230113, #244361 ) ;
#174043=( NAMED_UNIT ( * ) PLANE_ANGLE_UNIT ( ) SI_UNIT ( $, .RADIAN. ) );
#174062=DIRECTION ( 'NONE',  ( -1.000000000000000000, -0.000000000000000000, -0.000000000000000000 ) ) ;
#174081=ORIENTED_EDGE ( 'NONE', *, *, #140754, .T. ) ;
#174109=CARTESIAN_POINT ( 'NONE',  ( -20.85000000000000142, -1.263275465217258198, -41.40186466674640542 ) ) ;
#174143=EDGE_CURVE ( 'NONE', #32549, #62345, #23968, .T. ) ;
#174144=CARTESIAN_POINT ( 'NONE',  ( -20.94999999999999929, 0.000000000000000000, -33.50000000000000000 ) ) ;
#174184=CARTESIAN_POINT ( 'NONE',  ( 21.05000000000000071, 10.42338541491290549, -7.492051923870094221 ) ) ;
#174216=CYLINDRICAL_SURFACE ( 'NONE', #208588, 0.09999999999999982514 ) ;
#174229=VERTEX_POINT ( 'NONE', #210967 ) ;
#174236=VERTEX_POINT ( 'NONE', #32357 ) ;
#174247=DIRECTION ( 'NONE',  ( 0.000000000000000000, 0.000000000000000000, -1.000000000000000000 ) ) ;
#174256=EDGE_CURVE ( 'NONE', #174426, #194720, #171874, .T. ) ;
#174298=ORIENTED_EDGE ( 'NONE', *, *, #257091, .F. ) ;
#174330=AXIS2_PLACEMENT_3D ( 'NONE', #23936, #121746, #83833 ) ;
#174338=CARTESIAN_POINT ( 'NONE',  ( -21.05000000000000071, -11.39257802170566691, -30.42605042016806394 ) ) ;
#174340=DIRECTION ( 'NONE',  ( -0.000000000000000000, -0.1298341882520022694, -0.9915357197604853789 ) ) ;
#174343=CARTESIAN_POINT ( 'NONE',  ( -18.59999999999999787, 1.637172712970381694, -11.58215336547201879 ) ) ;
#174344=VECTOR ( 'NONE', #90579, 999.9999999999998863 ) ;
#174370=CARTESIAN_POINT ( 'NONE',  ( -23.15000000000000213, 0.000000000000000000, -33.50000000000000000 ) ) ;
#174381=ORIENTED_EDGE ( 'NONE', *, *, #219539, .F. ) ;
#174384=AXIS2_PLACEMENT_3D ( 'NONE', #201232, #103399, #199973 ) ;
#174387=CARTESIAN_POINT ( 'NONE',  ( 21.14999999999999503, -0.09999999999999939493, 11.64957080754479968 ) ) ;
#174399=DIRECTION ( 'NONE',  ( 0.000000000000000000, 0.000000000000000000, 1.000000000000000000 ) ) ;
#174426=VERTEX_POINT ( 'NONE', #66000 ) ;
#174434=CIRCLE ( 'NONE', #124311, 11.80000000000000249 ) ;
#174442=ORIENTED_EDGE ( 'NONE', *, *, #17747, .F. ) ;
#174454=CIRCLE ( 'NONE', #61972, 0.1000000000000000472 ) ;
#174461=EDGE_CURVE ( 'NONE', #131148, #103069, #203187, .T. ) ;
#174470=DIRECTION ( 'NONE',  ( 0.000000000000000000, 0.000000000000000000, 1.000000000000000000 ) ) ;
#174475=CIRCLE ( 'NONE', #157898, 0.1000000000000001860 ) ;
#174477=AXIS2_PLACEMENT_3D ( 'NONE', #143551, #186550, #44473 ) ;
#174485=CARTESIAN_POINT ( 'NONE',  ( 18.47149038651511077, -9.671457158006703025, -40.17278633473840443 ) ) ;
#174496=LINE ( 'NONE', #247873, #211946 ) ;
#174531=ORIENTED_EDGE ( 'NONE', *, *, #174143, .T. ) ;
#174537=ORIENTED_EDGE ( 'NONE', *, *, #63148, .T. ) ;
#174560=VERTEX_POINT ( 'NONE', #64715 ) ;
#174567=LINE ( 'NONE', #256550, #126753 ) ;
#174584=CIRCLE ( 'NONE', #49801, 0.09999999999999939493 ) ;
#174589=EDGE_LOOP ( 'NONE', ( #195176, #255118, #252155, #132237 ) ) ;
#174590=DIRECTION ( 'NONE',  ( 1.000000000000000000, 0.000000000000000000, 0.000000000000000000 ) ) ;
#174593=AXIS2_PLACEMENT_3D ( 'NONE', #61051, #143143, #141874 ) ;
#174619=ORIENTED_EDGE ( 'NONE', *, *, #184738, .F. ) ;
#174624=ORIENTED_EDGE ( 'NONE', *, *, #217371, .T. ) ;
#174718=EDGE_CURVE ( 'NONE', #210671, #203969, #36827, .T. ) ;
#174745=DIRECTION ( 'NONE',  ( 0.000000000000000000, 0.000000000000000000, -1.000000000000000000 ) ) ;
#174749=DIRECTION ( 'NONE',  ( 0.000000000000000000, 0.4930308989875230585, 0.8700118002898322711 ) ) ;
#174792=SHAPE_DEFINITION_REPRESENTATION ( #84581, #168659 ) ;
#174817=VECTOR ( 'NONE', #39141, 1000.000000000000000 ) ;
#174827=DIRECTION ( 'NONE',  ( -1.000000000000000000, -1.836970198721029934E-16, 0.000000000000000000 ) ) ;
#174832=AXIS2_PLACEMENT_3D ( 'NONE', #179857, #182424, #59863 ) ;
#174838=FACE_OUTER_BOUND ( 'NONE', #85526, .T. ) ;
#174856=DIRECTION ( 'NONE',  ( -1.000000000000000000, 0.000000000000000000, 0.000000000000000000 ) ) ;
#174858=EDGE_CURVE ( 'NONE', #28425, #106299, #81366, .T. ) ;
#174860=CARTESIAN_POINT ( 'NONE',  ( -23.25000000000000000, 11.65000000000000036, -26.48519422934604961 ) ) ;
#174863=CARTESIAN_POINT ( 'NONE',  ( 23.15000000000000213, -11.48912529307605368, -30.39999999999999503 ) ) ;
#174873=FACE_OUTER_BOUND ( 'NONE', #157037, .T. ) ;
#174906=CARTESIAN_POINT ( 'NONE',  ( 23.25000000000000000, -11.64999999999999147, -30.39999999999999503 ) ) ;
#174923=CARTESIAN_POINT ( 'NONE',  ( 20.95556889135987788, 10.62194358773509606, -7.642394221857522929 ) ) ;
#174936=ADVANCED_FACE ( 'NONE', ( #82649 ), #222167, .F. ) ;
#174940=EDGE_CURVE ( 'NONE', #185056, #231683, #162247, .T. ) ;
#174946=ORIENTED_EDGE ( 'NONE', *, *, #62855, .T. ) ;
#174961=CIRCLE ( 'NONE', #141572, 7.900000000000003908 ) ;
#174993=ORIENTED_EDGE ( 'NONE', *, *, #162712, .F. ) ;
#175006=DIRECTION ( 'NONE',  ( 0.000000000000000000, -0.000000000000000000, 1.000000000000000000 ) ) ;
#175007=DIRECTION ( 'NONE',  ( 1.000000000000000000, 0.000000000000000000, 0.000000000000000000 ) ) ;
#175008=ORIENTED_EDGE ( 'NONE', *, *, #153335, .F. ) ;
#175044=ORIENTED_EDGE ( 'NONE', *, *, #25832, .T. ) ;
#175047=CARTESIAN_POINT ( 'NONE',  ( 18.59999999999999787, 1.866714910057309273, -11.75267524628200633 ) ) ;
#175054=EDGE_LOOP ( 'NONE', ( #239500, #6539, #136905, #10026, #136537, #96352, #152000 ) ) ;
#175066=CARTESIAN_POINT ( 'NONE',  ( 20.94999999999999929, -11.48912529307605546, -30.39999999999999503 ) ) ;
#175069=ORIENTED_EDGE ( 'NONE', *, *, #78623, .F. ) ;
#175116=CIRCLE ( 'NONE', #112532, 0.2000000000000005107 ) ;
#175129=CARTESIAN_POINT ( 'NONE',  ( 22.49999999999999645, 11.64987090376337875, 0.08251989087297323389 ) ) ;
#175139=ADVANCED_FACE ( 'NONE', ( #257113 ), #198472, .T. ) ;
#175144=DIRECTION ( 'NONE',  ( 1.000000000000000000, -0.000000000000000000, -0.000000000000000000 ) ) ;
#175147=EDGE_CURVE ( 'NONE', #62255, #207350, #99351, .T. ) ;
#175198=CYLINDRICAL_SURFACE ( 'NONE', #242636, 0.09999999999999939493 ) ;
#175219=CARTESIAN_POINT ( 'NONE',  ( -21.14999999999999858, 11.65000000000000036, -3.469446951953614189E-15 ) ) ;
#175223=CYLINDRICAL_SURFACE ( 'NONE', #86278, 12.87500000000000000 ) ;
#175243=EDGE_CURVE ( 'NONE', #13199, #55509, #174496, .T. ) ;
#175252=ORIENTED_EDGE ( 'NONE', *, *, #757, .T. ) ;
#175270=AXIS2_PLACEMENT_3D ( 'NONE', #6160, #122279, #141828 ) ;
#175296=CIRCLE ( 'NONE', #162818, 0.1999999999999987899 ) ;
#175297=ADVANCED_FACE ( 'NONE', ( #53205 ), #161896, .T. ) ;
#175309=ORIENTED_EDGE ( 'NONE', *, *, #253639, .T. ) ;
#175316=CIRCLE ( 'NONE', #141967, 11.90000000000000213 ) ;
#175365=CARTESIAN_POINT ( 'NONE',  ( -21.07094088545368749, 0.09889370255222154626, 6.320167221917132316 ) ) ;
#175376=ADVANCED_FACE ( 'NONE', ( #207483, #234398, #28879 ), #114461, .F. ) ;
#175397=DIRECTION ( 'NONE',  ( 1.000000000000000000, -0.000000000000000000, -0.000000000000000000 ) ) ;
#175406=VERTEX_POINT ( 'NONE', #140429 ) ;
#175414=EDGE_LOOP ( 'NONE', ( #101784, #66474, #73757, #211079 ) ) ;
#175467=DIRECTION ( 'NONE',  ( 2.952720810173289112E-16, -1.000000000000000000, 0.000000000000000000 ) ) ;
#175500=ADVANCED_FACE ( 'NONE', ( #201698 ), #227672, .F. ) ;
#175542=VECTOR ( 'NONE', #160347, 1000.000000000000000 ) ;
#175544=AXIS2_PLACEMENT_3D ( 'NONE', #81731, #223826, #910 ) ;
#175546=FACE_BOUND ( 'NONE', #183931, .T. ) ;
#175597=ORIENTED_EDGE ( 'NONE', *, *, #85959, .F. ) ;
#175602=CARTESIAN_POINT ( 'NONE',  ( 20.95083306685154056, 8.916842641890202259, -8.477324853258354054 ) ) ;
#175617=EDGE_CURVE ( 'NONE', #113573, #10751, #191147, .T. ) ;
#175622=CARTESIAN_POINT ( 'NONE',  ( -18.50000000000000000, -1.164121893241208960, -41.41484808557160591 ) ) ;
#175640=CARTESIAN_POINT ( 'NONE',  ( -20.64999999999999858, -9.000000000000001776, -24.10603087734756045 ) ) ;
#175659=DIRECTION ( 'NONE',  ( -7.304098846218134667E-16, -1.000000000000000000, 0.000000000000000000 ) ) ;
#175668=EDGE_LOOP ( 'NONE', ( #101745, #132158, #7572, #205875, #32394 ) ) ;
#175674=CARTESIAN_POINT ( 'NONE',  ( 18.59999999999997655, 0.000000000000000000, -33.50000000000000000 ) ) ;
#175685=EDGE_CURVE ( 'NONE', #212201, #252532, #66375, .T. ) ;
#175717=CARTESIAN_POINT ( 'NONE',  ( 20.94999999999999574, -1.162701749938009677, -8.000000000000000000 ) ) ;
#175734=ORIENTED_EDGE ( 'NONE', *, *, #47184, .T. ) ;
#175842=CARTESIAN_POINT ( 'NONE',  ( -21.14999999999999858, 11.75000000000000000, -3.469446951953614189E-15 ) ) ;
#175886=CARTESIAN_POINT ( 'NONE',  ( 21.14999999999999858, 0.000000000000000000, 11.64957080754479968 ) ) ;
#175889=ORIENTED_EDGE ( 'NONE', *, *, #24163, .T. ) ;
#175920=LINE ( 'NONE', #220161, #21717 ) ;
#175930=DIRECTION ( 'NONE',  ( 0.000000000000000000, 0.000000000000000000, -1.000000000000000000 ) ) ;
#175936=ORIENTED_EDGE ( 'NONE', *, *, #36400, .T. ) ;
#175947=DIRECTION ( 'NONE',  ( 0.000000000000000000, 1.000000000000000000, 0.000000000000000000 ) ) ;
#175960=EDGE_LOOP ( 'NONE', ( #64368, #150254, #223419, #208613 ) ) ;
#175968=LINE ( 'NONE', #213783, #187187 ) ;
#175971=CARTESIAN_POINT ( 'NONE',  ( -23.25000000000000000, -1.835859311443637010, -45.00443916879852679 ) ) ;
#175972=ADVANCED_FACE ( 'NONE', ( #193409 ), #91721, .T. ) ;
#175990=DIRECTION ( 'NONE',  ( 0.000000000000000000, -0.000000000000000000, -1.000000000000000000 ) ) ;
#175993=CARTESIAN_POINT ( 'NONE',  ( 23.14999999999998437, -4.049999999999998934, 0.000000000000000000 ) ) ;
#176011=FACE_OUTER_BOUND ( 'NONE', #233159, .T. ) ;
#176013=CARTESIAN_POINT ( 'NONE',  ( -22.42253884134832020, 0.001932351135308873818, 11.64960569734842366 ) ) ;
#176018=AXIS2_PLACEMENT_3D ( 'NONE', #89637, #169227, #190041 ) ;
#176030=ADVANCED_FACE ( 'NONE', ( #233811 ), #134675, .F. ) ;
#176039=CARTESIAN_POINT ( 'NONE',  ( 18.52928932304149967, 10.27928932304150678, -24.67625343280360894 ) ) ;
#176049=CARTESIAN_POINT ( 'NONE',  ( -20.85000000000000142, 7.021664781900089913, -37.13356540189729316 ) ) ;
#176061=FACE_OUTER_BOUND ( 'NONE', #241219, .T. ) ;
#176074=LINE ( 'NONE', #216444, #107753 ) ;
#176085=CIRCLE ( 'NONE', #67723, 0.09999999999999939493 ) ;
#176109=DIRECTION ( 'NONE',  ( 0.000000000000000000, 0.000000000000000000, -1.000000000000000000 ) ) ;
#176124=LINE ( 'NONE', #213942, #214118 ) ;
#176143=EDGE_CURVE ( 'NONE', #214669, #106265, #79187, .T. ) ;
#176147=CYLINDRICAL_SURFACE ( 'NONE', #95517, 0.1000000000000002554 ) ;
#176149=CIRCLE ( 'NONE', #63690, 0.09999999999999939493 ) ;
#176168=CYLINDRICAL_SURFACE ( 'NONE', #55408, 0.09999999999999939493 ) ;
#176172=CARTESIAN_POINT ( 'NONE',  ( 20.95052659398289308, 10.47982436777990323, -7.575238755865602691 ) ) ;
#176173=CARTESIAN_POINT ( 'NONE',  ( -21.05000000000000071, 0.000000000000000000, -4.299999999999956302 ) ) ;
#176194=VERTEX_POINT ( 'NONE', #310 ) ;
#176206=CIRCLE ( 'NONE', #72737, 11.79999999999999716 ) ;
#176208=CIRCLE ( 'NONE', #76210, 0.1000000000000001860 ) ;
#176220=DIRECTION ( 'NONE',  ( 0.000000000000000000, 0.000000000000000000, -1.000000000000000000 ) ) ;
#176237=EDGE_LOOP ( 'NONE', ( #162176, #95325, #110772 ) ) ;
#176251=ORIENTED_EDGE ( 'NONE', *, *, #217371, .F. ) ;
#176260=DIRECTION ( 'NONE',  ( -1.000000000000000000, 0.000000000000000000, 0.000000000000000000 ) ) ;
#176286=ORIENTED_EDGE ( 'NONE', *, *, #199348, .F. ) ;
#176304=ORIENTED_EDGE ( 'NONE', *, *, #73190, .T. ) ;
#176309=CYLINDRICAL_SURFACE ( 'NONE', #69042, 0.09999999999999939493 ) ;
#176346=DIRECTION ( 'NONE',  ( 0.000000000000000000, 8.673617379884030739E-15, -1.000000000000000000 ) ) ;
#176369=AXIS2_PLACEMENT_3D ( 'NONE', #184355, #65701, #180526 ) ;
#176380=VERTEX_POINT ( 'NONE', #26831 ) ;
#176398=VERTEX_POINT ( 'NONE', #241992 ) ;
#176399=AXIS2_PLACEMENT_3D ( 'NONE', #156746, #137150, #217945 ) ;
#176402=ADVANCED_FACE ( 'NONE', ( #67209 ), #245851, .F. ) ;
#176485=DIRECTION ( 'NONE',  ( -1.000000000000000000, -0.000000000000000000, 0.000000000000000000 ) ) ;
#176501=CARTESIAN_POINT ( 'NONE',  ( -18.59999999999999787, -1.835859311443637010, -45.00443916879852679 ) ) ;
#176505=ORIENTED_EDGE ( 'NONE', *, *, #194278, .F. ) ;
#176510=ADVANCED_FACE ( 'NONE', ( #182030 ), #67391, .F. ) ;
#176514=ADVANCED_FACE ( 'NONE', ( #3364 ), #179842, .T. ) ;
#176517=EDGE_LOOP ( 'NONE', ( #65214, #19817, #115301, #136339 ) ) ;
#176528=EDGE_CURVE ( 'NONE', #134956, #16525, #238062, .T. ) ;
#176536=ORIENTED_EDGE ( 'NONE', *, *, #121171, .F. ) ;
#176552=DIRECTION ( 'NONE',  ( 1.000000000000000000, 0.000000000000000000, 0.000000000000000000 ) ) ;
#176554=EDGE_LOOP ( 'NONE', ( #130407, #121537, #17444, #86468 ) ) ;
#176576=ORIENTED_EDGE ( 'NONE', *, *, #43814, .T. ) ;
#176578=AXIS2_PLACEMENT_3D ( 'NONE', #149670, #33603, #193923 ) ;
#176613=CYLINDRICAL_SURFACE ( 'NONE', #249488, 0.09999999999999939493 ) ;
#176639=CARTESIAN_POINT ( 'NONE',  ( -21.93340585898930328, -5.963111948670274387E-16, 7.324147022125356621 ) ) ;
#176659=CARTESIAN_POINT ( 'NONE',  ( -21.05000000000000071, -11.29603075033528548, -3.047899159663867152 ) ) ;
#176669=CARTESIAN_POINT ( 'NONE',  ( 18.59999999999999076, 6.982009704856455556, -37.19615211825629331 ) ) ;
#176673=AXIS2_PLACEMENT_3D ( 'NONE', #49788, #172362, #94047 ) ;
#176729=CIRCLE ( 'NONE', #172666, 0.09999999999999939493 ) ;
#176737=DIRECTION ( 'NONE',  ( 0.000000000000000000, 3.552713678800499352E-15, -1.000000000000000000 ) ) ;
#176738=ORIENTED_EDGE ( 'NONE', *, *, #172978, .T. ) ;
#176762=DIRECTION ( 'NONE',  ( 1.000000000000000000, 0.000000000000000000, 0.000000000000000000 ) ) ;
#176773=EDGE_LOOP ( 'NONE', ( #105052, #92811, #141073, #111762 ) ) ;
#176787=AXIS2_PLACEMENT_3D ( 'NONE', #126655, #48393, #207498 ) ;
#176788=CYLINDRICAL_SURFACE ( 'NONE', #182226, 0.09999999999999939493 ) ;
#176810=CARTESIAN_POINT ( 'NONE',  ( 23.25000000000000000, -9.600000000000003197, -9.893969122652443104 ) ) ;
#176825=ADVANCED_FACE ( 'NONE', ( #169596 ), #249102, .F. ) ;
#176867=LINE ( 'NONE', #256307, #76442 ) ;
#176869=EDGE_CURVE ( 'NONE', #12754, #246027, #238252, .T. ) ;
#176880=DIRECTION ( 'NONE',  ( 0.000000000000000000, 0.9908441862701596881, 0.1350103645451904977 ) ) ;
#176904=EDGE_LOOP ( 'NONE', ( #223481, #169152, #119909, #163134 ) ) ;
#176968=ORIENTED_EDGE ( 'NONE', *, *, #111867, .T. ) ;
#176977=LINE ( 'NONE', #114405, #46156 ) ;
#177012=DIRECTION ( 'NONE',  ( -1.000000000000000000, 0.000000000000000000, 0.000000000000000000 ) ) ;
#177013=ORIENTED_EDGE ( 'NONE', *, *, #18480, .F. ) ;
#177017=DIRECTION ( 'NONE',  ( 0.000000000000000000, 2.664535259100376091E-15, 1.000000000000000000 ) ) ;
#177030=DIRECTION ( 'NONE',  ( 0.000000000000000000, 0.000000000000000000, 1.000000000000000000 ) ) ;
#177036=ORIENTED_EDGE ( 'NONE', *, *, #111081, .T. ) ;
#177058=CARTESIAN_POINT ( 'NONE',  ( 21.05000000000000071, 6.257814610476131634, 0.09779029130878996723 ) ) ;
#177059=DIRECTION ( 'NONE',  ( 0.000000000000000000, -1.000000000000000000, 1.387778780781442047E-14 ) ) ;
#177094=CARTESIAN_POINT ( 'NONE',  ( -18.59999999999999787, 11.64999999999999680, 11.75000000000000000 ) ) ;
#177126=AXIS2_PLACEMENT_3D ( 'NONE', #217452, #119671, #199201 ) ;
#177132=DIRECTION ( 'NONE',  ( 0.000000000000000000, 1.000000000000000000, -6.308085367188393199E-16 ) ) ;
#177153=ORIENTED_EDGE ( 'NONE', *, *, #214807, .T. ) ;
#177173=PLANE ( 'NONE',  #93099 ) ;
#177225=DIRECTION ( 'NONE',  ( 0.7071067811865475727, 0.7071067811865475727, -0.000000000000000000 ) ) ;
#177232=LINE ( 'NONE', #256685, #105196 ) ;
#177247=DIRECTION ( 'NONE',  ( 0.000000000000000000, -0.4930308989875248349, -0.8700118002898312719 ) ) ;
#177248=ORIENTED_EDGE ( 'NONE', *, *, #211216, .F. ) ;
#177256=VERTEX_POINT ( 'NONE', #74027 ) ;
#177261=LINE ( 'NONE', #152566, #69687 ) ;
#177276=CARTESIAN_POINT ( 'NONE',  ( 20.13684514580102913, 9.495855392750403468, -8.143031685684873011 ) ) ;
#177304=DIRECTION ( 'NONE',  ( 1.000000000000000000, -0.000000000000000000, -0.000000000000000000 ) ) ;
#177306=CARTESIAN_POINT ( 'NONE',  ( -21.04999999999999716, -0.08574093703340139594, 6.413826288812968457 ) ) ;
#177307=DIRECTION ( 'NONE',  ( 0.000000000000000000, -1.000000000000000000, 0.000000000000000000 ) ) ;
#177311=CARTESIAN_POINT ( 'NONE',  ( -21.05000000000000071, 5.899999999999947065, -10.21909976465641456 ) ) ;
#177325=CARTESIAN_POINT ( 'NONE',  ( -23.25000000000000000, 0.000000000000000000, 0.000000000000000000 ) ) ;
#177333=DIRECTION ( 'NONE',  ( 0.000000000000000000, 0.000000000000000000, -1.000000000000000000 ) ) ;
#177355=ORIENTED_EDGE ( 'NONE', *, *, #113697, .F. ) ;
#177365=DIRECTION ( 'NONE',  ( 0.000000000000000000, 0.000000000000000000, 1.000000000000000000 ) ) ;
#177411=VERTEX_POINT ( 'NONE', #58258 ) ;
#177431=CIRCLE ( 'NONE', #193980, 0.5000000000000004441 ) ;
#177446=ORIENTED_EDGE ( 'NONE', *, *, #179705, .T. ) ;
#177466=CARTESIAN_POINT ( 'NONE',  ( 20.95265033839679347, 10.51225083246715819, -7.565763756029960874 ) ) ;
#177480=ORIENTED_EDGE ( 'NONE', *, *, #123595, .T. ) ;
#177489=EDGE_CURVE ( 'NONE', #257228, #162975, #82236, .T. ) ;
#177521=ORIENTED_EDGE ( 'NONE', *, *, #129763, .F. ) ;
#177525=EDGE_CURVE ( 'NONE', #250352, #210177, #252958, .T. ) ;
#177527=ORIENTED_EDGE ( 'NONE', *, *, #185221, .F. ) ;
#177530=CARTESIAN_POINT ( 'NONE',  ( 23.14999999999999147, 0.000000000000000000, 0.000000000000000000 ) ) ;
#177535=DIRECTION ( 'NONE',  ( -1.000000000000000000, 0.000000000000000000, 0.000000000000000000 ) ) ;
#177566=CARTESIAN_POINT ( 'NONE',  ( -21.05000000000000071, 0.000000000000000000, 0.000000000000000000 ) ) ;
#177576=DIRECTION ( 'NONE',  ( 0.000000000000000000, 0.000000000000000000, -1.000000000000000000 ) ) ;
#177691=CIRCLE ( 'NONE', #52731, 0.09999999999999939493 ) ;
#177693=EDGE_CURVE ( 'NONE', #113100, #40685, #252563, .T. ) ;
#177697=CARTESIAN_POINT ( 'NONE',  ( -18.46907102845853998, -9.473727364764107151, -40.17603473873652575 ) ) ;
#177700=ORIENTED_EDGE ( 'NONE', *, *, #233901, .T. ) ;
#177704=EDGE_CURVE ( 'NONE', #108030, #28028, #130092, .T. ) ;
#177777=AXIS2_PLACEMENT_3D ( 'NONE', #170328, #131145, #224147 ) ;
#177778=ORIENTED_EDGE ( 'NONE', *, *, #98384, .F. ) ;
#177816=VERTEX_POINT ( 'NONE', #206464 ) ;
#177826=EDGE_LOOP ( 'NONE', ( #212771, #194471, #7004, #53421 ) ) ;
#177915=ORIENTED_EDGE ( 'NONE', *, *, #184766, .T. ) ;
#177926=CARTESIAN_POINT ( 'NONE',  ( -22.39999999999999858, -0.1008583690987139431, 11.74956712348939192 ) ) ;
#177952=CIRCLE ( 'NONE', #211276, 0.09999999999999939493 ) ;
#178011=EDGE_CURVE ( 'NONE', #165206, #243103, #257193, .T. ) ;
#178016=VERTEX_POINT ( 'NONE', #92921 ) ;
#178017=FACE_OUTER_BOUND ( 'NONE', #131565, .T. ) ;
#178018=CARTESIAN_POINT ( 'NONE',  ( -23.15000000000000213, 5.082284216461513184E-16, 4.149999999999999467 ) ) ;
#178048=CARTESIAN_POINT ( 'NONE',  ( 19.75857864376268935, 11.75000000000000355, -24.85000000000000142 ) ) ;
#178072=EDGE_CURVE ( 'NONE', #123338, #51281, #219420, .T. ) ;
#178120=DIRECTION ( 'NONE',  ( -0.000000000000000000, 3.469446951953635015E-14, 1.000000000000000000 ) ) ;
#178142=DIRECTION ( 'NONE',  ( 0.000000000000000000, 0.000000000000000000, -1.000000000000000000 ) ) ;
#178146=AXIS2_PLACEMENT_3D ( 'NONE', #14848, #94341, #192192 ) ;
#178156=CARTESIAN_POINT ( 'NONE',  ( -18.59999999999999787, -9.400000000000005684, -40.38204184817266906 ) ) ;
#178167=EDGE_CURVE ( 'NONE', #17846, #182491, #75945, .T. ) ;
#178179=DIRECTION ( 'NONE',  ( 0.000000000000000000, 0.000000000000000000, -1.000000000000000000 ) ) ;
#178233=DIRECTION ( 'NONE',  ( 1.000000000000000000, 0.000000000000000000, 0.000000000000000000 ) ) ;
#178296=CARTESIAN_POINT ( 'NONE',  ( -22.50000000000094502, 0.1008583690986050579, 11.74956712348940613 ) ) ;
#178301=ORIENTED_EDGE ( 'NONE', *, *, #220877, .T. ) ;
#178306=CARTESIAN_POINT ( 'NONE',  ( -18.59999999999999787, 1.162701749938009677, -8.099999999999999645 ) ) ;
#178308=ORIENTED_EDGE ( 'NONE', *, *, #29878, .F. ) ;
#178313=EDGE_CURVE ( 'NONE', #119379, #153971, #244376, .T. ) ;
#178317=AXIS2_PLACEMENT_3D ( 'NONE', #205025, #9409, #87657 ) ;
#178341=CARTESIAN_POINT ( 'NONE',  ( 21.04999999999999716, 6.344359042043513419, 0.01485563489366281686 ) ) ;
#178356=AXIS2_PLACEMENT_3D ( 'NONE', #105218, #107835, #89541 ) ;
#178372=ORIENTED_EDGE ( 'NONE', *, *, #178072, .F. ) ;
#178374=CARTESIAN_POINT ( 'NONE',  ( 22.50046968638104516, 0.04516984714028955683, 11.75004515447417930 ) ) ;
#178408=CARTESIAN_POINT ( 'NONE',  ( -22.39999999999999858, 11.65000000000000036, 0.09999999999999592548 ) ) ;
#178415=DIRECTION ( 'NONE',  ( 0.000000000000000000, 0.000000000000000000, -1.000000000000000000 ) ) ;
#178417=AXIS2_PLACEMENT_3D ( 'NONE', #234696, #162391, #99800 ) ;
#178493=VERTEX_POINT ( 'NONE', #140403 ) ;
#178495=CARTESIAN_POINT ( 'NONE',  ( -21.14999999999999858, -0.09999999999999939493, 11.64957080754479968 ) ) ;
#178507=DIRECTION ( 'NONE',  ( 1.000000000000000000, 0.000000000000000000, 0.000000000000000000 ) ) ;
#178509=TOROIDAL_SURFACE ( 'NONE', #66041, 3.899999999999999467, 0.1000000000000000056 ) ;
#178577=DIRECTION ( 'NONE',  ( 0.000000000000000000, 0.4999999999999994449, 0.8660254037844390407 ) ) ;
#178609=CARTESIAN_POINT ( 'NONE',  ( 18.49999999999998934, 10.37342005527971800, -24.76578812462619794 ) ) ;
#178610=FACE_OUTER_BOUND ( 'NONE', #60018, .T. ) ;
#178612=EDGE_CURVE ( 'NONE', #63069, #131644, #48920, .T. ) ;
#178679=CIRCLE ( 'NONE', #203579, 7.900000000000000355 ) ;
#178685=LINE ( 'NONE', #7238, #207567 ) ;
#178692=ORIENTED_EDGE ( 'NONE', *, *, #183659, .T. ) ;
#178710=ORIENTED_EDGE ( 'NONE', *, *, #45812, .F. ) ;
#178713=CARTESIAN_POINT ( 'NONE',  ( 21.08884785362045378, 6.357193367425240105, 0.04978309506684791552 ) ) ;
#178738=VERTEX_POINT ( 'NONE', #56684 ) ;
#178741=ORIENTED_EDGE ( 'NONE', *, *, #220206, .F. ) ;
#178755=CIRCLE ( 'NONE', #237158, 0.2000000000000005107 ) ;
#178758=CARTESIAN_POINT ( 'NONE',  ( 20.95035502843362707, 10.47763832677646789, -7.576299708736373262 ) ) ;
#178760=EDGE_LOOP ( 'NONE', ( #97154, #187623, #194285, #110725 ) ) ;
#178772=DIRECTION ( 'NONE',  ( 0.000000000000000000, 1.897661533703519897E-16, -1.000000000000000000 ) ) ;
#178783=VECTOR ( 'NONE', #74954, 1000.000000000000000 ) ;
#178822=EDGE_LOOP ( 'NONE', ( #90591, #128794, #250774, #75239 ) ) ;
#178824=CARTESIAN_POINT ( 'NONE',  ( -18.59999999999999787, 7.120270961697594103, -37.15956304183931991 ) ) ;
#178835=CIRCLE ( 'NONE', #20594, 3.900000000000000799 ) ;
#178875=CARTESIAN_POINT ( 'NONE',  ( -23.15000000000000213, 0.000000000000000000, 0.000000000000000000 ) ) ;
#178888=EDGE_CURVE ( 'NONE', #136601, #38380, #40786, .T. ) ;
#178923=ADVANCED_FACE ( 'NONE', ( #119279 ), #123965, .T. ) ;
#178928=CARTESIAN_POINT ( 'NONE',  ( -18.59999999999999787, 1.866714910057309273, -11.75267524628200633 ) ) ;
#179008=EDGE_LOOP ( 'NONE', ( #124159, #188566, #228180, #191620 ) ) ;
#179010=VERTEX_POINT ( 'NONE', #107400 ) ;
#179012=CARTESIAN_POINT ( 'NONE',  ( 18.43565242384934422, -9.519327731092435130, -6.972976376559337552 ) ) ;
#179019=CARTESIAN_POINT ( 'NONE',  ( -21.05000000000000071, -11.48912529307605901, -3.100000000000000533 ) ) ;
#179023=AXIS2_PLACEMENT_3D ( 'NONE', #142700, #24081, #222226 ) ;
#179037=CARTESIAN_POINT ( 'NONE',  ( -21.05000000000000071, 0.09779029130879170195, 6.257814610476114758 ) ) ;
#179050=EDGE_LOOP ( 'NONE', ( #217379, #106931, #9517 ) ) ;
#179102=TOROIDAL_SURFACE ( 'NONE', #224839, 0.2000000000000000111, 0.1000000000000000056 ) ;
#179117=DIRECTION ( 'NONE',  ( -1.000000000000000000, -0.000000000000000000, 0.000000000000000000 ) ) ;
#179125=ORIENTED_EDGE ( 'NONE', *, *, #183711, .T. ) ;
#179131=DIRECTION ( 'NONE',  ( 1.000000000000000000, 7.304098846218134667E-16, -4.607487905232622991E-31 ) ) ;
#179143=DIRECTION ( 'NONE',  ( 1.000000000000000000, 0.000000000000000000, -0.000000000000000000 ) ) ;
#179146=CARTESIAN_POINT ( 'NONE',  ( 20.95512820512820440, 8.876151316288115822, -8.558628995140949769 ) ) ;
#179173=DIRECTION ( 'NONE',  ( 0.000000000000000000, -0.9908441862701596881, 0.1350103645451904977 ) ) ;
#179180=ADVANCED_FACE ( 'NONE', ( #13455 ), #57478, .F. ) ;
#179182=ORIENTED_EDGE ( 'NONE', *, *, #5388, .T. ) ;
#179184=CARTESIAN_POINT ( 'NONE',  ( -20.64999999999999858, 7.249999999999999112, -21.15000000000000213 ) ) ;
#179205=ORIENTED_EDGE ( 'NONE', *, *, #116270, .T. ) ;
#179215=DIRECTION ( 'NONE',  ( 0.000000000000000000, 0.000000000000000000, -1.000000000000000000 ) ) ;
#179236=LINE ( 'NONE', #38417, #124233 ) ;
#179297=ORIENTED_EDGE ( 'NONE', *, *, #52512, .T. ) ;
#179312=DIRECTION ( 'NONE',  ( 0.000000000000000000, 0.000000000000000000, -1.000000000000000000 ) ) ;
#179325=EDGE_LOOP ( 'NONE', ( #174537, #98471, #51756, #145270 ) ) ;
#179361=DIRECTION ( 'NONE',  ( -0.000000000000000000, 0.8660254037844502539, 0.4999999999999799050 ) ) ;
#179387=DIRECTION ( 'NONE',  ( 0.000000000000000000, 0.000000000000000000, -1.000000000000000000 ) ) ;
#179399=PLANE ( 'NONE',  #236776 ) ;
#179430=DIRECTION ( 'NONE',  ( -1.000000000000000000, -0.000000000000000000, -0.000000000000000000 ) ) ;
#179452=DIRECTION ( 'NONE',  ( -1.000000000000000000, -0.000000000000000000, 0.000000000000000000 ) ) ;
#179477=ORIENTED_EDGE ( 'NONE', *, *, #7672, .T. ) ;
#179503=ADVANCED_FACE ( 'NONE', ( #187933 ), #124115, .T. ) ;
#179521=DIRECTION ( 'NONE',  ( -0.000000000000000000, -0.000000000000000000, -1.000000000000000000 ) ) ;
#179583=TOROIDAL_SURFACE ( 'NONE', #133753, 4.099999999999999645, 0.1000000000000000056 ) ;
#179623=CARTESIAN_POINT ( 'NONE',  ( -18.59999999999999787, -1.164121893241208960, -41.31484808557160449 ) ) ;
#179636=CARTESIAN_POINT ( 'NONE',  ( 21.05000000000000071, -0.01759718700860490523, 6.440770893661947660 ) ) ;
#179638=DIRECTION ( 'NONE',  ( 1.000000000000000000, 0.000000000000000000, 0.000000000000000000 ) ) ;
#179648=CARTESIAN_POINT ( 'NONE',  ( 22.40000000000010516, -9.465491541613135773E-13, 11.64957080754511232 ) ) ;
#179656=DIRECTION ( 'NONE',  ( 0.000000000000000000, 0.000000000000000000, 1.000000000000000000 ) ) ;
#179705=EDGE_CURVE ( 'NONE', #141418, #36387, #61962, .T. ) ;
#179706=AXIS2_PLACEMENT_3D ( 'NONE', #110619, #94894, #134023 ) ;
#179744=EDGE_CURVE ( 'NONE', #103735, #16503, #74475, .T. ) ;
#179755=DIRECTION ( 'NONE',  ( 0.000000000000000000, -1.000000000000000000, 0.000000000000000000 ) ) ;
#179763=ADVANCED_FACE ( 'NONE', ( #71396 ), #230451, .T. ) ;
#179776=ADVANCED_FACE ( 'NONE', ( #209605 ), #178509, .T. ) ;
#179829=CARTESIAN_POINT ( 'NONE',  ( 20.97565083910961548, 10.47461740127880958, -7.577943176588548546 ) ) ;
#179842=TOROIDAL_SURFACE ( 'NONE', #88204, 11.89999999999999858, 0.1000000000000000056 ) ;
#179854=DIRECTION ( 'NONE',  ( 1.000000000000000000, 3.265361837132813093E-16, -0.000000000000000000 ) ) ;
#179857=CARTESIAN_POINT ( 'NONE',  ( 22.60000000000000142, 0.000000000000000000, 0.000000000000000000 ) ) ;
#179883=DIRECTION ( 'NONE',  ( 1.000000000000000000, 0.000000000000000000, 0.000000000000000000 ) ) ;
#179916=CARTESIAN_POINT ( 'NONE',  ( 20.94999999999999574, 1.249999999999999334, -7.900000000000000355 ) ) ;
#179920=CARTESIAN_POINT ( 'NONE',  ( 21.05000000000000071, 0.000000000000000000, -33.50000000000000000 ) ) ;
#179933=EDGE_LOOP ( 'NONE', ( #152588, #162406, #78692, #28984 ) ) ;
#179976=ORIENTED_EDGE ( 'NONE', *, *, #198164, .F. ) ;
#180003=VERTEX_POINT ( 'NONE', #150594 ) ;
#180004=CIRCLE ( 'NONE', #4981, 0.1000000000000002554 ) ;
#180025=DIRECTION ( 'NONE',  ( -1.000000000000000000, 0.000000000000000000, 0.000000000000000000 ) ) ;
#180038=VERTEX_POINT ( 'NONE', #39659 ) ;
#180052=ADVANCED_FACE ( 'NONE', ( #78733 ), #235251, .F. ) ;
#180059=DIRECTION ( 'NONE',  ( -0.000000000000000000, -0.000000000000000000, -1.000000000000000000 ) ) ;
#180107=DIRECTION ( 'NONE',  ( 1.000000000000000000, 0.000000000000000000, -0.000000000000000000 ) ) ;
#180109=ORIENTED_EDGE ( 'NONE', *, *, #155728, .T. ) ;
#180123=ORIENTED_EDGE ( 'NONE', *, *, #257779, .T. ) ;
#180132=DIRECTION ( 'NONE',  ( 1.000000000000000000, -0.000000000000000000, -0.000000000000000000 ) ) ;
#180148=DIRECTION ( 'NONE',  ( 1.000000000000000000, 0.000000000000000000, 0.000000000000000000 ) ) ;
#180170=VECTOR ( 'NONE', #28209, 1000.000000000000114 ) ;
#180176=DIRECTION ( 'NONE',  ( 0.000000000000000000, -2.428612866367527723E-14, -1.000000000000000000 ) ) ;
#180197=CARTESIAN_POINT ( 'NONE',  ( 21.05000000000000071, 0.000000000000000000, -35.50000000000000711 ) ) ;
#180213=CARTESIAN_POINT ( 'NONE',  ( -2.995603634470884209E-16, -11.75000000000000000, -21.25000000000000000 ) ) ;
#180219=CARTESIAN_POINT ( 'NONE',  ( -18.60000000000000142, -9.523954320752791247, -40.38201705682730847 ) ) ;
#180274=CIRCLE ( 'NONE', #88467, 0.09999999999999867328 ) ;
#180300=ORIENTED_EDGE ( 'NONE', *, *, #228889, .T. ) ;
#180318=ADVANCED_FACE ( 'NONE', ( #228551 ), #150301, .F. ) ;
#180321=CIRCLE ( 'NONE', #63602, 0.09999999999999967248 ) ;
#180381=FACE_OUTER_BOUND ( 'NONE', #241056, .T. ) ;
#180404=PLANE ( 'NONE',  #174384 ) ;
#180442=DIRECTION ( 'NONE',  ( -0.000000000000000000, 1.000000000000000000, 0.000000000000000000 ) ) ;
#180460=DIRECTION ( 'NONE',  ( 0.000000000000000000, 0.000000000000000000, -1.000000000000000000 ) ) ;
#180465=ORIENTED_EDGE ( 'NONE', *, *, #247179, .T. ) ;
#180486=FACE_OUTER_BOUND ( 'NONE', #84499, .T. ) ;
#180526=DIRECTION ( 'NONE',  ( -0.7071067811865388020, 0.7071067811865561215, 0.000000000000000000 ) ) ;
#180563=ORIENTED_EDGE ( 'NONE', *, *, #184534, .T. ) ;
#180587=ADVANCED_FACE ( 'NONE', ( #21083 ), #220543, .T. ) ;
#180594=AXIS2_PLACEMENT_3D ( 'NONE', #129041, #207307, #127760 ) ;
#180598=LINE ( 'NONE', #81457, #216925 ) ;
#180601=CARTESIAN_POINT ( 'NONE',  ( 19.92426406871192412, 11.75000000000000711, -24.85000000000000142 ) ) ;
#180626=VECTOR ( 'NONE', #158123, 1000.000000000000000 ) ;
#180654=VERTEX_POINT ( 'NONE', #27518 ) ;
#180655=VECTOR ( 'NONE', #202415, 1000.000000000000000 ) ;
#180662=DIRECTION ( 'NONE',  ( -1.000000000000000000, 0.000000000000000000, 0.000000000000000000 ) ) ;
#180686=DIRECTION ( 'NONE',  ( -1.000000000000000000, 0.000000000000000000, 0.000000000000000000 ) ) ;
#180689=ORIENTED_EDGE ( 'NONE', *, *, #164477, .T. ) ;
#180693=ORIENTED_EDGE ( 'NONE', *, *, #104171, .F. ) ;
#180723=CIRCLE ( 'NONE', #5904, 11.65000000000000036 ) ;
#180748=EDGE_LOOP ( 'NONE', ( #77218, #139596, #133950, #39240, #226429 ) ) ;
#180779=EDGE_CURVE ( 'NONE', #124163, #239652, #254031, .T. ) ;
#180812=AXIS2_PLACEMENT_3D ( 'NONE', #47340, #222114, #205127 ) ;
#180820=CIRCLE ( 'NONE', #39188, 4.049999999999998934 ) ;
#180825=CARTESIAN_POINT ( 'NONE',  ( -20.85000000000000142, 7.120270961697594103, -37.15956304183931991 ) ) ;
#180845=EDGE_CURVE ( 'NONE', #227113, #23245, #203968, .T. ) ;
#180858=DIRECTION ( 'NONE',  ( -1.000000000000000000, 0.000000000000000000, 0.000000000000000000 ) ) ;
#180912=CARTESIAN_POINT ( 'NONE',  ( 21.05000000000000071, -11.29603075033528548, -3.047899159663867152 ) ) ;
#180986=EDGE_CURVE ( 'NONE', #133804, #98230, #237300, .T. ) ;
#180993=VERTEX_POINT ( 'NONE', #51839 ) ;
#181005=FACE_BOUND ( 'NONE', #88877, .T. ) ;
#181007=ORIENTED_EDGE ( 'NONE', *, *, #81664, .T. ) ;
#181029=DIRECTION ( 'NONE',  ( 0.000000000000000000, 0.000000000000000000, 1.000000000000000000 ) ) ;
#181056=FACE_OUTER_BOUND ( 'NONE', #80236, .T. ) ;
#181089=CARTESIAN_POINT ( 'NONE',  ( -18.50000000000000000, 9.150000000000002132, -21.15000000000000213 ) ) ;
#181110=( BOUNDED_SURFACE ( )  B_SPLINE_SURFACE ( 3, 2, ( 
 ( #134097, #10334, #252759 ),
 ( #234483, #75452, #15468 ),
 ( #190247, #152425, #93700 ),
 ( #135378, #211087, #74178 ),
 ( #35053, #230658, #154986 ),
 ( #55821, #70325, #151119 ),
 ( #214930, #14194, #113267 ),
 ( #115832, #32485, #173296 ),
 ( #153735, #149846, #131546 ),
 ( #231952, #229377, #53297 ) ),
 .UNSPECIFIED., .F., .F., .F. ) 
 B_SPLINE_SURFACE_WITH_KNOTS ( ( 4, 2, 2, 2, 4 ),
 ( 3, 3 ),
 ( 0.0001701955120502369480, 0.0002247052511886134046, 0.0002792149903269898611, 0.0003882344686037427200, 0.0006062734251572484377 ),
 ( 0.000000000000000000, 1.000000000000000000 ),
 .UNSPECIFIED. ) 
 GEOMETRIC_REPRESENTATION_ITEM ( )  RATIONAL_B_SPLINE_SURFACE ( (
 ( 1.000000000000000000, 0.2966190024560417804, 1.000000000000000000),
 ( 1.000000000000000000, 0.2964522492711155199, 1.000000000000000000),
 ( 1.000000000000000000, 0.3059923531884136128, 1.000000000000000000),
 ( 1.000000000000000000, 0.3355751146944749297, 1.000000000000000000),
 ( 1.000000000000000000, 0.3550672384963041162, 1.000000000000000000),
 ( 1.000000000000000000, 0.4157034672181008084, 1.000000000000000000),
 ( 1.000000000000000000, 0.4588031877652027912, 1.000000000000000000),
 ( 1.000000000000000000, 0.5771441759664686089, 1.000000000000000000),
 ( 1.000000000000000000, 0.6469377121768989936, 1.000000000000000000),
 ( 1.000000000000000000, 0.7071067811865475727, 1.000000000000000000) ) ) 
 REPRESENTATION_ITEM ( '' )  SURFACE ( )  );
#181112=CARTESIAN_POINT ( 'NONE',  ( -20.85000000000000142, -1.835859311443635233, -45.00443916879852679 ) ) ;
#181114=CARTESIAN_POINT ( 'NONE',  ( 20.19326291201701196, 10.15606098790381751, -7.761861807602776331 ) ) ;
#181116=DIRECTION ( 'NONE',  ( 4.336808689942128177E-15, 0.8660254037844330455, -0.5000000000000096589 ) ) ;
#181117=ORIENTED_EDGE ( 'NONE', *, *, #174461, .F. ) ;
#181136=DIRECTION ( 'NONE',  ( 1.000000000000000000, 2.952720810173289112E-16, -0.000000000000000000 ) ) ;
#181140=DIRECTION ( 'NONE',  ( 1.000000000000000000, 0.000000000000000000, 0.000000000000000000 ) ) ;
#181147=CIRCLE ( 'NONE', #106076, 0.09999999999999967248 ) ;
#181148=AXIS2_PLACEMENT_3D ( 'NONE', #187024, #13510, #153055 ) ;
#181169=LINE ( 'NONE', #217679, #159484 ) ;
#181172=DIRECTION ( 'NONE',  ( 1.000000000000000000, 0.000000000000000000, 0.000000000000000000 ) ) ;
#181187=CIRCLE ( 'NONE', #60529, 0.1000000000000000472 ) ;
#181301=CARTESIAN_POINT ( 'NONE',  ( -20.85000000000000142, -1.851617760468904805, -45.10318971960366241 ) ) ;
#181302=CARTESIAN_POINT ( 'NONE',  ( 18.59999999999999432, -1.637172712970379918, -11.58215336547201701 ) ) ;
#181314=CYLINDRICAL_SURFACE ( 'NONE', #210198, 0.09999999999999939493 ) ;
#181339=ORIENTED_EDGE ( 'NONE', *, *, #208897, .F. ) ;
#181366=DIRECTION ( 'NONE',  ( 0.000000000000000000, 4.336808689941893885E-15, 1.000000000000000000 ) ) ;
#181383=DIRECTION ( 'NONE',  ( 0.000000000000000000, 0.000000000000000000, -1.000000000000000000 ) ) ;
#181407=DIRECTION ( 'NONE',  ( -1.000000000000000000, -0.000000000000000000, -0.000000000000000000 ) ) ;
#181436=CARTESIAN_POINT ( 'NONE',  ( 23.14999999999999503, 11.65000000000000746, -12.15000000000000036 ) ) ;
#181451=LINE ( 'NONE', #2776, #239423 ) ;
#181457=CIRCLE ( 'NONE', #169172, 0.09999999999999939493 ) ;
#181468=DIRECTION ( 'NONE',  ( 0.000000000000000000, -0.000000000000000000, 1.000000000000000000 ) ) ;
#181473=LINE ( 'NONE', #204850, #145472 ) ;
#181481=EDGE_LOOP ( 'NONE', ( #5431, #66705, #163398, #219737 ) ) ;
#181572=CARTESIAN_POINT ( 'NONE',  ( -20.94403535211772294, 10.30632246270531738, -39.00418367788957852 ) ) ;
#181573=DIRECTION ( 'NONE',  ( 0.000000000000000000, 0.000000000000000000, 1.000000000000000000 ) ) ;
#181591=EDGE_LOOP ( 'NONE', ( #36788, #64118, #200541, #52349 ) ) ;
#181606=ORIENTED_EDGE ( 'NONE', *, *, #214235, .T. ) ;
#181613=CARTESIAN_POINT ( 'NONE',  ( 23.14999999999999858, 4.775700934579428569, -11.84876810404597158 ) ) ;
#181627=EDGE_LOOP ( 'NONE', ( #58174, #193022, #20421, #83957 ) ) ;
#181705=FACE_OUTER_BOUND ( 'NONE', #179050, .T. ) ;
#181721=ORIENTED_EDGE ( 'NONE', *, *, #90771, .T. ) ;
#181736=CARTESIAN_POINT ( 'NONE',  ( -18.52643265882458579, 10.31973158070286978, -39.05053347133545572 ) ) ;
#181743=CARTESIAN_POINT ( 'NONE',  ( -20.96428641294235717, 11.75000000000033928, -26.67489317794143133 ) ) ;
#181744=EDGE_CURVE ( 'NONE', #144336, #39052, #50891, .T. ) ;
#181758=CARTESIAN_POINT ( 'NONE',  ( 20.85000000000000142, -1.149570369575693807, -41.31591248450196474 ) ) ;
#181767=ORIENTED_EDGE ( 'NONE', *, *, #210634, .T. ) ;
#181773=ADVANCED_FACE ( 'NONE', ( #13099 ), #10525, .T. ) ;
#181793=AXIS2_PLACEMENT_3D ( 'NONE', #144183, #201605, #243289 ) ;
#181795=AXIS2_PLACEMENT_3D ( 'NONE', #51334, #72235, #168803 ) ;
#181812=CARTESIAN_POINT ( 'NONE',  ( 18.49999999999999645, 1.728086936794461570, 13.11556499483223348 ) ) ;
#181879=AXIS2_PLACEMENT_3D ( 'NONE', #108902, #50202, #151914 ) ;
#181882=CARTESIAN_POINT ( 'NONE',  ( 18.59999999999996945, 10.33248238082518711, -39.09484654391314962 ) ) ;
#181892=DIRECTION ( 'NONE',  ( 2.694716079187272946E-16, -1.000000000000000000, 0.000000000000000000 ) ) ;
#181930=LINE ( 'NONE', #44986, #59681 ) ;
#181947=DIRECTION ( 'NONE',  ( -1.000000000000000000, -0.000000000000000000, 0.000000000000000000 ) ) ;
#181954=CARTESIAN_POINT ( 'NONE',  ( 20.94999999999999574, -11.48912529307605901, -3.000000000000002665 ) ) ;
#182030=FACE_OUTER_BOUND ( 'NONE', #204171, .T. ) ;
#182038=FACE_OUTER_BOUND ( 'NONE', #221680, .T. ) ;
#182063=AXIS2_PLACEMENT_3D ( 'NONE', #236005, #57352, #232183 ) ;
#182078=DIRECTION ( 'NONE',  ( -1.000000000000000000, 0.000000000000000000, 0.000000000000000000 ) ) ;
#182113=DIRECTION ( 'NONE',  ( -1.836970198721029934E-16, 1.000000000000000000, 0.000000000000000000 ) ) ;
#182154=CARTESIAN_POINT ( 'NONE',  ( 21.05000000000000782, -0.01681986838567536488, 6.307425219565410579 ) ) ;
#182172=DIRECTION ( 'NONE',  ( -0.000000000000000000, -0.8700118002898321601, 0.4930308989875230030 ) ) ;
#182224=ORIENTED_EDGE ( 'NONE', *, *, #146740, .F. ) ;
#182226=AXIS2_PLACEMENT_3D ( 'NONE', #92091, #256228, #157235 ) ;
#182256=AXIS2_PLACEMENT_3D ( 'NONE', #14302, #130356, #149956 ) ;
#182302=EDGE_CURVE ( 'NONE', #32767, #71370, #109007, .T. ) ;
#182329=CARTESIAN_POINT ( 'NONE',  ( -21.53752568617671059, 6.786807874503945293, 0.09897446126636783026 ) ) ;
#182342=ORIENTED_EDGE ( 'NONE', *, *, #149288, .T. ) ;
#182352=ORIENTED_EDGE ( 'NONE', *, *, #19173, .F. ) ;
#182359=AXIS2_PLACEMENT_3D ( 'NONE', #24331, #3447, #146801 ) ;
#182371=DIRECTION ( 'NONE',  ( 0.000000000000000000, 2.891205793294679805E-16, -1.000000000000000000 ) ) ;
#182385=ORIENTED_EDGE ( 'NONE', *, *, #19451, .F. ) ;
#182389=CARTESIAN_POINT ( 'NONE',  ( -18.59999999999999787, 1.162701749938009677, -8.099999999999999645 ) ) ;
#182401=CARTESIAN_POINT ( 'NONE',  ( -20.64999999999999858, 7.150000000000000355, -12.25000000000000000 ) ) ;
#182402=CARTESIAN_POINT ( 'NONE',  ( 21.05000000000000071, 6.257814610476124528, 0.09779029130879343668 ) ) ;
#182403=DIRECTION ( 'NONE',  ( 0.000000000000000000, 0.000000000000000000, -1.000000000000000000 ) ) ;
#182424=DIRECTION ( 'NONE',  ( 1.000000000000000000, 0.000000000000000000, 0.000000000000000000 ) ) ;
#182425=DIRECTION ( 'NONE',  ( 0.000000000000000000, 0.1568667991644863147, 0.9876197685951252359 ) ) ;
#182474=ORIENTED_EDGE ( 'NONE', *, *, #38418, .F. ) ;
#182484=LINE ( 'NONE', #110296, #27765 ) ;
#182491=VERTEX_POINT ( 'NONE', #46445 ) ;
#182503=CIRCLE ( 'NONE', #228282, 0.5000000000000004441 ) ;
#182572=DIRECTION ( 'NONE',  ( -1.000000000000000000, -2.952720810173289112E-16, 0.000000000000000000 ) ) ;
#182609=ORIENTED_EDGE ( 'NONE', *, *, #146143, .F. ) ;
#182625=ADVANCED_FACE ( 'NONE', ( #194980 ), #237650, .T. ) ;
#182691=CARTESIAN_POINT ( 'NONE',  ( 23.15000000000000213, -11.74999999999999112, -12.15000000000000036 ) ) ;
#182716=ADVANCED_FACE ( 'NONE', ( #154580 ), #134948, .T. ) ;
#182722=CARTESIAN_POINT ( 'NONE',  ( 21.05000000000000071, -11.64999999999999147, -2.900000000000003464 ) ) ;
#182725=CARTESIAN_POINT ( 'NONE',  ( 23.25000000000000000, -8.596261682242991142, -9.450127517150276546 ) ) ;
#182734=TOROIDAL_SURFACE ( 'NONE', #132647, 0.2000000000000000111, 0.1000000000000000056 ) ;
#182737=VECTOR ( 'NONE', #254567, 1000.000000000000000 ) ;
#182742=AXIS2_PLACEMENT_3D ( 'NONE', #227603, #48968, #196187 ) ;
#182754=CARTESIAN_POINT ( 'NONE',  ( -20.94999999999999574, 11.62071067811865177, -26.63158334765902424 ) ) ;
#182760=CARTESIAN_POINT ( 'NONE',  ( 21.13614978966381841, -3.602007608198911206E-16, 6.499104701833793740 ) ) ;
#182762=EDGE_LOOP ( 'NONE', ( #34038, #167652, #71076, #201886 ) ) ;
#182763=EDGE_CURVE ( 'NONE', #233645, #52039, #157136, .T. ) ;
#182768=EDGE_CURVE ( 'NONE', #60900, #214033, #581, .T. ) ;
#182792=CARTESIAN_POINT ( 'NONE',  ( 23.24999999999999645, 5.599999999999996980, 11.75000000000000000 ) ) ;
#182794=ORIENTED_EDGE ( 'NONE', *, *, #131123, .T. ) ;
#182814=ORIENTED_EDGE ( 'NONE', *, *, #240088, .F. ) ;
#182820=ORIENTED_EDGE ( 'NONE', *, *, #214699, .T. ) ;
#182828=DIRECTION ( 'NONE',  ( 1.000000000000000000, -0.000000000000000000, -0.000000000000000000 ) ) ;
#182837=EDGE_CURVE ( 'NONE', #81993, #248248, #183111, .T. ) ;
#182851=CARTESIAN_POINT ( 'NONE',  ( 18.58685178364169133, -9.406733083804247997, -7.124420469087726637 ) ) ;
#182862=CARTESIAN_POINT ( 'NONE',  ( -23.25000000000000000, 2.600000000000000089, -20.27537807723789953 ) ) ;
#182869=DIRECTION ( 'NONE',  ( 0.000000000000000000, 0.000000000000000000, -1.000000000000000000 ) ) ;
#182944=ORIENTED_EDGE ( 'NONE', *, *, #184122, .F. ) ;
#182967=ORIENTED_EDGE ( 'NONE', *, *, #2804, .T. ) ;
#183030=CARTESIAN_POINT ( 'NONE',  ( -18.50596464788227635, 10.30632246270531560, -39.00418367788958562 ) ) ;
#183033=AXIS2_PLACEMENT_3D ( 'NONE', #36819, #39386, #116335 ) ;
#183034=EDGE_LOOP ( 'NONE', ( #239503, #5832, #38053 ) ) ;
#183044=ORIENTED_EDGE ( 'NONE', *, *, #25519, .T. ) ;
#183051=CARTESIAN_POINT ( 'NONE',  ( -23.15000000000000213, 4.150000000000001243, 11.75000000000000000 ) ) ;
#183079=ORIENTED_EDGE ( 'NONE', *, *, #49650, .F. ) ;
#183080=VERTEX_POINT ( 'NONE', #96487 ) ;
#183096=ADVANCED_FACE ( 'NONE', ( #219014 ), #179583, .F. ) ;
#183111=LINE ( 'NONE', #181812, #246012 ) ;
#183118=EDGE_CURVE ( 'NONE', #158092, #40817, #250296, .T. ) ;
#183141=CARTESIAN_POINT ( 'NONE',  ( -23.25000000000000000, 4.349999999999999645, -21.14999999999999858 ) ) ;
#183173=EDGE_LOOP ( 'NONE', ( #109425, #3661, #251816, #210208 ) ) ;
#183203=CARTESIAN_POINT ( 'NONE',  ( -23.25000000000000000, -11.65000000000000036, -30.39999999999999858 ) ) ;
#183232=FACE_OUTER_BOUND ( 'NONE', #235836, .T. ) ;
#183241=CARTESIAN_POINT ( 'NONE',  ( -18.59999999999999787, 1.340746217933695750, 10.27286250542118040 ) ) ;
#183242=VERTEX_POINT ( 'NONE', #128921 ) ;
#183269=DIRECTION ( 'NONE',  ( -1.000000000000000000, 0.000000000000000000, 3.469446951953635015E-14 ) ) ;
#183282=VERTEX_POINT ( 'NONE', #11549 ) ;
#183287=ORIENTED_EDGE ( 'NONE', *, *, #5826, .F. ) ;
#183289=EDGE_CURVE ( 'NONE', #163426, #105990, #29756, .T. ) ;
#183320=CARTESIAN_POINT ( 'NONE',  ( -23.15000000000000213, 11.65000000000000036, -12.14999999999999858 ) ) ;
#183333=EDGE_CURVE ( 'NONE', #84692, #33602, #34041, .T. ) ;
#183346=FACE_OUTER_BOUND ( 'NONE', #101175, .T. ) ;
#183382=DIRECTION ( 'NONE',  ( 0.000000000000000000, -0.1350103645451876666, -0.9908441862701600211 ) ) ;
#183417=VERTEX_POINT ( 'NONE', #84133 ) ;
#183443=CARTESIAN_POINT ( 'NONE',  ( -18.46093223321774701, -9.480682968274523503, -7.084550513926728854 ) ) ;
#183451=CARTESIAN_POINT ( 'NONE',  ( 18.42636655943171320, -9.496944315770630141, -40.10908057115552339 ) ) ;
#183488=DIRECTION ( 'NONE',  ( 0.000000000000000000, 0.000000000000000000, 1.000000000000000000 ) ) ;
#183499=DIRECTION ( 'NONE',  ( 0.000000000000000000, 0.000000000000000000, 1.000000000000000000 ) ) ;
#183568=DIRECTION ( 'NONE',  ( 1.000000000000000000, 0.000000000000000000, 0.000000000000000000 ) ) ;
#183577=EDGE_LOOP ( 'NONE', ( #230131, #103054, #67105, #113896 ) ) ;
#183581=AXIS2_PLACEMENT_3D ( 'NONE', #206381, #246772, #29062 ) ;
#183637=ORIENTED_EDGE ( 'NONE', *, *, #180779, .F. ) ;
#183642=CIRCLE ( 'NONE', #104493, 11.75000000000000000 ) ;
#183647=CARTESIAN_POINT ( 'NONE',  ( 22.39999999999999858, 7.790779598373383408, 0.09999999999999939493 ) ) ;
#183651=ORIENTED_EDGE ( 'NONE', *, *, #92395, .T. ) ;
#183659=EDGE_CURVE ( 'NONE', #217291, #79953, #184019, .T. ) ;
#183684=CARTESIAN_POINT ( 'NONE',  ( 18.59999999999999076, 6.550000000000000711, -21.25000000000000000 ) ) ;
#183696=DIRECTION ( 'NONE',  ( -0.000000000000000000, -0.1350103645451904977, 0.9908441862701596881 ) ) ;
#183704=AXIS2_PLACEMENT_3D ( 'NONE', #235398, #195023, #252386 ) ;
#183711=EDGE_CURVE ( 'NONE', #16494, #55133, #5103, .T. ) ;
#183737=ORIENTED_EDGE ( 'NONE', *, *, #125305, .F. ) ;
#183769=EDGE_CURVE ( 'NONE', #180654, #143742, #7847, .T. ) ;
#183775=ORIENTED_EDGE ( 'NONE', *, *, #86680, .T. ) ;
#183800=CARTESIAN_POINT ( 'NONE',  ( -18.59999999999999787, 11.64999999999999680, -21.35000000000000142 ) ) ;
#183816=EDGE_LOOP ( 'NONE', ( #90915, #117366, #73393, #115779 ) ) ;
#183845=AXIS2_PLACEMENT_3D ( 'NONE', #100482, #180059, #256966 ) ;
#183873=TOROIDAL_SURFACE ( 'NONE', #221263, 3.899999999999999467, 0.1000000000000000056 ) ;
#183901=DIRECTION ( 'NONE',  ( 1.000000000000000000, 0.000000000000000000, 0.000000000000000000 ) ) ;
#183908=EDGE_LOOP ( 'NONE', ( #211194, #192123, #46693, #146991 ) ) ;
#183917=ORIENTED_EDGE ( 'NONE', *, *, #257764, .T. ) ;
#183929=ORIENTED_EDGE ( 'NONE', *, *, #61571, .F. ) ;
#183931=EDGE_LOOP ( 'NONE', ( #70188, #201472 ) ) ;
#183935=ORIENTED_EDGE ( 'NONE', *, *, #85126, .F. ) ;
#183942=DIRECTION ( 'NONE',  ( 0.000000000000000000, 0.000000000000000000, -1.000000000000000000 ) ) ;
#183956=EDGE_CURVE ( 'NONE', #251409, #17057, #221592, .T. ) ;
#183968=CARTESIAN_POINT ( 'NONE',  ( -23.15000000000000213, -11.39257802170566691, -30.42605042016806394 ) ) ;
#183975=AXIS2_PLACEMENT_3D ( 'NONE', #12830, #33701, #113188 ) ;
#183984=CARTESIAN_POINT ( 'NONE',  ( 20.85000000000000142, -1.835859311443637010, -45.00443916879852679 ) ) ;
#184019=CIRCLE ( 'NONE', #183845, 0.09999999999999939493 ) ;
#184043=DIRECTION ( 'NONE',  ( 0.000000000000000000, 0.000000000000000000, 1.000000000000000000 ) ) ;
#184065=CARTESIAN_POINT ( 'NONE',  ( 23.24999999999999289, 11.65000000000000746, 0.000000000000000000 ) ) ;
#184097=DIRECTION ( 'NONE',  ( 0.000000000000000000, 0.000000000000000000, -1.000000000000000000 ) ) ;
#184108=CARTESIAN_POINT ( 'NONE',  ( -20.93302460841142931, 10.31565961586829872, -39.03641941191782649 ) ) ;
#184115=ORIENTED_EDGE ( 'NONE', *, *, #54576, .T. ) ;
#184122=EDGE_CURVE ( 'NONE', #116070, #164389, #175920, .T. ) ;
#184169=EDGE_CURVE ( 'NONE', #162626, #250243, #159286, .T. ) ;
#184180=VERTEX_POINT ( 'NONE', #206681 ) ;
#184187=EDGE_LOOP ( 'NONE', ( #5287, #123454, #86361, #221984 ) ) ;
#184228=VECTOR ( 'NONE', #256700, 1000.000000000000000 ) ;
#184241=DIRECTION ( 'NONE',  ( 0.000000000000000000, 0.000000000000000000, 1.000000000000000000 ) ) ;
#184244=DIRECTION ( 'NONE',  ( 1.000000000000000000, 0.000000000000000000, 0.000000000000000000 ) ) ;
#184293=FACE_OUTER_BOUND ( 'NONE', #18844, .T. ) ;
#184324=AXIS2_PLACEMENT_3D ( 'NONE', #190380, #166014, #151247 ) ;
#184332=VECTOR ( 'NONE', #53607, 1000.000000000000000 ) ;
#184334=CARTESIAN_POINT ( 'NONE',  ( -23.15000000000000213, 11.75000000000000000, -12.15000000000000036 ) ) ;
#184337=CIRCLE ( 'NONE', #155175, 3.999999999999996447 ) ;
#184339=VECTOR ( 'NONE', #6720, 1000.000000000000000 ) ;
#184355=CARTESIAN_POINT ( 'NONE',  ( 20.04142135623730070, 11.65000000000000391, -21.35000000000000142 ) ) ;
#184356=EDGE_CURVE ( 'NONE', #118795, #165206, #242644, .T. ) ;
#184357=DIRECTION ( 'NONE',  ( -0.000000000000000000, -0.2605042016806452532, -0.9654727137038777718 ) ) ;
#184376=EDGE_CURVE ( 'NONE', #116906, #242879, #117749, .T. ) ;
#184400=CARTESIAN_POINT ( 'NONE',  ( 23.15000000000000213, -9.000000000000000000, -23.60603087734755690 ) ) ;
#184418=ORIENTED_EDGE ( 'NONE', *, *, #160551, .F. ) ;
#184424=VECTOR ( 'NONE', #107366, 1000.000000000000000 ) ;
#184438=CARTESIAN_POINT ( 'NONE',  ( 18.55121869061587958, 10.32747123226657848, -39.07740328502492844 ) ) ;
#184452=CARTESIAN_POINT ( 'NONE',  ( -1.739115166359751801E-14, 11.64999999999998970, -24.85000000000000142 ) ) ;
#184498=AXIS2_PLACEMENT_3D ( 'NONE', #3290, #162407, #106242 ) ;
#184509=ORIENTED_EDGE ( 'NONE', *, *, #187956, .F. ) ;
#184534=EDGE_CURVE ( 'NONE', #227113, #225538, #159454, .T. ) ;
#184612=ORIENTED_EDGE ( 'NONE', *, *, #103425, .F. ) ;
#184617=ORIENTED_EDGE ( 'NONE', *, *, #173945, .F. ) ;
#184661=CARTESIAN_POINT ( 'NONE',  ( -20.94999999999999929, 0.000000000000000000, -33.50000000000000000 ) ) ;
#184671=EDGE_LOOP ( 'NONE', ( #41735, #3594, #126819, #22238 ) ) ;
#184678=AXIS2_PLACEMENT_3D ( 'NONE', #240132, #237559, #61489 ) ;
#184680=VERTEX_POINT ( 'NONE', #207678 ) ;
#184706=FACE_BOUND ( 'NONE', #203959, .T. ) ;
#184708=AXIS2_PLACEMENT_3D ( 'NONE', #223843, #63492, #100035 ) ;
#184717=FACE_OUTER_BOUND ( 'NONE', #204130, .T. ) ;
#184738=EDGE_CURVE ( 'NONE', #174426, #106998, #92793, .T. ) ;
#184761=FACE_OUTER_BOUND ( 'NONE', #179325, .T. ) ;
#184766=EDGE_CURVE ( 'NONE', #213112, #71518, #142840, .T. ) ;
#184781=AXIS2_PLACEMENT_3D ( 'NONE', #187083, #155674, #35723 ) ;
#184836=CIRCLE ( 'NONE', #189139, 0.09999999999999939493 ) ;
#184867=DIRECTION ( 'NONE',  ( 1.000000000000000000, -0.000000000000000000, -0.000000000000000000 ) ) ;
#184879=DIRECTION ( 'NONE',  ( 0.000000000000000000, 0.8660254037844383745, -0.5000000000000003331 ) ) ;
#184883=EDGE_LOOP ( 'NONE', ( #194577, #125664, #193924, #91636, #152345 ) ) ;
#184902=CIRCLE ( 'NONE', #168390, 0.09999999999999939493 ) ;
#184903=ADVANCED_FACE ( 'NONE', ( #159265 ), #201316, .F. ) ;
#184912=DIRECTION ( 'NONE',  ( 0.000000000000000000, 0.5000000000000004441, 0.8660254037844384856 ) ) ;
#184920=EDGE_LOOP ( 'NONE', ( #45838, #75158, #161695, #213047, #118924, #130978 ) ) ;
#184921=EDGE_CURVE ( 'NONE', #101735, #117327, #105614, .T. ) ;
#184931=VERTEX_POINT ( 'NONE', #120159 ) ;
#184937=VECTOR ( 'NONE', #78106, 1000.000000000000000 ) ;
#184938=PLANE ( 'NONE',  #221435 ) ;
#184939=LINE ( 'NONE', #67558, #28020 ) ;
#184979=EDGE_CURVE ( 'NONE', #172995, #28201, #55529, .T. ) ;
#184999=CIRCLE ( 'NONE', #147401, 7.800000000000001599 ) ;
#185005=CARTESIAN_POINT ( 'NONE',  ( 23.14999999999998437, 4.959819536546799335E-16, 4.049999999999998934 ) ) ;
#185028=CARTESIAN_POINT ( 'NONE',  ( 22.47071067811865319, 7.720074744498043984, 0.09909245470260480415 ) ) ;
#185047=EDGE_CURVE ( 'NONE', #63983, #83974, #13883, .T. ) ;
#185054=VERTEX_POINT ( 'NONE', #186524 ) ;
#185056=VERTEX_POINT ( 'NONE', #7896 ) ;
#185094=EDGE_CURVE ( 'NONE', #18698, #201752, #53422, .T. ) ;
#185139=CIRCLE ( 'NONE', #164305, 0.1000000000000002554 ) ;
#185191=DIRECTION ( 'NONE',  ( -1.000000000000000000, 0.000000000000000000, 0.000000000000000000 ) ) ;
#185196=CARTESIAN_POINT ( 'NONE',  ( -20.54999999999999716, 0.000000000000000000, 0.000000000000000000 ) ) ;
#185205=ORIENTED_EDGE ( 'NONE', *, *, #123407, .F. ) ;
#185215=EDGE_CURVE ( 'NONE', #47350, #36387, #218224, .T. ) ;
#185221=EDGE_CURVE ( 'NONE', #207337, #64464, #239768, .T. ) ;
#185251=CYLINDRICAL_SURFACE ( 'NONE', #236260, 0.09999999999999939493 ) ;
#185254=DIRECTION ( 'NONE',  ( 1.000000000000000000, 0.000000000000000000, 0.000000000000000000 ) ) ;
#185276=CARTESIAN_POINT ( 'NONE',  ( -20.54999999999999716, 7.249999999999999112, -12.25000000000000000 ) ) ;
#185279=CARTESIAN_POINT ( 'NONE',  ( -21.04999999999999716, 6.440770893661913910, -0.01759718700864921007 ) ) ;
#185298=AXIS2_PLACEMENT_3D ( 'NONE', #216223, #167844, #226479 ) ;
#185346=ORIENTED_EDGE ( 'NONE', *, *, #131304, .F. ) ;
#185385=FACE_OUTER_BOUND ( 'NONE', #234101, .T. ) ;
#185399=EDGE_CURVE ( 'NONE', #9216, #31326, #101510, .T. ) ;
#185451=ORIENTED_EDGE ( 'NONE', *, *, #74646, .T. ) ;
#185457=CIRCLE ( 'NONE', #222855, 0.6000000000000015321 ) ;
#185459=ORIENTED_EDGE ( 'NONE', *, *, #3402, .F. ) ;
#185464=CARTESIAN_POINT ( 'NONE',  ( -18.39999999999999858, -9.600000000000003197, -40.20018939122204671 ) ) ;
#185465=EDGE_CURVE ( 'NONE', #233652, #209763, #30835, .T. ) ;
#185478=VERTEX_POINT ( 'NONE', #170552 ) ;
#185532=ORIENTED_EDGE ( 'NONE', *, *, #64920, .F. ) ;
#185560=MECHANICAL_DESIGN_GEOMETRIC_PRESENTATION_REPRESENTATION('',(#202141),#60459);
#185573=CARTESIAN_POINT ( 'NONE',  ( 23.14999999999999858, 5.950000000000003730, -23.19429769496518645 ) ) ;
#185576=DIRECTION ( 'NONE',  ( 0.000000000000000000, 0.000000000000000000, 1.000000000000000000 ) ) ;
#185605=DIRECTION ( 'NONE',  ( 1.000000000000000000, 0.000000000000000000, 0.000000000000000000 ) ) ;
#185633=VECTOR ( 'NONE', #43271, 1000.000000000000000 ) ;
#185660=FACE_OUTER_BOUND ( 'NONE', #201075, .T. ) ;
#185686=ADVANCED_FACE ( 'NONE', ( #101174 ), #201687, .F. ) ;
#185701=CARTESIAN_POINT ( 'NONE',  ( -20.64999999999999858, 0.000000000000000000, -33.50000000000000000 ) ) ;
#185707=DIRECTION ( 'NONE',  ( -1.000000000000000000, 0.000000000000000000, 0.000000000000000000 ) ) ;
#185709=EDGE_LOOP ( 'NONE', ( #75806, #160270, #38874 ) ) ;
#185719=CIRCLE ( 'NONE', #48344, 0.09999999999999892308 ) ;
#185723=FACE_OUTER_BOUND ( 'NONE', #201148, .T. ) ;
#185730=ADVANCED_FACE ( 'NONE', ( #115657 ), #243378, .F. ) ;
#185736=VERTEX_POINT ( 'NONE', #80344 ) ;
#185764=CIRCLE ( 'NONE', #123226, 0.09999999999999939493 ) ;
#185800=ORIENTED_EDGE ( 'NONE', *, *, #31943, .F. ) ;
#185810=CYLINDRICAL_SURFACE ( 'NONE', #36534, 7.900000000000003908 ) ;
#185812=CARTESIAN_POINT ( 'NONE',  ( 20.94999999999999929, -9.000000000000000000, -23.60603087734755690 ) ) ;
#185826=ADVANCED_FACE ( 'NONE', ( #26853 ), #89244, .T. ) ;
#185835=CYLINDRICAL_SURFACE ( 'NONE', #73555, 0.09999999999999939493 ) ;
#185837=DIRECTION ( 'NONE',  ( 0.000000000000000000, 0.000000000000000000, -1.000000000000000000 ) ) ;
#185892=ORIENTED_EDGE ( 'NONE', *, *, #97123, .F. ) ;
#185900=EDGE_CURVE ( 'NONE', #118795, #198340, #5950, .T. ) ;
#185915=LINE ( 'NONE', #67251, #78499 ) ;
#185931=DIRECTION ( 'NONE',  ( 0.000000000000000000, -0.4999999999999836242, 0.8660254037844480335 ) ) ;
#185937=FACE_OUTER_BOUND ( 'NONE', #56529, .T. ) ;
#185949=CARTESIAN_POINT ( 'NONE',  ( 21.14999999999999503, 0.000000000000000000, 6.249999999999998224 ) ) ;
#185964=CARTESIAN_POINT ( 'NONE',  ( 23.14999999999999858, 0.000000000000000000, -33.50000000000000000 ) ) ;
#185994=EDGE_CURVE ( 'NONE', #120640, #213598, #17228, .T. ) ;
#186008=CARTESIAN_POINT ( 'NONE',  ( 18.49999999999999645, -9.419078080849526913, -40.32992535020828484 ) ) ;
#186009=DIRECTION ( 'NONE',  ( 2.952720810173289112E-16, -1.000000000000000000, 0.000000000000000000 ) ) ;
#186025=VECTOR ( 'NONE', #241690, 1000.000000000000000 ) ;
#186036=CARTESIAN_POINT ( 'NONE',  ( 21.05000000000000071, 0.09779029130922507751, 6.257814610481526429 ) ) ;
#186044=DIRECTION ( 'NONE',  ( 1.000000000000000000, 0.000000000000000000, 0.000000000000000000 ) ) ;
#186072=TOROIDAL_SURFACE ( 'NONE', #131906, 0.2000000000000000111, 0.1000000000000000056 ) ;
#186130=EDGE_LOOP ( 'NONE', ( #46168, #137081, #72741, #8818 ) ) ;
#186160=EDGE_CURVE ( 'NONE', #209135, #187669, #61476, .T. ) ;
#186168=FACE_OUTER_BOUND ( 'NONE', #239332, .T. ) ;
#186183=ORIENTED_EDGE ( 'NONE', *, *, #565, .T. ) ;
#186187=DIRECTION ( 'NONE',  ( 1.000000000000000000, 0.000000000000000000, -0.000000000000000000 ) ) ;
#186188=VERTEX_POINT ( 'NONE', #182722 ) ;
#186232=LINE ( 'NONE', #246201, #17450 ) ;
#186246=DIRECTION ( 'NONE',  ( 0.000000000000000000, 0.000000000000000000, -1.000000000000000000 ) ) ;
#186251=ADVANCED_FACE ( 'NONE', ( #108311 ), #206122, .T. ) ;
#186264=DIRECTION ( 'NONE',  ( 0.000000000000000000, 0.9908441862701596881, 0.1350103645451904977 ) ) ;
#186290=DIRECTION ( 'NONE',  ( 0.000000000000000000, 0.000000000000000000, 1.000000000000000000 ) ) ;
#186352=CIRCLE ( 'NONE', #115593, 0.1000000000000000472 ) ;
#186387=DIRECTION ( 'NONE',  ( -1.000000000000000000, -0.000000000000000000, -0.000000000000000000 ) ) ;
#186391=DIRECTION ( 'NONE',  ( 0.000000000000000000, -0.9915357197604882655, 0.1298341882519793711 ) ) ;
#186404=CARTESIAN_POINT ( 'NONE',  ( 19.80993210785512204, 11.74999999999953104, -24.76711774888639184 ) ) ;
#186409=EDGE_LOOP ( 'NONE', ( #50744, #240073, #81739, #118129 ) ) ;
#186427=CARTESIAN_POINT ( 'NONE',  ( -23.15000000000000213, 11.75000000000000000, -30.39999999999999858 ) ) ;
#186432=CARTESIAN_POINT ( 'NONE',  ( -22.49999999999999645, 11.74956712348939014, 0.1008583690987081283 ) ) ;
#186453=ORIENTED_EDGE ( 'NONE', *, *, #192819, .T. ) ;
#186468=CARTESIAN_POINT ( 'NONE',  ( -23.25000000000000000, -11.75000000000000000, -3.100000000000001865 ) ) ;
#186479=CARTESIAN_POINT ( 'NONE',  ( 23.15000000000000213, -12.41227409414968363, -30.39999999999999503 ) ) ;
#186481=( BOUNDED_SURFACE ( )  B_SPLINE_SURFACE ( 3, 2, ( 
 ( #109915, #167365, #227301 ),
 ( #229881, #189475, #224724 ),
 ( #246858, #245595, #206461 ),
 ( #66947, #149076, #46090 ),
 ( #186927, #126929, #209031 ),
 ( #147783, #111214, #106048 ) ),
 .UNSPECIFIED., .F., .F., .F. ) 
 B_SPLINE_SURFACE_WITH_KNOTS ( ( 4, 2, 4 ),
 ( 3, 3 ),
 ( -1.776356839400250465E-15, 0.7853981633974468357, 1.570796326794895448 ),
 ( 0.000000000000000000, 1.000000000000000000 ),
 .UNSPECIFIED. ) 
 GEOMETRIC_REPRESENTATION_ITEM ( )  RATIONAL_B_SPLINE_SURFACE ( (
 ( 1.000000000000000000, 0.5000000000000101030, 1.000000000000000000),
 ( 1.000000000000000000, 0.4993418825328820865, 1.000000000000000000),
 ( 1.000000000000000000, 0.5278258667065299781, 1.000000000000000000),
 ( 1.000000000000000000, 0.6092287576688560913, 1.000000000000000000),
 ( 1.000000000000000000, 0.6611148371784629774, 1.000000000000000000),
 ( 1.000000000000000000, 0.7071067811865658914, 1.000000000000000000) ) ) 
 REPRESENTATION_ITEM ( '' )  SURFACE ( )  );
#186497=( BOUNDED_SURFACE ( )  B_SPLINE_SURFACE ( 3, 2, ( 
 ( #147416, #7922, #11788 ),
 ( #249104, #71750, #150010 ),
 ( #165718, #229532, #146125 ),
 ( #108298, #129142, #148715 ),
 ( #87427, #67874, #131706 ),
 ( #50854, #126573, #211244 ) ),
 .UNSPECIFIED., .F., .F., .F. ) 
 B_SPLINE_SURFACE_WITH_KNOTS ( ( 4, 2, 4 ),
 ( 3, 3 ),
 ( 0.0001792624049599548033, 0.0003686986002124708565, 0.0005581347954649869096 ),
 ( 0.000000000000000000, 1.000000000000000000 ),
 .UNSPECIFIED. ) 
 GEOMETRIC_REPRESENTATION_ITEM ( )  RATIONAL_B_SPLINE_SURFACE ( (
 ( 1.000000000000000000, 0.9238795325112848511, 1.000000000000000000),
 ( 1.000000000000000000, 0.9229318695238726278, 1.000000000000000000),
 ( 1.000000000000000000, 0.8926288119230381124, 1.000000000000000000),
 ( 1.000000000000000000, 0.8123777807271690410, 1.000000000000000000),
 ( 1.000000000000000000, 0.7629087100931283283, 1.000000000000000000),
 ( 1.000000000000000000, 0.7071067811865475727, 1.000000000000000000) ) ) 
 REPRESENTATION_ITEM ( '' )  SURFACE ( )  );
#186520=DIRECTION ( 'NONE',  ( 0.000000000000000000, -1.000000000000000000, 0.000000000000000000 ) ) ;
#186522=DIRECTION ( 'NONE',  ( 0.000000000000000000, 0.000000000000000000, -1.000000000000000000 ) ) ;
#186523=ORIENTED_EDGE ( 'NONE', *, *, #16135, .T. ) ;
#186524=CARTESIAN_POINT ( 'NONE',  ( -20.64999999999999858, 0.000000000000000000, -20.62500000000000355 ) ) ;
#186550=DIRECTION ( 'NONE',  ( 1.000000000000000000, -0.000000000000000000, -0.000000000000000000 ) ) ;
#186575=CARTESIAN_POINT ( 'NONE',  ( -21.05000000000000071, 1.162701749938009677, -8.000000000000000000 ) ) ;
#186643=DIRECTION ( 'NONE',  ( -0.000000000000000000, 0.000000000000000000, 1.000000000000000000 ) ) ;
#186675=CARTESIAN_POINT ( 'NONE',  ( 19.88284271247461987, 11.69142135623731704, -24.75000000000000000 ) ) ;
#186727=CARTESIAN_POINT ( 'NONE',  ( 18.49999999999999289, 6.649999999999999467, -21.15000000000000213 ) ) ;
#186733=TOROIDAL_SURFACE ( 'NONE', #178356, 0.2000000000000000111, 0.1000000000000000056 ) ;
#186775=EDGE_CURVE ( 'NONE', #96700, #203969, #240318, .T. ) ;
#186788=CIRCLE ( 'NONE', #74382, 0.09999999999999939493 ) ;
#186790=EDGE_CURVE ( 'NONE', #56536, #239317, #113131, .T. ) ;
#186869=CYLINDRICAL_SURFACE ( 'NONE', #33215, 4.000000000000000000 ) ;
#186879=CARTESIAN_POINT ( 'NONE',  ( 21.05000000000000071, 1.162701749938009677, -8.099999999999999645 ) ) ;
#186886=CARTESIAN_POINT ( 'NONE',  ( 20.94999999999999929, 4.813084112149527805, -21.55848224347618114 ) ) ;
#186892=DIRECTION ( 'NONE',  ( 0.000000000000000000, 0.000000000000000000, -1.000000000000000000 ) ) ;
#186927=CARTESIAN_POINT ( 'NONE',  ( 20.94999999999999929, 11.63687328910416952, -26.67824078667522159 ) ) ;
#186963=ORIENTED_EDGE ( 'NONE', *, *, #229436, .F. ) ;
#186979=CIRCLE ( 'NONE', #211902, 12.97499999999999964 ) ;
#187004=DIRECTION ( 'NONE',  ( 0.000000000000000000, -1.000000000000000000, 0.000000000000000000 ) ) ;
#187024=CARTESIAN_POINT ( 'NONE',  ( 23.14999999999999858, 0.000000000000000000, -33.50000000000000000 ) ) ;
#187036=CIRCLE ( 'NONE', #82915, 0.5000000000000022204 ) ;
#187045=ADVANCED_FACE ( 'NONE', ( #185937 ), #123402, .F. ) ;
#187059=AXIS2_PLACEMENT_3D ( 'NONE', #198008, #136748, #200585 ) ;
#187071=EDGE_CURVE ( 'NONE', #29061, #184680, #140338, .T. ) ;
#187076=VERTEX_POINT ( 'NONE', #204209 ) ;
#187079=ORIENTED_EDGE ( 'NONE', *, *, #33485, .T. ) ;
#187083=CARTESIAN_POINT ( 'NONE',  ( 21.00000000000000000, 9.749999999999998224, -21.15000000000000213 ) ) ;
#187105=FACE_OUTER_BOUND ( 'NONE', #27269, .T. ) ;
#187130=DIRECTION ( 'NONE',  ( -1.000000000000000000, 0.000000000000000000, 0.000000000000000000 ) ) ;
#187147=EDGE_CURVE ( 'NONE', #155798, #169470, #99504, .T. ) ;
#187149=DIRECTION ( 'NONE',  ( -1.000000000000000000, 0.000000000000000000, 0.000000000000000000 ) ) ;
#187176=CARTESIAN_POINT ( 'NONE',  ( -21.05000000000000071, 1.749999999999999778, -11.66951155790164307 ) ) ;
#187178=ORIENTED_EDGE ( 'NONE', *, *, #108515, .T. ) ;
#187187=VECTOR ( 'NONE', #209950, 1000.000000000000000 ) ;
#187192=DIRECTION ( 'NONE',  ( 2.952720810173289112E-16, -1.000000000000000000, -0.000000000000000000 ) ) ;
#187195=ADVANCED_FACE ( 'NONE', ( #197338 ), #252085, .T. ) ;
#187222=FACE_OUTER_BOUND ( 'NONE', #236327, .T. ) ;
#187224=FACE_OUTER_BOUND ( 'NONE', #156680, .T. ) ;
#187232=EDGE_LOOP ( 'NONE', ( #94357, #237283, #145082, #69864 ) ) ;
#187257=CARTESIAN_POINT ( 'NONE',  ( 20.93975676684922504, 10.31104185822947450, -39.02045169831057336 ) ) ;
#187258=DIRECTION ( 'NONE',  ( -1.000000000000000000, -0.000000000000000000, -0.000000000000000000 ) ) ;
#187262=CIRCLE ( 'NONE', #254417, 0.09999999999999939493 ) ;
#187265=CARTESIAN_POINT ( 'NONE',  ( 21.05000000000000071, 8.776282889868772585, -12.17621514106822467 ) ) ;
#187294=CARTESIAN_POINT ( 'NONE',  ( 21.05000000000000071, -8.730841121495320323, -23.90192528101566438 ) ) ;
#187309=EDGE_CURVE ( 'NONE', #13242, #202160, #160534, .T. ) ;
#187310=CARTESIAN_POINT ( 'NONE',  ( 23.14999999999999503, 11.65000000000000746, -26.48519422934606027 ) ) ;
#187317=ADVANCED_FACE ( 'NONE', ( #143786 ), #110615, .T. ) ;
#187366=DIRECTION ( 'NONE',  ( 1.000000000000000000, 1.836970198721029934E-16, 0.000000000000000000 ) ) ;
#187416=AXIS2_PLACEMENT_3D ( 'NONE', #203544, #164424, #104412 ) ;
#187431=ORIENTED_EDGE ( 'NONE', *, *, #70932, .F. ) ;
#187436=AXIS2_PLACEMENT_3D ( 'NONE', #137483, #235312, #56645 ) ;
#187457=AXIS2_PLACEMENT_3D ( 'NONE', #8232, #125593, #69502 ) ;
#187471=CARTESIAN_POINT ( 'NONE',  ( 18.39999999999999858, -9.599999999999997868, -7.032069396699667685 ) ) ;
#187483=DIRECTION ( 'NONE',  ( 0.000000000000000000, 0.000000000000000000, -1.000000000000000000 ) ) ;
#187501=CARTESIAN_POINT ( 'NONE',  ( 21.05000000000000071, 0.000000000000000000, 0.000000000000000000 ) ) ;
#187530=CARTESIAN_POINT ( 'NONE',  ( 21.14999999999999503, -11.64999999999999147, -2.900000000000003464 ) ) ;
#187541=ORIENTED_EDGE ( 'NONE', *, *, #77684, .F. ) ;
#187562=CYLINDRICAL_SURFACE ( 'NONE', #250437, 0.1000000000000028644 ) ;
#187590=EDGE_CURVE ( 'NONE', #105026, #80105, #138482, .T. ) ;
#187592=ORIENTED_EDGE ( 'NONE', *, *, #230181, .F. ) ;
#187603=CYLINDRICAL_SURFACE ( 'NONE', #158732, 0.09999999999999939493 ) ;
#187606=ORIENTED_EDGE ( 'NONE', *, *, #166967, .F. ) ;
#187621=LINE ( 'NONE', #6393, #65643 ) ;
#187623=ORIENTED_EDGE ( 'NONE', *, *, #83181, .T. ) ;
#187669=VERTEX_POINT ( 'NONE', #121555 ) ;
#187694=CARTESIAN_POINT ( 'NONE',  ( 19.87657994472027312, 11.74999999999995204, -24.76578812462619439 ) ) ;
#187716=CYLINDRICAL_SURFACE ( 'NONE', #202834, 0.09999999999999939493 ) ;
#187722=FACE_OUTER_BOUND ( 'NONE', #253822, .T. ) ;
#187725=ORIENTED_EDGE ( 'NONE', *, *, #101229, .T. ) ;
#187754=ORIENTED_EDGE ( 'NONE', *, *, #234752, .T. ) ;
#187765=EDGE_LOOP ( 'NONE', ( #221337, #27118, #29221, #108877 ) ) ;
#187781=ADVANCED_FACE ( 'NONE', ( #8004 ), #244020, .T. ) ;
#187790=LINE ( 'NONE', #106938, #60062 ) ;
#187838=ORIENTED_EDGE ( 'NONE', *, *, #52177, .T. ) ;
#187842=DIRECTION ( 'NONE',  ( 0.000000000000000000, 0.000000000000000000, -1.000000000000000000 ) ) ;
#187863=DIRECTION ( 'NONE',  ( 0.000000000000000000, -1.000000000000000000, -0.000000000000000000 ) ) ;
#187865=CARTESIAN_POINT ( 'NONE',  ( -21.05000000000000071, 6.540656951701244282, -0.09999999999999939493 ) ) ;
#187866=ORIENTED_EDGE ( 'NONE', *, *, #201903, .F. ) ;
#187877=ORIENTED_EDGE ( 'NONE', *, *, #16461, .T. ) ;
#187880=DIRECTION ( 'NONE',  ( -1.000000000000000000, 0.000000000000000000, 0.000000000000000000 ) ) ;
#187881=DIRECTION ( 'NONE',  ( 0.000000000000000000, -1.000000000000000000, 0.000000000000000000 ) ) ;
#187884=AXIS2_PLACEMENT_3D ( 'NONE', #141596, #20392, #219849 ) ;
#187888=CARTESIAN_POINT ( 'NONE',  ( 22.50000000000000000, 0.000000000000000000, 0.000000000000000000 ) ) ;
#187903=CARTESIAN_POINT ( 'NONE',  ( -21.05000000000000071, 1.835341550224413698, -11.55515129256298401 ) ) ;
#187933=FACE_OUTER_BOUND ( 'NONE', #204703, .T. ) ;
#187944=LINE ( 'NONE', #84943, #23516 ) ;
#187956=EDGE_CURVE ( 'NONE', #163426, #127360, #81717, .T. ) ;
#187967=TOROIDAL_SURFACE ( 'NONE', #117036, 11.65000000000000036, 0.1000000000000000056 ) ;
#187995=CIRCLE ( 'NONE', #212943, 0.09999999999999939493 ) ;
#188079=ORIENTED_EDGE ( 'NONE', *, *, #211233, .F. ) ;
#188106=VECTOR ( 'NONE', #231543, 1000.000000000000000 ) ;
#188115=ORIENTED_EDGE ( 'NONE', *, *, #87991, .T. ) ;
#188118=ORIENTED_EDGE ( 'NONE', *, *, #149373, .F. ) ;
#188128=EDGE_CURVE ( 'NONE', #243786, #20836, #202559, .T. ) ;
#188129=DIRECTION ( 'NONE',  ( -1.000000000000000000, -0.000000000000000000, -0.000000000000000000 ) ) ;
#188153=CIRCLE ( 'NONE', #34244, 0.6000000000000015321 ) ;
#188154=DIRECTION ( 'NONE',  ( 1.000000000000000000, 0.000000000000000000, 0.000000000000000000 ) ) ;
#188176=AXIS2_PLACEMENT_3D ( 'NONE', #253392, #53914, #57746 ) ;
#188185=DIRECTION ( 'NONE',  ( 0.000000000000000000, 1.000000000000000000, 0.000000000000000000 ) ) ;
#188205=ORIENTED_EDGE ( 'NONE', *, *, #172679, .T. ) ;
#188251=CARTESIAN_POINT ( 'NONE',  ( 18.49999999999998934, 6.649999999999999467, -12.35000000000000320 ) ) ;
#188252=CARTESIAN_POINT ( 'NONE',  ( 22.50497660315937409, -0.07871793022550384322, 11.74979550489544167 ) ) ;
#188306=CARTESIAN_POINT ( 'NONE',  ( -20.94999999999999929, -11.29603075033528192, -30.45210084033612929 ) ) ;
#188349=DIRECTION ( 'NONE',  ( 1.000000000000000000, 0.000000000000000000, -0.000000000000000000 ) ) ;
#188360=DIRECTION ( 'NONE',  ( 0.000000000000000000, 0.4999999999999799605, -0.8660254037844502539 ) ) ;
#188362=CARTESIAN_POINT ( 'NONE',  ( -20.85000000000000142, 11.75000000000000000, -33.50000000000000000 ) ) ;
#188415=DIRECTION ( 'NONE',  ( 1.000000000000000000, -0.000000000000000000, -0.000000000000000000 ) ) ;
#188419=CARTESIAN_POINT ( 'NONE',  ( -21.14999999999999858, 11.75000000000000000, -6.783865662978153743 ) ) ;
#188433=DIRECTION ( 'NONE',  ( 0.000000000000000000, 0.000000000000000000, -1.000000000000000000 ) ) ;
#188448=DIRECTION ( 'NONE',  ( 1.000000000000000000, -0.000000000000000000, -0.000000000000000000 ) ) ;
#188449=DIRECTION ( 'NONE',  ( 0.000000000000000000, 0.000000000000000000, -1.000000000000000000 ) ) ;
#188454=EDGE_CURVE ( 'NONE', #86491, #211613, #173589, .T. ) ;
#188470=ORIENTED_EDGE ( 'NONE', *, *, #32685, .T. ) ;
#188479=DIRECTION ( 'NONE',  ( -2.915501640297153790E-16, 1.000000000000000000, 0.000000000000000000 ) ) ;
#188562=CARTESIAN_POINT ( 'NONE',  ( -20.64999999999999858, 4.349999999999999645, -12.35000000000000142 ) ) ;
#188566=ORIENTED_EDGE ( 'NONE', *, *, #7213, .T. ) ;
#188570=DIRECTION ( 'NONE',  ( 1.000000000000000000, 0.000000000000000000, 0.000000000000000000 ) ) ;
#188611=EDGE_LOOP ( 'NONE', ( #186453, #135501, #27677, #147791 ) ) ;
#188630=DIRECTION ( 'NONE',  ( -1.000000000000000000, 0.000000000000000000, 0.000000000000000000 ) ) ;
#188634=ORIENTED_EDGE ( 'NONE', *, *, #125791, .T. ) ;
#188659=ORIENTED_EDGE ( 'NONE', *, *, #222745, .T. ) ;
#188675=VERTEX_POINT ( 'NONE', #237662 ) ;
#188705=DIRECTION ( 'NONE',  ( -1.000000000000000000, 0.000000000000000000, 0.000000000000000000 ) ) ;
#188713=CARTESIAN_POINT ( 'NONE',  ( -23.15000000000000213, 11.75000000000000000, 11.75000000000000000 ) ) ;
#188717=VECTOR ( 'NONE', #46604, 1000.000000000000000 ) ;
#188743=CARTESIAN_POINT ( 'NONE',  ( 23.14999999999998437, 4.049999999999998934, 5.021051876504146399E-16 ) ) ;
#188857=ADVANCED_FACE ( 'NONE', ( #189247 ), #252231, .T. ) ;
#188873=ORIENTED_EDGE ( 'NONE', *, *, #183118, .F. ) ;
#188890=CARTESIAN_POINT ( 'NONE',  ( -18.59999999999999787, 1.749999999999999778, -11.66951155790164307 ) ) ;
#188893=CARTESIAN_POINT ( 'NONE',  ( -18.41817142474038960, -9.498703066602091738, -40.10396548763700508 ) ) ;
#188903=ORIENTED_EDGE ( 'NONE', *, *, #243284, .F. ) ;
#188911=CIRCLE ( 'NONE', #5721, 3.899999999999999467 ) ;
#188931=CARTESIAN_POINT ( 'NONE',  ( 21.14999999999999858, -11.64999999999999147, 3.469446951953614189E-15 ) ) ;
#188939=ADVANCED_FACE ( 'NONE', ( #185385 ), #6745, .T. ) ;
#188955=DIRECTION ( 'NONE',  ( 0.000000000000000000, 0.000000000000000000, -1.000000000000000000 ) ) ;
#188959=CARTESIAN_POINT ( 'NONE',  ( 19.75857864376269291, 11.75000000000000711, -24.85000000000000142 ) ) ;
#188960=EDGE_CURVE ( 'NONE', #50839, #206018, #75722, .T. ) ;
#188984=CARTESIAN_POINT ( 'NONE',  ( 21.05000000000000071, 0.000000000000000000, 0.000000000000000000 ) ) ;
#189038=AXIS2_PLACEMENT_3D ( 'NONE', #256703, #98933, #238475 ) ;
#189041=DIRECTION ( 'NONE',  ( -1.000000000000000000, -0.000000000000000000, -0.000000000000000000 ) ) ;
#189048=AXIS2_PLACEMENT_3D ( 'NONE', #213455, #173102, #54383 ) ;
#189052=AXIS2_PLACEMENT_3D ( 'NONE', #89570, #29643, #229100 ) ;
#189064=CARTESIAN_POINT ( 'NONE',  ( 18.59999999999999432, -1.866714910057309273, -11.75267524628200633 ) ) ;
#189072=DIRECTION ( 'NONE',  ( -1.000000000000000000, 0.000000000000000000, 0.000000000000000000 ) ) ;
#189081=EDGE_CURVE ( 'NONE', #11322, #199652, #202541, .T. ) ;
#189094=CARTESIAN_POINT ( 'NONE',  ( -20.54999999999999716, 7.249999999999999112, -21.15000000000000213 ) ) ;
#189097=EDGE_CURVE ( 'NONE', #39052, #37010, #31707, .T. ) ;
#189098=VECTOR ( 'NONE', #14841, 1000.000000000000000 ) ;
#189129=ORIENTED_EDGE ( 'NONE', *, *, #19425, .F. ) ;
#189139=AXIS2_PLACEMENT_3D ( 'NONE', #129329, #52340, #207602 ) ;
#189155=EDGE_CURVE ( 'NONE', #232204, #59020, #223199, .T. ) ;
#189200=LINE ( 'NONE', #95224, #135862 ) ;
#189247=FACE_OUTER_BOUND ( 'NONE', #147530, .T. ) ;
#189274=EDGE_CURVE ( 'NONE', #107696, #49099, #60886, .T. ) ;
#189296=ORIENTED_EDGE ( 'NONE', *, *, #112499, .F. ) ;
#189314=FACE_OUTER_BOUND ( 'NONE', #111370, .T. ) ;
#189316=DIRECTION ( 'NONE',  ( 4.408576920032447355E-17, -0.1350103645451876666, -0.9908441862701600211 ) ) ;
#189328=COLOUR_RGB ( '', 0.09019608, 0.27058824, 0.51372549) ;
#189343=EDGE_LOOP ( 'NONE', ( #164754, #60316, #129141, #192342 ) ) ;
#189347=AXIS2_PLACEMENT_3D ( 'NONE', #173547, #95236, #174827 ) ;
#189394=CARTESIAN_POINT ( 'NONE',  ( -21.05000000000000071, -11.64999999999999858, -30.39999999999999503 ) ) ;
#189408=EDGE_CURVE ( 'NONE', #28201, #158172, #114530, .T. ) ;
#189435=DIRECTION ( 'NONE',  ( -1.000000000000000000, -0.000000000000000000, 0.000000000000000000 ) ) ;
#189436=DIRECTION ( 'NONE',  ( 0.000000000000000000, 0.000000000000000000, -1.000000000000000000 ) ) ;
#189475=CARTESIAN_POINT ( 'NONE',  ( 21.05315837374230981, 11.74999999956163244, -26.65835599938597866 ) ) ;
#189517=CARTESIAN_POINT ( 'NONE',  ( -18.59999999999999787, 11.64999999999999680, 11.75000000000000000 ) ) ;
#189547=CIRCLE ( 'NONE', #164604, 0.5000000000000013323 ) ;
#189551=DIRECTION ( 'NONE',  ( 0.000000000000000000, 0.9999631594459056361, -0.008583690987128059571 ) ) ;
#189570=ORIENTED_EDGE ( 'NONE', *, *, #61307, .F. ) ;
#189589=EDGE_LOOP ( 'NONE', ( #218407, #145714, #100245, #157029 ) ) ;
#189609=CARTESIAN_POINT ( 'NONE',  ( -21.37071067811865532, 8.070710678118656389, -21.25000000000000000 ) ) ;
#189610=ADVANCED_FACE ( 'NONE', ( #136638 ), #59653, .T. ) ;
#189623=CARTESIAN_POINT ( 'NONE',  ( -20.94999999999999929, -11.39257802170566869, -30.42605042016806394 ) ) ;
#189630=DIRECTION ( 'NONE',  ( -1.000000000000000000, 0.000000000000000000, 0.000000000000000000 ) ) ;
#189665=AXIS2_PLACEMENT_3D ( 'NONE', #133549, #31912, #52718 ) ;
#189690=ORIENTED_EDGE ( 'NONE', *, *, #173343, .T. ) ;
#189709=AXIS2_PLACEMENT_3D ( 'NONE', #165540, #11603, #109383 ) ;
#189712=DIRECTION ( 'NONE',  ( -0.000000000000000000, -1.000000000000000000, 0.000000000000000000 ) ) ;
#189714=CARTESIAN_POINT ( 'NONE',  ( 20.94999999999999929, 11.65000000000000391, -26.65839931010294706 ) ) ;
#189748=ORIENTED_EDGE ( 'NONE', *, *, #138023, .F. ) ;
#189796=AXIS2_PLACEMENT_3D ( 'NONE', #125208, #204718, #67787 ) ;
#189807=TOROIDAL_SURFACE ( 'NONE', #77352, 12.77500000000000036, 0.1000000000000000056 ) ;
#189811=CARTESIAN_POINT ( 'NONE',  ( 20.89878130938411616, 10.32747123226657493, -39.07740328502492844 ) ) ;
#189826=DIRECTION ( 'NONE',  ( 0.000000000000000000, -0.000000000000000000, 1.000000000000000000 ) ) ;
#189828=AXIS2_PLACEMENT_3D ( 'NONE', #129453, #208984, #30369 ) ;
#189848=CARTESIAN_POINT ( 'NONE',  ( 21.04999999999963478, 10.62950747926064032, -7.627979399996550391 ) ) ;
#189850=DIRECTION ( 'NONE',  ( 0.000000000000000000, -1.000000000000000000, 0.000000000000000000 ) ) ;
#189902=DIRECTION ( 'NONE',  ( -1.000000000000000000, -0.000000000000000000, -0.000000000000000000 ) ) ;
#189937=CIRCLE ( 'NONE', #231642, 0.2000000000000005107 ) ;
#189945=CARTESIAN_POINT ( 'NONE',  ( -20.64999999999999858, 4.349999999999999645, -12.35000000000000142 ) ) ;
#190041=DIRECTION ( 'NONE',  ( 0.000000000000000000, 0.000000000000000000, -1.000000000000000000 ) ) ;
#190054=CARTESIAN_POINT ( 'NONE',  ( 20.94999999999999929, 14.05000000000000071, -27.98630492923908619 ) ) ;
#190059=DIRECTION ( 'NONE',  ( -0.000000000000000000, -0.000000000000000000, 1.000000000000000000 ) ) ;
#190063=ORIENTED_EDGE ( 'NONE', *, *, #49348, .F. ) ;
#190084=CARTESIAN_POINT ( 'NONE',  ( 21.07199075132371746, 8.774944999116087274, -12.21353216161286426 ) ) ;
#190140=ORIENTED_EDGE ( 'NONE', *, *, #178011, .F. ) ;
#190187=ADVANCED_FACE ( 'NONE', ( #116176 ), #86350, .T. ) ;
#190212=FACE_OUTER_BOUND ( 'NONE', #150973, .T. ) ;
#190230=SPHERICAL_SURFACE ( 'NONE', #189709, 0.1000000000000000056 ) ;
#190231=VECTOR ( 'NONE', #95498, 1000.000000000000000 ) ;
#190238=AXIS2_PLACEMENT_3D ( 'NONE', #114148, #172894, #252360 ) ;
#190247=CARTESIAN_POINT ( 'NONE',  ( 18.41815437325346849, -9.498709853141427573, -40.10394583880211172 ) ) ;
#190282=( BOUNDED_SURFACE ( )  B_SPLINE_SURFACE ( 3, 2, ( 
 ( #216182, #77956, #153720 ),
 ( #37580, #237048, #234468 ),
 ( #97501, #14179, #157555 ),
 ( #137927, #217461, #38861 ),
 ( #191537, #16734, #12896 ),
 ( #231935, #92391, #35038 ),
 ( #171985, #251469, #114538 ),
 ( #72877, #53284, #54554 ) ),
 .UNSPECIFIED., .F., .F., .F. ) 
 B_SPLINE_SURFACE_WITH_KNOTS ( ( 4, 2, 2, 4 ),
 ( 3, 3 ),
 ( 0.0001704874539069866865, 0.0003809798300636611833, 0.0004862260181419984588, 0.0005914722062203357344 ),
 ( 0.000000000000000000, 1.000000000000000000 ),
 .UNSPECIFIED. ) 
 GEOMETRIC_REPRESENTATION_ITEM ( )  RATIONAL_B_SPLINE_SURFACE ( (
 ( 1.000000000000000000, 0.7071067811864942820, 1.000000000000000000),
 ( 1.000000000000000000, 0.7670648383578079210, 1.000000000000000000),
 ( 1.000000000000000000, 0.8204820770250040862, 1.000000000000000000),
 ( 1.000000000000000000, 0.8877218296114878227, 1.000000000000000000),
 ( 1.000000000000000000, 0.9080815932665453616, 1.000000000000000000),
 ( 1.000000000000000000, 0.9395541505861941811, 1.000000000000000000),
 ( 1.000000000000000000, 0.9506520335378926267, 1.000000000000000000),
 ( 1.000000000000000000, 0.9504532311154582080, 1.000000000000000000) ) ) 
 REPRESENTATION_ITEM ( '' )  SURFACE ( )  );
#190304=ORIENTED_EDGE ( 'NONE', *, *, #117126, .F. ) ;
#190309=VERTEX_POINT ( 'NONE', #199577 ) ;
#190312=CARTESIAN_POINT ( 'NONE',  ( -20.94999999999999929, -1.736257131597395809, -11.56865232901749785 ) ) ;
#190332=EDGE_LOOP ( 'NONE', ( #145144, #257029, #82212 ) ) ;
#190380=CARTESIAN_POINT ( 'NONE',  ( -20.94999999999999929, 0.000000000000000000, -33.50000000000000000 ) ) ;
#190404=ORIENTED_EDGE ( 'NONE', *, *, #34187, .T. ) ;
#190408=LINE ( 'NONE', #84826, #99042 ) ;
#190469=AXIS2_PLACEMENT_3D ( 'NONE', #131652, #33887, #213754 ) ;
#190538=LINE ( 'NONE', #232229, #37424 ) ;
#190539=CARTESIAN_POINT ( 'NONE',  ( 23.14999999999999858, 5.599999999999996980, -21.09473398108690390 ) ) ;
#190545=ORIENTED_EDGE ( 'NONE', *, *, #75821, .T. ) ;
#190559=LINE ( 'NONE', #150148, #55688 ) ;
#190560=VECTOR ( 'NONE', #130462, 1000.000000000000000 ) ;
#190575=DIRECTION ( 'NONE',  ( 0.000000000000000000, 1.000000000000000000, 0.000000000000000000 ) ) ;
#190581=DIRECTION ( 'NONE',  ( -4.701977403289178058E-30, 1.734723475976807094E-14, -1.000000000000000000 ) ) ;
#190628=ORIENTED_EDGE ( 'NONE', *, *, #108995, .T. ) ;
#190684=ORIENTED_EDGE ( 'NONE', *, *, #65882, .T. ) ;
#190746=ORIENTED_EDGE ( 'NONE', *, *, #69986, .T. ) ;
#190749=SPHERICAL_SURFACE ( 'NONE', #107559, 0.1000000000000000056 ) ;
#190760=ADVANCED_FACE ( 'NONE', ( #246075 ), #186733, .T. ) ;
#190762=ORIENTED_EDGE ( 'NONE', *, *, #107088, .F. ) ;
#190768=ORIENTED_EDGE ( 'NONE', *, *, #218835, .F. ) ;
#190771=ORIENTED_EDGE ( 'NONE', *, *, #21758, .F. ) ;
#190790=CARTESIAN_POINT ( 'NONE',  ( -20.54999999999999716, -9.400000000000003908, -9.893969122652444881 ) ) ;
#190817=LINE ( 'NONE', #250744, #32554 ) ;
#190952=AXIS2_PLACEMENT_3D ( 'NONE', #174370, #197726, #135174 ) ;
#190971=ORIENTED_EDGE ( 'NONE', *, *, #54179, .T. ) ;
#190985=( NAMED_UNIT ( * ) SI_UNIT ( $, .STERADIAN. ) SOLID_ANGLE_UNIT ( ) );
#190990=CIRCLE ( 'NONE', #32794, 0.09999999999999939493 ) ;
#191019=EDGE_LOOP ( 'NONE', ( #10723, #71800, #130097, #177915 ) ) ;
#191045=DIRECTION ( 'NONE',  ( 0.000000000000000000, 0.000000000000000000, 1.000000000000000000 ) ) ;
#191070=VERTEX_POINT ( 'NONE', #120149 ) ;
#191075=CARTESIAN_POINT ( 'NONE',  ( -20.85000000000000142, 11.74999999999999645, -26.71613433702190576 ) ) ;
#191078=CARTESIAN_POINT ( 'NONE',  ( 18.49999999999999645, 0.000000000000000000, 0.000000000000000000 ) ) ;
#191120=CARTESIAN_POINT ( 'NONE',  ( -18.59999999999999787, 11.74999999999999645, -7.014805770653998351 ) ) ;
#191125=CARTESIAN_POINT ( 'NONE',  ( 21.04105312098496583, 8.875332623043611591, -12.32850674721203355 ) ) ;
#191147=LINE ( 'NONE', #72477, #207872 ) ;
#191196=EDGE_CURVE ( 'NONE', #18698, #178738, #224487, .T. ) ;
#191197=FACE_OUTER_BOUND ( 'NONE', #76852, .T. ) ;
#191203=UNCERTAINTY_MEASURE_WITH_UNIT (LENGTH_MEASURE( 1.000000000000000082E-05 ), #133583, 'distance_accuracy_value', 'NONE');
#191228=AXIS2_PLACEMENT_3D ( 'NONE', #172203, #251684, #15674 ) ;
#191237=CYLINDRICAL_SURFACE ( 'NONE', #63536, 0.09999999999999939493 ) ;
#191295=DIRECTION ( 'NONE',  ( -0.000000000000000000, -0.000000000000000000, -1.000000000000000000 ) ) ;
#191298=EDGE_CURVE ( 'NONE', #158172, #253517, #199389, .T. ) ;
#191314=AXIS2_PLACEMENT_3D ( 'NONE', #110450, #87012, #11362 ) ;
#191337=EDGE_LOOP ( 'NONE', ( #245925, #254685, #140372, #232447 ) ) ;
#191344=B_SPLINE_CURVE_WITH_KNOTS ( 'NONE', 3,
 ( #24813, #5182, #41801, #84707, #65181, #121352, #22230, #61340, #164301, #198275 ),
 .UNSPECIFIED., .F., .F.,
 ( 4, 3, 3, 4 ),
 ( 1.734723475976807094E-18, 0.0002000000000008561227, 0.001000000000082977483, 0.001967863649483316338 ),
 .UNSPECIFIED. ) ;
#191355=VERTEX_POINT ( 'NONE', #251610 ) ;
#191373=EDGE_LOOP ( 'NONE', ( #175008, #37387, #222761 ) ) ;
#191420=CARTESIAN_POINT ( 'NONE',  ( -21.04999999999999716, -9.600000000000001421, -7.032069396699667685 ) ) ;
#191428=CARTESIAN_POINT ( 'NONE',  ( -21.05000000000000071, -11.65000000000000036, -3.000000000000002665 ) ) ;
#191445=CARTESIAN_POINT ( 'NONE',  ( -23.15000000000000213, -9.500000000000003553, -9.893969122652444881 ) ) ;
#191476=CYLINDRICAL_SURFACE ( 'NONE', #183975, 4.049999999999998934 ) ;
#191478=FACE_OUTER_BOUND ( 'NONE', #96466, .T. ) ;
#191537=CARTESIAN_POINT ( 'NONE',  ( 18.46082813847998594, -9.480749650907464243, -7.084370102715693562 ) ) ;
#191608=CARTESIAN_POINT ( 'NONE',  ( -20.94999999999999929, -1.362429037193305881, -41.38888124792119783 ) ) ;
#191620=ORIENTED_EDGE ( 'NONE', *, *, #71153, .T. ) ;
#191634=AXIS2_PLACEMENT_3D ( 'NONE', #44513, #124048, #203572 ) ;
#191656=ORIENTED_EDGE ( 'NONE', *, *, #92123, .T. ) ;
#191687=EDGE_CURVE ( 'NONE', #204739, #231683, #123661, .T. ) ;
#191690=VERTEX_POINT ( 'NONE', #110497 ) ;
#191698=CARTESIAN_POINT ( 'NONE',  ( 23.14999999999999858, 0.000000000000000000, -33.50000000000000000 ) ) ;
#191728=CYLINDRICAL_SURFACE ( 'NONE', #75328, 0.09999999999999939493 ) ;
#191733=CARTESIAN_POINT ( 'NONE',  ( -22.49510344025093644, 0.06712767819425934090, 11.64997010511425835 ) ) ;
#191753=EDGE_CURVE ( 'NONE', #222808, #142144, #88343, .T. ) ;
#191770=ORIENTED_EDGE ( 'NONE', *, *, #40372, .T. ) ;
#191777=CARTESIAN_POINT ( 'NONE',  ( -18.59999999999999787, 9.350000000000001421, -12.34999999999999964 ) ) ;
#191803=DIRECTION ( 'NONE',  ( -0.000000000000000000, 0.000000000000000000, 1.000000000000000000 ) ) ;
#191808=ORIENTED_EDGE ( 'NONE', *, *, #111081, .F. ) ;
#191813=DIRECTION ( 'NONE',  ( 1.000000000000000000, 2.952720810173289112E-16, -0.000000000000000000 ) ) ;
#191836=B_SPLINE_CURVE_WITH_KNOTS ( 'NONE', 3,
 ( #79504, #238595, #18269, #142055, #122517, #202043, #3841 ),
 .UNSPECIFIED., .F., .F.,
 ( 4, 3, 4 ),
 ( 0.000000000000000000, 0.0009834301579439998740, 0.001767853679402675614 ),
 .UNSPECIFIED. ) ;
#191880=EDGE_LOOP ( 'NONE', ( #53339, #135276, #210111, #76559 ) ) ;
#191882=CARTESIAN_POINT ( 'NONE',  ( -21.14999999999999858, 6.540656951701240729, 0.000000000000000000 ) ) ;
#191917=VERTEX_POINT ( 'NONE', #58207 ) ;
#191932=ORIENTED_EDGE ( 'NONE', *, *, #126569, .F. ) ;
#191939=AXIS2_PLACEMENT_3D ( 'NONE', #135232, #156130, #15326 ) ;
#191967=VERTEX_POINT ( 'NONE', #22987 ) ;
#191990=FACE_OUTER_BOUND ( 'NONE', #138311, .T. ) ;
#192022=DIRECTION ( 'NONE',  ( 0.000000000000000000, 0.000000000000000000, -1.000000000000000000 ) ) ;
#192049=ORIENTED_EDGE ( 'NONE', *, *, #198337, .T. ) ;
#192063=LINE ( 'NONE', #34285, #16751 ) ;
#192073=VERTEX_POINT ( 'NONE', #127196 ) ;
#192082=AXIS2_PLACEMENT_3D ( 'NONE', #133736, #93325, #154625 ) ;
#192093=CARTESIAN_POINT ( 'NONE',  ( -23.25000000000000000, 0.000000000000000000, 0.000000000000000000 ) ) ;
#192099=ORIENTED_EDGE ( 'NONE', *, *, #127025, .F. ) ;
#192114=CARTESIAN_POINT ( 'NONE',  ( -23.25000000000000000, 4.959819536546777642E-16, 4.049999999999998934 ) ) ;
#192123=ORIENTED_EDGE ( 'NONE', *, *, #37960, .T. ) ;
#192131=ORIENTED_EDGE ( 'NONE', *, *, #19944, .F. ) ;
#192132=DIRECTION ( 'NONE',  ( 0.000000000000000000, 0.000000000000000000, 1.000000000000000000 ) ) ;
#192178=DIRECTION ( 'NONE',  ( -1.000000000000000000, 0.000000000000000000, 0.000000000000000000 ) ) ;
#192179=CARTESIAN_POINT ( 'NONE',  ( 23.24999999999999289, 11.65000000000000746, -26.48519422934606027 ) ) ;
#192192=DIRECTION ( 'NONE',  ( 0.000000000000000000, 0.000000000000000000, -1.000000000000000000 ) ) ;
#192201=AXIS2_PLACEMENT_3D ( 'NONE', #873, #21769, #225062 ) ;
#192246=CARTESIAN_POINT ( 'NONE',  ( -21.05000000000000071, 0.000000000000000000, 0.000000000000000000 ) ) ;
#192260=( LENGTH_UNIT ( ) NAMED_UNIT ( * ) SI_UNIT ( .MILLI., .METRE. ) );
#192291=DIRECTION ( 'NONE',  ( 0.000000000000000000, 1.000000000000000000, 0.000000000000000000 ) ) ;
#192295=ORIENTED_EDGE ( 'NONE', *, *, #56567, .T. ) ;
#192300=ORIENTED_EDGE ( 'NONE', *, *, #151762, .F. ) ;
#192305=CARTESIAN_POINT ( 'NONE',  ( 21.05193202509564543, 10.72393601969718802, -12.17253460332576331 ) ) ;
#192339=DIRECTION ( 'NONE',  ( 0.000000000000000000, 1.000000000000000000, 0.000000000000000000 ) ) ;
#192342=ORIENTED_EDGE ( 'NONE', *, *, #35631, .F. ) ;
#192364=EDGE_CURVE ( 'NONE', #37872, #216320, #170934, .T. ) ;
#192376=DIRECTION ( 'NONE',  ( -1.000000000000000000, -0.000000000000000000, -0.000000000000000000 ) ) ;
#192390=CARTESIAN_POINT ( 'NONE',  ( 22.57320508075687115, 11.75000000000000000, 0.000000000000000000 ) ) ;
#192395=B_SPLINE_CURVE_WITH_KNOTS ( 'NONE', 3,
 ( #236844, #256348, #55611, #233029, #75241, #36103, #116908, #77758 ),
 .UNSPECIFIED., .F., .F.,
 ( 4, 2, 2, 4 ),
 ( 0.000000000000000000, 0.0001049670497870001246, 0.0002099340995740002491, 0.0004198681991479959446 ),
 .UNSPECIFIED. ) ;
#192420=CARTESIAN_POINT ( 'NONE',  ( 20.95262331984765325, 10.50415726278985851, -7.560888329593319135 ) ) ;
#192423=ADVANCED_FACE ( 'NONE', ( #129454 ), #66827, .T. ) ;
#192455=CARTESIAN_POINT ( 'NONE',  ( -20.64999999999999858, 0.000000000000000000, -33.50000000000000000 ) ) ;
#192484=EDGE_CURVE ( 'NONE', #151938, #26951, #95839, .T. ) ;
#192511=CARTESIAN_POINT ( 'NONE',  ( -18.50000000000000000, 1.637172712970379918, -11.58215336547201879 ) ) ;
#192522=CARTESIAN_POINT ( 'NONE',  ( 22.47071067811864964, 0.09909245470260576172, 7.720074744498039543 ) ) ;
#192563=EDGE_CURVE ( 'NONE', #106654, #71518, #16909, .T. ) ;
#192576=CARTESIAN_POINT ( 'NONE',  ( 20.94999999999999929, -11.64999999999999147, -30.50000000000000000 ) ) ;
#192582=EDGE_LOOP ( 'NONE', ( #182224, #129554, #157949, #251914 ) ) ;
#192585=ORIENTED_EDGE ( 'NONE', *, *, #178011, .T. ) ;
#192635=EDGE_CURVE ( 'NONE', #169096, #94374, #162848, .T. ) ;
#192659=VERTEX_POINT ( 'NONE', #5005 ) ;
#192666=CARTESIAN_POINT ( 'NONE',  ( -20.94999999999999929, -1.835341550224413698, -11.55515129256298046 ) ) ;
#192754=CARTESIAN_POINT ( 'NONE',  ( -18.33981767444264932, -9.569575789804277477, -40.31916184372506251 ) ) ;
#192764=ORIENTED_EDGE ( 'NONE', *, *, #246037, .T. ) ;
#192773=CARTESIAN_POINT ( 'NONE',  ( 20.94999999999999574, -11.74999999999999112, -3.100000000000001865 ) ) ;
#192796=DIRECTION ( 'NONE',  ( 2.952720810173289112E-16, -1.000000000000000000, 0.000000000000000000 ) ) ;
#192808=EDGE_CURVE ( 'NONE', #61026, #62345, #176977, .T. ) ;
#192810=VERTEX_POINT ( 'NONE', #40035 ) ;
#192816=VECTOR ( 'NONE', #254372, 1000.000000000000000 ) ;
#192819=EDGE_CURVE ( 'NONE', #18698, #29243, #29445, .T. ) ;
#192826=CARTESIAN_POINT ( 'NONE',  ( -20.00857864376270001, 9.350000000000001421, -12.34999999999999964 ) ) ;
#192874=ORIENTED_EDGE ( 'NONE', *, *, #10707, .T. ) ;
#192880=EDGE_LOOP ( 'NONE', ( #124927, #26901, #5471, #108794 ) ) ;
#192891=ORIENTED_EDGE ( 'NONE', *, *, #214391, .F. ) ;
#192906=CARTESIAN_POINT ( 'NONE',  ( -22.50000000000000000, 0.000000000000000000, 6.249999999999998224 ) ) ;
#192935=CARTESIAN_POINT ( 'NONE',  ( 20.94999999999999929, 5.900000000000005684, -23.28090023534362629 ) ) ;
#192962=CARTESIAN_POINT ( 'NONE',  ( 22.41477678272288188, 0.0008238657629441799605, 11.64958528451539976 ) ) ;
#192963=AXIS2_PLACEMENT_3D ( 'NONE', #21044, #180107, #80972 ) ;
#192993=DIRECTION ( 'NONE',  ( 1.000000000000000000, -0.000000000000000000, -0.000000000000000000 ) ) ;
#193018=CARTESIAN_POINT ( 'NONE',  ( 18.49999999999999289, 10.34378108835317711, -24.82844527787753464 ) ) ;
#193022=ORIENTED_EDGE ( 'NONE', *, *, #253639, .F. ) ;
#193046=ORIENTED_EDGE ( 'NONE', *, *, #78182, .T. ) ;
#193058=CIRCLE ( 'NONE', #234739, 0.1000000000000001582 ) ;
#193075=EDGE_CURVE ( 'NONE', #220463, #4416, #187262, .T. ) ;
#193103=ORIENTED_EDGE ( 'NONE', *, *, #95479, .F. ) ;
#193119=CARTESIAN_POINT ( 'NONE',  ( 21.11101077988997332, 6.423684734726043288, 0.01528526891430725086 ) ) ;
#193139=DIRECTION ( 'NONE',  ( 0.000000000000000000, 0.000000000000000000, -1.000000000000000000 ) ) ;
#193147=CARTESIAN_POINT ( 'NONE',  ( -21.10257677756356642, 6.398381742532730065, 0.02495074956798192661 ) ) ;
#193149=FACE_OUTER_BOUND ( 'NONE', #103102, .T. ) ;
#193155=VERTEX_POINT ( 'NONE', #247171 ) ;
#193180=ADVANCED_FACE ( 'NONE', ( #54109 ), #94514, .T. ) ;
#193265=ADVANCED_FACE ( 'NONE', ( #37144 ), #155812, .F. ) ;
#193346=DIRECTION ( 'NONE',  ( 0.000000000000000000, 1.000000000000000000, 0.000000000000000000 ) ) ;
#193357=ORIENTED_EDGE ( 'NONE', *, *, #47184, .F. ) ;
#193367=EDGE_CURVE ( 'NONE', #67142, #62135, #12475, .T. ) ;
#193384=ORIENTED_EDGE ( 'NONE', *, *, #141502, .T. ) ;
#193409=FACE_OUTER_BOUND ( 'NONE', #142443, .T. ) ;
#193433=CIRCLE ( 'NONE', #147612, 0.09999999999999971412 ) ;
#193441=DIRECTION ( 'NONE',  ( 0.000000000000000000, 0.000000000000000000, -1.000000000000000000 ) ) ;
#193468=DIRECTION ( 'NONE',  ( 0.000000000000000000, 0.000000000000000000, -1.000000000000000000 ) ) ;
#193484=CARTESIAN_POINT ( 'NONE',  ( -23.15000000000000213, 2.599999999999998312, -20.27537807723789953 ) ) ;
#193514=LINE ( 'NONE', #134782, #228185 ) ;
#193532=ORIENTED_EDGE ( 'NONE', *, *, #106884, .F. ) ;
#193546=DIRECTION ( 'NONE',  ( 0.000000000000000000, 0.000000000000000000, -1.000000000000000000 ) ) ;
#193558=EDGE_CURVE ( 'NONE', #214079, #79078, #6976, .T. ) ;
#193579=EDGE_CURVE ( 'NONE', #112707, #163200, #192063, .T. ) ;
#193582=ORIENTED_EDGE ( 'NONE', *, *, #186160, .F. ) ;
#193594=AXIS2_PLACEMENT_3D ( 'NONE', #63284, #248355, #210517 ) ;
#193595=CARTESIAN_POINT ( 'NONE',  ( -23.15000000000000213, 11.65000000000000036, -21.35000000000000142 ) ) ;
#193600=CIRCLE ( 'NONE', #73014, 11.79999999999999716 ) ;
#193604=ORIENTED_EDGE ( 'NONE', *, *, #130602, .F. ) ;
#193628=CARTESIAN_POINT ( 'NONE',  ( -22.45305610364634674, -0.1008583690987139569, 11.74956712348939192 ) ) ;
#193708=CARTESIAN_POINT ( 'NONE',  ( 20.95429693346636668, 10.54330487989576781, -7.560882538313035361 ) ) ;
#193716=DIRECTION ( 'NONE',  ( 0.000000000000000000, 0.000000000000000000, 1.000000000000000000 ) ) ;
#193752=VERTEX_POINT ( 'NONE', #161921 ) ;
#193771=EDGE_CURVE ( 'NONE', #177816, #185056, #87629, .T. ) ;
#193800=AXIS2_PLACEMENT_3D ( 'NONE', #119746, #140558, #122296 ) ;
#193803=CIRCLE ( 'NONE', #164589, 0.09999999999999939493 ) ;
#193883=VERTEX_POINT ( 'NONE', #225685 ) ;
#193887=ORIENTED_EDGE ( 'NONE', *, *, #52069, .F. ) ;
#193890=CYLINDRICAL_SURFACE ( 'NONE', #15886, 0.1000000000000000194 ) ;
#193923=DIRECTION ( 'NONE',  ( 0.000000000000000000, 0.9915357197604883766, -0.1298341882519788160 ) ) ;
#193924=ORIENTED_EDGE ( 'NONE', *, *, #58403, .T. ) ;
#193980=AXIS2_PLACEMENT_3D ( 'NONE', #101239, #103838, #878 ) ;
#194009=CARTESIAN_POINT ( 'NONE',  ( 18.39999999999999858, -9.682403433476396870, -40.15684337741279109 ) ) ;
#194013=AXIS2_PLACEMENT_3D ( 'NONE', #245373, #129270, #208806 ) ;
#194033=DIRECTION ( 'NONE',  ( 0.1538461538461510236, 0.9880948137434718559, 0.000000000000000000 ) ) ;
#194046=LINE ( 'NONE', #188890, #107157 ) ;
#194064=EDGE_CURVE ( 'NONE', #214472, #67636, #146086, .T. ) ;
#194101=ORIENTED_EDGE ( 'NONE', *, *, #84634, .F. ) ;
#194141=ADVANCED_FACE ( 'NONE', ( #203288 ), #79471, .T. ) ;
#194169=( BOUNDED_SURFACE ( )  B_SPLINE_SURFACE ( 3, 2, ( 
 ( #122342, #221410, #124917 ),
 ( #123630, #24546, #143165 ),
 ( #241010, #44087, #182329 ),
 ( #102745, #144438, #161486 ) ),
 .UNSPECIFIED., .F., .F., .F. ) 
 B_SPLINE_SURFACE_WITH_KNOTS ( ( 4, 4 ),
 ( 3, 3 ),
 ( 0.04058434257139457990, 0.04256401539001584966 ),
 ( 0.000000000000000000, 1.000000000000000000 ),
 .UNSPECIFIED. ) 
 GEOMETRIC_REPRESENTATION_ITEM ( )  RATIONAL_B_SPLINE_SURFACE ( (
 ( 1.000000000000000000, 0.7103081912008196719, 1.000000000000000000),
 ( 1.000000000000000000, 0.7104998333555380130, 1.000000000000000000),
 ( 1.000000000000000000, 0.7107238315755268765, 1.000000000000000000),
 ( 1.000000000000000000, 0.7110073749539379540, 1.000000000000000000) ) ) 
 REPRESENTATION_ITEM ( '' )  SURFACE ( )  );
#194198=EDGE_CURVE ( 'NONE', #177816, #157290, #112781, .T. ) ;
#194250=DIRECTION ( 'NONE',  ( 0.000000000000000000, 0.000000000000000000, 1.000000000000000000 ) ) ;
#194266=CARTESIAN_POINT ( 'NONE',  ( 22.48508240969612615, 0.04627641451691485996, 11.65001073157356792 ) ) ;
#194278=EDGE_CURVE ( 'NONE', #62345, #168131, #38155, .T. ) ;
#194282=ADVANCED_FACE ( 'NONE', ( #150696 ), #111571, .F. ) ;
#194285=ORIENTED_EDGE ( 'NONE', *, *, #134483, .T. ) ;
#194288=DIRECTION ( 'NONE',  ( 0.000000000000000000, -1.000000000000000000, 0.000000000000000000 ) ) ;
#194307=AXIS2_PLACEMENT_3D ( 'NONE', #101181, #178233, #159947 ) ;
#194322=CARTESIAN_POINT ( 'NONE',  ( 18.59999999999999076, 6.550000000000000711, -10.01702717044001822 ) ) ;
#194325=ORIENTED_EDGE ( 'NONE', *, *, #58820, .T. ) ;
#194330=DIRECTION ( 'NONE',  ( 0.000000000000000000, 1.776356839400250267E-15, -1.000000000000000000 ) ) ;
#194337=CARTESIAN_POINT ( 'NONE',  ( -21.44999999999999929, 7.349999999999998757, -21.15000000000000213 ) ) ;
#194349=PLANE ( 'NONE',  #2977 ) ;
#194353=TOROIDAL_SURFACE ( 'NONE', #190238, 0.4000000000000003553, 0.1000000000000000056 ) ;
#194410=DIRECTION ( 'NONE',  ( 1.000000000000000000, 0.000000000000000000, 0.000000000000000000 ) ) ;
#194414=AXIS2_PLACEMENT_3D ( 'NONE', #21643, #238098, #59432 ) ;
#194415=CARTESIAN_POINT ( 'NONE',  ( 21.09316766718127667, 6.370153312474412743, 0.03926340231470034497 ) ) ;
#194434=CARTESIAN_POINT ( 'NONE',  ( 23.15000000000000213, -11.64999999999999147, -30.50000000000000000 ) ) ;
#194440=VECTOR ( 'NONE', #170824, 1000.000000000000000 ) ;
#194471=ORIENTED_EDGE ( 'NONE', *, *, #121864, .F. ) ;
#194511=ORIENTED_EDGE ( 'NONE', *, *, #256833, .T. ) ;
#194519=ORIENTED_EDGE ( 'NONE', *, *, #109051, .F. ) ;
#194523=EDGE_CURVE ( 'NONE', #257538, #225666, #112963, .T. ) ;
#194533=DIRECTION ( 'NONE',  ( 0.000000000000000000, -0.9893560106964500722, 0.1455152366551550613 ) ) ;
#194537=AXIS2_PLACEMENT_3D ( 'NONE', #105189, #4824, #83064 ) ;
#194551=DIRECTION ( 'NONE',  ( 0.000000000000000000, -0.000000000000000000, 1.000000000000000000 ) ) ;
#194577=ORIENTED_EDGE ( 'NONE', *, *, #141432, .F. ) ;
#194598=DIRECTION ( 'NONE',  ( 1.000000000000000000, -0.000000000000000000, -0.000000000000000000 ) ) ;
#194617=CIRCLE ( 'NONE', #82126, 0.09999999999999939493 ) ;
#194620=VECTOR ( 'NONE', #95456, 1000.000000000000000 ) ;
#194634=DIRECTION ( 'NONE',  ( 0.000000000000000000, -0.9887567792719341719, -0.1495327102803664099 ) ) ;
#194647=EDGE_CURVE ( 'NONE', #116070, #158940, #163232, .T. ) ;
#194654=ORIENTED_EDGE ( 'NONE', *, *, #75131, .F. ) ;
#194688=ORIENTED_EDGE ( 'NONE', *, *, #94918, .T. ) ;
#194698=CYLINDRICAL_SURFACE ( 'NONE', #89284, 0.1000000000000028644 ) ;
#194712=DIRECTION ( 'NONE',  ( 1.000000000000000000, 2.952720810173289112E-16, -0.000000000000000000 ) ) ;
#194720=VERTEX_POINT ( 'NONE', #191445 ) ;
#194733=DIRECTION ( 'NONE',  ( 1.000000000000000000, 0.000000000000000000, 0.000000000000000000 ) ) ;
#194765=DIRECTION ( 'NONE',  ( 1.000000000000000000, 0.000000000000000000, 0.000000000000000000 ) ) ;
#194769=DIRECTION ( 'NONE',  ( -0.000000000000000000, -0.000000000000000000, -1.000000000000000000 ) ) ;
#194816=AXIS2_PLACEMENT_3D ( 'NONE', #188562, #230252, #9926 ) ;
#194848=DIRECTION ( 'NONE',  ( -1.000000000000000000, -0.000000000000000000, -0.000000000000000000 ) ) ;
#194893=DIRECTION ( 'NONE',  ( 1.000000000000000000, 0.000000000000000000, 0.000000000000000000 ) ) ;
#194959=EDGE_CURVE ( 'NONE', #120793, #216320, #113517, .T. ) ;
#194980=FACE_OUTER_BOUND ( 'NONE', #46177, .T. ) ;
#195003=EDGE_LOOP ( 'NONE', ( #127768, #47946, #66714, #198864 ) ) ;
#195008=ORIENTED_EDGE ( 'NONE', *, *, #19256, .F. ) ;
#195021=ORIENTED_EDGE ( 'NONE', *, *, #213948, .T. ) ;
#195023=DIRECTION ( 'NONE',  ( 1.000000000000000000, -0.000000000000000000, -0.000000000000000000 ) ) ;
#195037=CIRCLE ( 'NONE', #124299, 12.77500000000000036 ) ;
#195050=LINE ( 'NONE', #153381, #5538 ) ;
#195095=EDGE_CURVE ( 'NONE', #11636, #44715, #205063, .T. ) ;
#195134=CARTESIAN_POINT ( 'NONE',  ( -23.25000000000000000, 11.65000000000000036, 0.000000000000000000 ) ) ;
#195148=EDGE_CURVE ( 'NONE', #11036, #126038, #170299, .T. ) ;
#195176=ORIENTED_EDGE ( 'NONE', *, *, #127025, .T. ) ;
#195195=CARTESIAN_POINT ( 'NONE',  ( -20.85000000000000142, 10.33248238082518711, -39.09484654391314962 ) ) ;
#195202=FACE_OUTER_BOUND ( 'NONE', #102818, .T. ) ;
#195210=AXIS2_PLACEMENT_3D ( 'NONE', #136099, #133564, #55275 ) ;
#195234=ORIENTED_EDGE ( 'NONE', *, *, #31337, .F. ) ;
#195278=CARTESIAN_POINT ( 'NONE',  ( 21.11344571971284623, 10.61787902351794699, -12.24602089239997227 ) ) ;
#195300=ORIENTED_EDGE ( 'NONE', *, *, #157742, .F. ) ;
#195307=EDGE_CURVE ( 'NONE', #117327, #50256, #171812, .T. ) ;
#195323=DIRECTION ( 'NONE',  ( 0.000000000000000000, 1.000000000000000000, 0.000000000000000000 ) ) ;
#195346=DIRECTION ( 'NONE',  ( 0.000000000000000000, -0.000000000000000000, 1.000000000000000000 ) ) ;
#195349=EDGE_LOOP ( 'NONE', ( #7592, #107149, #190768, #221317 ) ) ;
#195388=ORIENTED_EDGE ( 'NONE', *, *, #31507, .T. ) ;
#195391=AXIS2_PLACEMENT_3D ( 'NONE', #86859, #105120, #24368 ) ;
#195404=DIRECTION ( 'NONE',  ( 1.000000000000000000, 0.000000000000000000, 0.000000000000000000 ) ) ;
#195411=AXIS2_PLACEMENT_3D ( 'NONE', #166515, #83054, #63519 ) ;
#195446=ADVANCED_FACE ( 'NONE', ( #3147 ), #26608, .T. ) ;
#195465=CARTESIAN_POINT ( 'NONE',  ( -21.09316766718153247, 0.03926340231467564945, 6.370153312474713836 ) ) ;
#195509=CYLINDRICAL_SURFACE ( 'NONE', #256731, 0.09999999999999939493 ) ;
#195546=CARTESIAN_POINT ( 'NONE',  ( 22.44352723754029810, 0.009277095043280617764, 11.64972134534870563 ) ) ;
#195567=CARTESIAN_POINT ( 'NONE',  ( -20.64999999999999858, 1.999999999999998224, -20.27537807723789953 ) ) ;
#195568=DIRECTION ( 'NONE',  ( -1.000000000000000000, 0.000000000000000000, 0.000000000000000000 ) ) ;
#195571=CARTESIAN_POINT ( 'NONE',  ( -22.41119224318417125, 0.000000000000000000, 11.64957080754479968 ) ) ;
#195591=DIRECTION ( 'NONE',  ( -1.000000000000000000, -0.000000000000000000, 0.000000000000000000 ) ) ;
#195592=AXIS2_PLACEMENT_3D ( 'NONE', #180825, #120873, #2157 ) ;
#195600=CARTESIAN_POINT ( 'NONE',  ( 18.49999999999998934, 10.28015861705704737, -24.72457207120110922 ) ) ;
#195692=DIRECTION ( 'NONE',  ( -0.000000000000000000, -0.7397360091702755991, -0.6728971962616832059 ) ) ;
#195698=AXIS2_PLACEMENT_3D ( 'NONE', #8727, #176485, #172668 ) ;
#195735=DIRECTION ( 'NONE',  ( 0.000000000000000000, 0.000000000000000000, -1.000000000000000000 ) ) ;
#195784=LINE ( 'NONE', #78361, #113876 ) ;
#195789=DIRECTION ( 'NONE',  ( 1.000000000000000000, 0.000000000000000000, 0.000000000000000000 ) ) ;
#195792=ORIENTED_EDGE ( 'NONE', *, *, #238538, .T. ) ;
#195824=ORIENTED_EDGE ( 'NONE', *, *, #104963, .F. ) ;
#195853=DIRECTION ( 'NONE',  ( -1.000000000000000000, 0.000000000000000000, 0.000000000000000000 ) ) ;
#195874=AXIS2_PLACEMENT_3D ( 'NONE', #197301, #103328, #99467 ) ;
#195884=ORIENTED_EDGE ( 'NONE', *, *, #39966, .F. ) ;
#195886=VERTEX_POINT ( 'NONE', #184065 ) ;
#195899=DIRECTION ( 'NONE',  ( 1.000000000000000000, 0.000000000000000000, 0.000000000000000000 ) ) ;
#195908=CARTESIAN_POINT ( 'NONE',  ( 23.14999999999999858, 0.000000000000000000, -33.50000000000000000 ) ) ;
#195916=AXIS2_PLACEMENT_3D ( 'NONE', #140873, #125167, #200846 ) ;
#195961=EDGE_LOOP ( 'NONE', ( #99734, #204628, #93694, #20804 ) ) ;
#195968=EDGE_CURVE ( 'NONE', #16790, #5236, #42972, .T. ) ;
#195973=ADVANCED_FACE ( 'NONE', ( #247892 ), #207506, .T. ) ;
#195977=AXIS2_PLACEMENT_3D ( 'NONE', #1934, #21535, #223553 ) ;
#196028=CARTESIAN_POINT ( 'NONE',  ( 23.14999999999999503, 6.550000000000000711, -21.15000000000000213 ) ) ;
#196054=FACE_OUTER_BOUND ( 'NONE', #222116, .T. ) ;
#196061=ORIENTED_EDGE ( 'NONE', *, *, #75383, .T. ) ;
#196067=EDGE_LOOP ( 'NONE', ( #2119, #149625, #46762, #238912 ) ) ;
#196082=EDGE_CURVE ( 'NONE', #74339, #72992, #147867, .T. ) ;
#196091=ORIENTED_EDGE ( 'NONE', *, *, #180845, .F. ) ;
#196102=VECTOR ( 'NONE', #172935, 1000.000000000000000 ) ;
#196103=CIRCLE ( 'NONE', #87744, 0.1000000000000000472 ) ;
#196115=DIRECTION ( 'NONE',  ( 0.000000000000000000, 1.000000000000000000, 2.891205793294679805E-16 ) ) ;
#196175=ORIENTED_EDGE ( 'NONE', *, *, #224221, .T. ) ;
#196185=EDGE_CURVE ( 'NONE', #226600, #11036, #23099, .T. ) ;
#196187=DIRECTION ( 'NONE',  ( -1.000000000000000000, -1.836970198721029934E-16, 0.000000000000000000 ) ) ;
#196192=CARTESIAN_POINT ( 'NONE',  ( 20.94999999999999929, 11.65000000000000391, -26.71613433702190932 ) ) ;
#196230=CARTESIAN_POINT ( 'NONE',  ( -23.15000000000000213, 0.000000000000000000, 0.000000000000000000 ) ) ;
#196246=ADVANCED_FACE ( 'NONE', ( #221255, #184706 ), #84271, .F. ) ;
#196280=DIRECTION ( 'NONE',  ( -0.000000000000000000, 1.000000000000000000, -0.000000000000000000 ) ) ;
#196296=ORIENTED_EDGE ( 'NONE', *, *, #221568, .F. ) ;
#196311=EDGE_LOOP ( 'NONE', ( #240300, #200240, #166342, #78247 ) ) ;
#196320=FACE_OUTER_BOUND ( 'NONE', #97373, .T. ) ;
#196342=DIRECTION ( 'NONE',  ( -1.000000000000000000, -3.265361837132813093E-16, 0.000000000000000000 ) ) ;
#196343=VECTOR ( 'NONE', #223265, 1000.000000000000000 ) ;
#196350=LINE ( 'NONE', #36018, #84624 ) ;
#196352=AXIS2_PLACEMENT_3D ( 'NONE', #27304, #88494, #246319 ) ;
#196373=ORIENTED_EDGE ( 'NONE', *, *, #253602, .T. ) ;
#196401=VERTEX_POINT ( 'NONE', #116731 ) ;
#196404=DIRECTION ( 'NONE',  ( 2.952720810173289112E-16, -1.000000000000000000, 0.000000000000000000 ) ) ;
#196427=DIRECTION ( 'NONE',  ( 0.000000000000000000, 0.000000000000000000, 1.000000000000000000 ) ) ;
#196433=DIRECTION ( 'NONE',  ( 0.000000000000000000, 0.000000000000000000, 1.000000000000000000 ) ) ;
#196441=DIRECTION ( 'NONE',  ( 1.000000000000000000, -0.000000000000000000, -0.000000000000000000 ) ) ;
#196442=EDGE_LOOP ( 'NONE', ( #165721, #243615, #65535, #172540 ) ) ;
#196444=CARTESIAN_POINT ( 'NONE',  ( -21.05000000000000071, 13.99999999999999822, -28.07290746961752603 ) ) ;
#196465=CARTESIAN_POINT ( 'NONE',  ( -18.59999999999999787, -1.835341550224411922, -11.55515129256297868 ) ) ;
#196474=ORIENTED_EDGE ( 'NONE', *, *, #239153, .T. ) ;
#196537=DIRECTION ( 'NONE',  ( 1.000000000000000000, -0.000000000000000000, -0.000000000000000000 ) ) ;
#196553=ADVANCED_FACE ( 'NONE', ( #222229 ), #167931, .F. ) ;
#196554=EDGE_CURVE ( 'NONE', #28425, #79078, #130478, .T. ) ;
#196585=CARTESIAN_POINT ( 'NONE',  ( 23.14999999999999858, 4.999999999999997335, -21.09473398108690390 ) ) ;
#196617=ORIENTED_EDGE ( 'NONE', *, *, #75829, .T. ) ;
#196687=ORIENTED_EDGE ( 'NONE', *, *, #32369, .F. ) ;
#196783=CIRCLE ( 'NONE', #84294, 0.09999999999999939493 ) ;
#196802=DIRECTION ( 'NONE',  ( 0.000000000000000000, -1.000000000000000000, -0.000000000000000000 ) ) ;
#196812=FACE_OUTER_BOUND ( 'NONE', #8282, .T. ) ;
#196820=DIRECTION ( 'NONE',  ( 0.000000000000000000, -0.8700118002898321601, 0.4930308989875230030 ) ) ;
#196829=FACE_OUTER_BOUND ( 'NONE', #162225, .T. ) ;
#196830=DIRECTION ( 'NONE',  ( 0.000000000000000000, 0.9999631594459056361, -0.008583690987128059571 ) ) ;
#196937=AXIS2_PLACEMENT_3D ( 'NONE', #243099, #43628, #163576 ) ;
#196950=ORIENTED_EDGE ( 'NONE', *, *, #14166, .T. ) ;
#196952=EDGE_CURVE ( 'NONE', #11085, #68838, #162006, .T. ) ;
#196978=DIRECTION ( 'NONE',  ( 0.000000000000000000, 0.9908441862701596881, -0.1350103645451904977 ) ) ;
#197025=CARTESIAN_POINT ( 'NONE',  ( -20.94999999999999929, -11.48912529307605546, -30.50000000000000000 ) ) ;
#197037=VERTEX_POINT ( 'NONE', #90125 ) ;
#197079=CARTESIAN_POINT ( 'NONE',  ( -20.54999999999999716, 1.999999999999998224, -13.22462192276210224 ) ) ;
#197081=FACE_OUTER_BOUND ( 'NONE', #23397, .T. ) ;
#197101=DIRECTION ( 'NONE',  ( 1.000000000000000000, 0.000000000000000000, -0.000000000000000000 ) ) ;
#197113=ORIENTED_EDGE ( 'NONE', *, *, #230207, .F. ) ;
#197115=CARTESIAN_POINT ( 'NONE',  ( -21.05000000000000071, -11.65000000000000036, -3.000000000000002665 ) ) ;
#197118=FACE_OUTER_BOUND ( 'NONE', #135969, .T. ) ;
#197159=DIRECTION ( 'NONE',  ( -0.7071067811865475727, -0.7071067811865475727, 0.000000000000000000 ) ) ;
#197163=CIRCLE ( 'NONE', #247228, 0.1000000000000002554 ) ;
#197168=ORIENTED_EDGE ( 'NONE', *, *, #67837, .T. ) ;
#197174=ADVANCED_FACE ( 'NONE', ( #174873 ), #93984, .T. ) ;
#197195=CARTESIAN_POINT ( 'NONE',  ( -21.05000000000000071, -0.2561057920922211739, 0.03489644167229202787 ) ) ;
#197218=CARTESIAN_POINT ( 'NONE',  ( -18.45140287520617761, -9.486077739529564568, -40.14052312668610512 ) ) ;
#197230=EDGE_LOOP ( 'NONE', ( #76297, #96551, #182352, #182944 ) ) ;
#197248=AXIS2_PLACEMENT_3D ( 'NONE', #4546, #84043, #206613 ) ;
#197257=DIRECTION ( 'NONE',  ( 1.000000000000000000, 0.000000000000000000, 0.000000000000000000 ) ) ;
#197300=VERTEX_POINT ( 'NONE', #243777 ) ;
#197301=CARTESIAN_POINT ( 'NONE',  ( -23.15000000000000213, 4.150000000000001243, -21.14999999999999858 ) ) ;
#197317=ORIENTED_EDGE ( 'NONE', *, *, #146802, .T. ) ;
#197338=FACE_OUTER_BOUND ( 'NONE', #118849, .T. ) ;
#197345=ORIENTED_EDGE ( 'NONE', *, *, #6525, .T. ) ;
#197368=AXIS2_PLACEMENT_3D ( 'NONE', #86000, #69061, #106868 ) ;
#197383=AXIS2_PLACEMENT_3D ( 'NONE', #35338, #217759, #58685 ) ;
#197410=ORIENTED_EDGE ( 'NONE', *, *, #142824, .F. ) ;
#197422=CARTESIAN_POINT ( 'NONE',  ( 21.13507111622890022, 10.71768338699838807, -12.24916858636078842 ) ) ;
#197463=CARTESIAN_POINT ( 'NONE',  ( -22.50000000000000000, 0.000000000000000000, 11.64957080754479968 ) ) ;
#197492=AXIS2_PLACEMENT_3D ( 'NONE', #18139, #97649, #177247 ) ;
#197497=EDGE_CURVE ( 'NONE', #49158, #106325, #174567, .T. ) ;
#197500=DIRECTION ( 'NONE',  ( 1.000000000000000000, -0.000000000000000000, -0.000000000000000000 ) ) ;
#197501=CARTESIAN_POINT ( 'NONE',  ( 18.52928932188133970, 10.27928932188134858, -24.65000000000000213 ) ) ;
#197544=ADVANCED_FACE ( 'NONE', ( #132828 ), #190282, .T. ) ;
#197546=VECTOR ( 'NONE', #235485, 1000.000000000000000 ) ;
#197548=DIRECTION ( 'NONE',  ( 0.000000000000000000, 0.000000000000000000, 1.000000000000000000 ) ) ;
#197591=ORIENTED_EDGE ( 'NONE', *, *, #215535, .F. ) ;
#197601=DIRECTION ( 'NONE',  ( 0.000000000000000000, 0.000000000000000000, -1.000000000000000000 ) ) ;
#197636=CIRCLE ( 'NONE', #85183, 0.1000000000000001860 ) ;
#197659=DIRECTION ( 'NONE',  ( 0.000000000000000000, 1.734723475976807292E-15, -1.000000000000000000 ) ) ;
#197671=ORIENTED_EDGE ( 'NONE', *, *, #11284, .F. ) ;
#197726=DIRECTION ( 'NONE',  ( 1.000000000000000000, 0.000000000000000000, -0.000000000000000000 ) ) ;
#197733=DIRECTION ( 'NONE',  ( 0.000000000000000000, 0.8660254037844384856, -0.5000000000000003331 ) ) ;
#197743=EDGE_CURVE ( 'NONE', #252270, #151938, #14363, .T. ) ;
#197763=ORIENTED_EDGE ( 'NONE', *, *, #31328, .T. ) ;
#197777=VERTEX_POINT ( 'NONE', #192179 ) ;
#197788=ORIENTED_EDGE ( 'NONE', *, *, #222483, .T. ) ;
#197872=ORIENTED_EDGE ( 'NONE', *, *, #101390, .T. ) ;
#197899=FACE_OUTER_BOUND ( 'NONE', #104342, .T. ) ;
#197929=FACE_OUTER_BOUND ( 'NONE', #102041, .T. ) ;
#197950=DIRECTION ( 'NONE',  ( 0.000000000000000000, -0.1298341882520022694, -0.9915357197604852679 ) ) ;
#197965=VERTEX_POINT ( 'NONE', #223263 ) ;
#197977=CARTESIAN_POINT ( 'NONE',  ( 21.05000000000000071, -9.000000000000000000, -24.00603087734755547 ) ) ;
#197980=CARTESIAN_POINT ( 'NONE',  ( 22.39999999999999503, 11.75000000000000000, 0.09999999999999592548 ) ) ;
#197989=CARTESIAN_POINT ( 'NONE',  ( -21.08134388332232589, 0.07581891750697818122, 6.334680580517975557 ) ) ;
#198008=CARTESIAN_POINT ( 'NONE',  ( 21.14999999999999858, 0.000000000000000000, -0.09999999999999592548 ) ) ;
#198045=ORIENTED_EDGE ( 'NONE', *, *, #85001, .F. ) ;
#198048=CIRCLE ( 'NONE', #256234, 0.09999999999999999167 ) ;
#198064=LINE ( 'NONE', #57251, #149784 ) ;
#198069=EDGE_CURVE ( 'NONE', #24262, #176398, #40387, .T. ) ;
#198072=CARTESIAN_POINT ( 'NONE',  ( -20.94999999999999929, 0.000000000000000000, -33.50000000000000000 ) ) ;
#198076=ORIENTED_EDGE ( 'NONE', *, *, #81759, .F. ) ;
#198081=DIRECTION ( 'NONE',  ( -1.000000000000000000, -0.000000000000000000, -0.000000000000000000 ) ) ;
#198085=CARTESIAN_POINT ( 'NONE',  ( 20.30531438145591139, 10.09690106109084695, -7.796017807273384115 ) ) ;
#198105=DIRECTION ( 'NONE',  ( 1.000000000000000000, 0.000000000000000000, 0.000000000000000000 ) ) ;
#198142=DIRECTION ( 'NONE',  ( -1.000000000000000000, 0.000000000000000000, 0.000000000000000000 ) ) ;
#198164=EDGE_CURVE ( 'NONE', #5222, #148838, #93619, .T. ) ;
#198168=CARTESIAN_POINT ( 'NONE',  ( -23.15000000000000213, 0.000000000000000000, -33.50000000000000000 ) ) ;
#198173=CARTESIAN_POINT ( 'NONE',  ( 20.94999999999999574, -1.835341550224411922, -11.55515129256298046 ) ) ;
#198187=FACE_OUTER_BOUND ( 'NONE', #252709, .T. ) ;
#198199=DIRECTION ( 'NONE',  ( 0.000000000000000000, 0.1350103645451904977, 0.9908441862701596881 ) ) ;
#198200=ORIENTED_EDGE ( 'NONE', *, *, #117338, .F. ) ;
#198210=CARTESIAN_POINT ( 'NONE',  ( -20.94999999999999929, 5.899999999999947065, -10.21909976465641456 ) ) ;
#198212=EDGE_LOOP ( 'NONE', ( #70697, #175252, #91299, #66593 ) ) ;
#198214=CARTESIAN_POINT ( 'NONE',  ( -23.15000000000000213, 0.000000000000000000, -12.77499999999999858 ) ) ;
#198229=CARTESIAN_POINT ( 'NONE',  ( 21.08134388332232234, 6.334680580517956905, 0.07581891750702302035 ) ) ;
#198253=AXIS2_PLACEMENT_3D ( 'NONE', #192246, #108827, #207961 ) ;
#198258=EDGE_LOOP ( 'NONE', ( #83118, #32081, #156685, #224914, #249999, #15883, #126134, #29716, #119567 ) ) ;
#198267=AXIS2_PLACEMENT_3D ( 'NONE', #238637, #18301, #59973 ) ;
#198275=CARTESIAN_POINT ( 'NONE',  ( 22.47071067811865319, 0.09909245470260570621, 7.720074744498046648 ) ) ;
#198281=ORIENTED_EDGE ( 'NONE', *, *, #25183, .T. ) ;
#198297=ORIENTED_EDGE ( 'NONE', *, *, #218095, .F. ) ;
#198302=ORIENTED_EDGE ( 'NONE', *, *, #25183, .F. ) ;
#198309=ORIENTED_EDGE ( 'NONE', *, *, #237579, .F. ) ;
#198312=AXIS2_PLACEMENT_3D ( 'NONE', #74853, #72259, #13570 ) ;
#198316=CIRCLE ( 'NONE', #73276, 0.09999999999999939493 ) ;
#198337=EDGE_CURVE ( 'NONE', #157290, #53632, #140727, .T. ) ;
#198340=VERTEX_POINT ( 'NONE', #218975 ) ;
#198358=ADVANCED_FACE ( 'NONE', ( #62491 ), #68882, .F. ) ;
#198380=DIRECTION ( 'NONE',  ( 3.469446951953728416E-14, -0.8660254037844309360, 0.5000000000000134337 ) ) ;
#198399=ORIENTED_EDGE ( 'NONE', *, *, #7862, .F. ) ;
#198406=VECTOR ( 'NONE', #94108, 1000.000000000000000 ) ;
#198427=ORIENTED_EDGE ( 'NONE', *, *, #39966, .T. ) ;
#198453=DIRECTION ( 'NONE',  ( 0.000000000000000000, -0.4930308989875324399, -0.8700118002898268310 ) ) ;
#198472=CYLINDRICAL_SURFACE ( 'NONE', #20412, 0.09999999999999939493 ) ;
#198475=CIRCLE ( 'NONE', #194414, 0.09999999999999939493 ) ;
#198478=CARTESIAN_POINT ( 'NONE',  ( -18.52328366898031931, -9.642321089041253401, -40.21481933757005578 ) ) ;
#198515=AXIS2_PLACEMENT_3D ( 'NONE', #31673, #194598, #192022 ) ;
#198518=CARTESIAN_POINT ( 'NONE',  ( 22.60000000000000142, 0.1008583690987122083, 11.74956712348939192 ) ) ;
#198573=CARTESIAN_POINT ( 'NONE',  ( -21.14999999999999858, 6.540656951701240729, 0.000000000000000000 ) ) ;
#198580=EDGE_CURVE ( 'NONE', #99784, #129969, #127300, .T. ) ;
#198611=EDGE_LOOP ( 'NONE', ( #73043, #223032, #246105, #215406, #86303, #151205, #177527 ) ) ;
#198633=LINE ( 'NONE', #39603, #14792 ) ;
#198647=FACE_OUTER_BOUND ( 'NONE', #113425, .T. ) ;
#198658=ORIENTED_EDGE ( 'NONE', *, *, #156283, .T. ) ;
#198695=EDGE_CURVE ( 'NONE', #255042, #185478, #73179, .T. ) ;
#198730=ADVANCED_FACE ( 'NONE', ( #221224 ), #230619, .T. ) ;
#198761=ORIENTED_EDGE ( 'NONE', *, *, #130745, .T. ) ;
#198780=ORIENTED_EDGE ( 'NONE', *, *, #3402, .T. ) ;
#198788=DIRECTION ( 'NONE',  ( 0.000000000000000000, -1.000000000000000000, 0.000000000000000000 ) ) ;
#198839=AXIS2_PLACEMENT_3D ( 'NONE', #169267, #27186, #85797 ) ;
#198849=EDGE_CURVE ( 'NONE', #59419, #120448, #171271, .T. ) ;
#198857=CIRCLE ( 'NONE', #3211, 0.1000000000000028644 ) ;
#198864=ORIENTED_EDGE ( 'NONE', *, *, #197497, .F. ) ;
#198876=CIRCLE ( 'NONE', #32330, 0.5999999999999998668 ) ;
#198913=DIRECTION ( 'NONE',  ( -1.000000000000000000, 0.000000000000000000, 0.000000000000000000 ) ) ;
#198928=CARTESIAN_POINT ( 'NONE',  ( 23.14999999999999147, -4.149999999999999467, 0.000000000000000000 ) ) ;
#198943=DIRECTION ( 'NONE',  ( 1.000000000000000000, 0.000000000000000000, 0.000000000000000000 ) ) ;
#198969=FACE_OUTER_BOUND ( 'NONE', #97313, .T. ) ;
#198974=DIRECTION ( 'NONE',  ( 0.000000000000000000, -0.8068669527896844551, -0.5907332058517525963 ) ) ;
#199007=ORIENTED_EDGE ( 'NONE', *, *, #34327, .T. ) ;
#199031=ORIENTED_EDGE ( 'NONE', *, *, #105721, .T. ) ;
#199036=AXIS2_PLACEMENT_3D ( 'NONE', #189517, #89116, #10878 ) ;
#199045=VERTEX_POINT ( 'NONE', #19864 ) ;
#199053=AXIS2_PLACEMENT_3D ( 'NONE', #57935, #234017, #179215 ) ;
#199068=LINE ( 'NONE', #119547, #106542 ) ;
#199069=ORIENTED_EDGE ( 'NONE', *, *, #57577, .T. ) ;
#199105=CARTESIAN_POINT ( 'NONE',  ( -23.25000000000000000, 0.000000000000000000, -12.77499999999999858 ) ) ;
#199141=CARTESIAN_POINT ( 'NONE',  ( 18.49999999999999289, 7.021664781900089913, -37.33356540189728889 ) ) ;
#199154=DIRECTION ( 'NONE',  ( 0.000000000000000000, 0.000000000000000000, -1.000000000000000000 ) ) ;
#199162=VERTEX_POINT ( 'NONE', #9269 ) ;
#199163=CARTESIAN_POINT ( 'NONE',  ( 21.05000000000000071, 6.540656951701244282, -0.1000000000000009354 ) ) ;
#199201=DIRECTION ( 'NONE',  ( 0.000000000000000000, 0.000000000000000000, -1.000000000000000000 ) ) ;
#199213=ADVANCED_FACE ( 'NONE', ( #155238 ), #14436, .T. ) ;
#199242=AXIS2_PLACEMENT_3D ( 'NONE', #29471, #110242, #145515 ) ;
#199289=EDGE_CURVE ( 'NONE', #115921, #206232, #96486, .T. ) ;
#199313=ORIENTED_EDGE ( 'NONE', *, *, #96836, .F. ) ;
#199327=TOROIDAL_SURFACE ( 'NONE', #95265, 0.2000000000000000111, 0.1000000000000000056 ) ;
#199342=CARTESIAN_POINT ( 'NONE',  ( -23.25000000000000000, -11.75000000000000000, -33.50000000000000000 ) ) ;
#199348=EDGE_CURVE ( 'NONE', #180003, #253474, #197636, .T. ) ;
#199358=CIRCLE ( 'NONE', #128610, 0.09999999999999939493 ) ;
#199369=ADVANCED_FACE ( 'NONE', ( #104193 ), #214568, .F. ) ;
#199381=DIRECTION ( 'NONE',  ( 0.000000000000000000, 0.000000000000000000, 1.000000000000000000 ) ) ;
#199389=CIRCLE ( 'NONE', #86903, 0.09999999999999939493 ) ;
#199417=DIRECTION ( 'NONE',  ( 1.000000000000000000, 0.000000000000000000, 0.000000000000000000 ) ) ;
#199459=( BOUNDED_SURFACE ( )  B_SPLINE_SURFACE ( 3, 2, ( 
 ( #150024, #144849, #187865 ),
 ( #146139, #105703, #48327 ),
 ( #169614, #185279, #9201 ),
 ( #229549, #6629, #50869 ),
 ( #31378, #110875, #88715 ),
 ( #86140, #27529, #245259 ) ),
 .UNSPECIFIED., .F., .F., .F. ) 
 B_SPLINE_SURFACE_WITH_KNOTS ( ( 4, 2, 4 ),
 ( 3, 3 ),
 ( 0.0001300404313046711721, 0.0003183318589266732066, 0.0005066232865486751868 ),
 ( 0.000000000000000000, 1.000000000000000000 ),
 .UNSPECIFIED. ) 
 GEOMETRIC_REPRESENTATION_ITEM ( )  RATIONAL_B_SPLINE_SURFACE ( (
 ( 1.000000000000000000, 0.7071067811865352493, 1.000000000000000000),
 ( 1.000000000000000000, 0.7625113560539715785, 1.000000000000000000),
 ( 1.000000000000000000, 0.8126073484689285698, 1.000000000000000000),
 ( 1.000000000000000000, 0.8923049332731626260, 1.000000000000000000),
 ( 1.000000000000000000, 0.9231914937770224761, 1.000000000000000000),
 ( 1.000000000000000000, 0.9238795325112909573, 1.000000000000000000) ) ) 
 REPRESENTATION_ITEM ( '' )  SURFACE ( )  );
#199480=DIRECTION ( 'NONE',  ( 0.000000000000000000, -0.5000000000000275335, -0.8660254037844228314 ) ) ;
#199492=DIRECTION ( 'NONE',  ( 0.000000000000000000, 0.000000000000000000, -1.000000000000000000 ) ) ;
#199555=EDGE_CURVE ( 'NONE', #67614, #58239, #2185, .T. ) ;
#199573=EDGE_LOOP ( 'NONE', ( #77873, #193357, #172683, #119554 ) ) ;
#199577=CARTESIAN_POINT ( 'NONE',  ( -18.59999999999999787, 11.74999999999999645, -21.35000000000000142 ) ) ;
#199652=VERTEX_POINT ( 'NONE', #12839 ) ;
#199662=VERTEX_POINT ( 'NONE', #233175 ) ;
#199667=CIRCLE ( 'NONE', #83065, 0.2000000000000000944 ) ;
#199669=AXIS2_PLACEMENT_3D ( 'NONE', #122390, #117256, #221455 ) ;
#199694=VECTOR ( 'NONE', #189902, 1000.000000000000000 ) ;
#199764=EDGE_CURVE ( 'NONE', #191355, #102134, #102295, .T. ) ;
#199768=ORIENTED_EDGE ( 'NONE', *, *, #9228, .F. ) ;
#199782=EDGE_LOOP ( 'NONE', ( #121336, #12159, #154820, #168281 ) ) ;
#199836=ORIENTED_EDGE ( 'NONE', *, *, #107678, .T. ) ;
#199869=TOROIDAL_SURFACE ( 'NONE', #112725, 4.099999999999999645, 0.1000000000000000056 ) ;
#199870=EDGE_CURVE ( 'NONE', #153115, #16503, #169025, .T. ) ;
#199888=DIRECTION ( 'NONE',  ( 1.000000000000000000, 0.000000000000000000, 0.000000000000000000 ) ) ;
#199912=AXIS2_PLACEMENT_3D ( 'NONE', #164778, #81348, #240458 ) ;
#199934=VECTOR ( 'NONE', #247821, 999.9999999999998863 ) ;
#199957=CARTESIAN_POINT ( 'NONE',  ( -21.05000000000000071, 1.162701749938009677, -7.900000000000000355 ) ) ;
#199973=DIRECTION ( 'NONE',  ( 0.000000000000000000, 0.000000000000000000, -1.000000000000000000 ) ) ;
#199975=CARTESIAN_POINT ( 'NONE',  ( -22.50000000000000000, 0.000000000000000000, 0.000000000000000000 ) ) ;
#200084=DIRECTION ( 'NONE',  ( 0.000000000000000000, 0.9908441862701596881, -0.1350103645451904977 ) ) ;
#200104=TOROIDAL_SURFACE ( 'NONE', #33737, 0.2000000000000000111, 0.1000000000000000056 ) ;
#200193=ORIENTED_EDGE ( 'NONE', *, *, #111425, .T. ) ;
#200208=ORIENTED_EDGE ( 'NONE', *, *, #188960, .F. ) ;
#200225=DIRECTION ( 'NONE',  ( 0.000000000000000000, 8.881784197001252323E-16, -1.000000000000000000 ) ) ;
#200240=ORIENTED_EDGE ( 'NONE', *, *, #201764, .F. ) ;
#200279=AXIS2_PLACEMENT_3D ( 'NONE', #170279, #175397, #134921 ) ;
#200286=EDGE_CURVE ( 'NONE', #253366, #57845, #106596, .T. ) ;
#200291=DIRECTION ( 'NONE',  ( -0.000000000000000000, 0.000000000000000000, 1.000000000000000000 ) ) ;
#200294=ORIENTED_EDGE ( 'NONE', *, *, #82800, .T. ) ;
#200295=ORIENTED_EDGE ( 'NONE', *, *, #4608, .T. ) ;
#200312=CARTESIAN_POINT ( 'NONE',  ( 22.39999999999999858, 7.790779598373383408, 0.09999999999999939493 ) ) ;
#200322=EDGE_LOOP ( 'NONE', ( #115182, #86062, #115634, #231987 ) ) ;
#200337=CIRCLE ( 'NONE', #17198, 12.87500000000000000 ) ;
#200351=SPHERICAL_SURFACE ( 'NONE', #36858, 0.1000000000000000056 ) ;
#200370=ADVANCED_FACE ( 'NONE', ( #83984 ), #203978, .F. ) ;
#200376=ADVANCED_FACE ( 'NONE', ( #48756 ), #114998, .T. ) ;
#200423=AXIS2_PLACEMENT_3D ( 'NONE', #53497, #90036, #187881 ) ;
#200429=PLANE ( 'NONE',  #115786 ) ;
#200462=EDGE_CURVE ( 'NONE', #153115, #103735, #211047, .T. ) ;
#200477=LINE ( 'NONE', #41421, #209384 ) ;
#200480=ORIENTED_EDGE ( 'NONE', *, *, #50303, .T. ) ;
#200521=ORIENTED_EDGE ( 'NONE', *, *, #106334, .T. ) ;
#200534=AXIS2_PLACEMENT_3D ( 'NONE', #236992, #235692, #219982 ) ;
#200536=CARTESIAN_POINT ( 'NONE',  ( -23.15000000000000213, 11.65000000000000036, -12.14999999999999858 ) ) ;
#200539=EDGE_LOOP ( 'NONE', ( #142230, #93251, #252866, #33057 ) ) ;
#200541=ORIENTED_EDGE ( 'NONE', *, *, #150711, .F. ) ;
#200568=ORIENTED_EDGE ( 'NONE', *, *, #82329, .T. ) ;
#200585=DIRECTION ( 'NONE',  ( 0.000000000000000000, 6.308085367188393199E-16, 1.000000000000000000 ) ) ;
#200605=CARTESIAN_POINT ( 'NONE',  ( -21.14999999999999858, 11.65000000000000036, -0.1000000000000028644 ) ) ;
#200647=DIRECTION ( 'NONE',  ( 0.000000000000000000, 1.000000000000000000, 0.000000000000000000 ) ) ;
#200648=CARTESIAN_POINT ( 'NONE',  ( -18.59999999999999787, 9.350000000000001421, -12.14999999999999858 ) ) ;
#200693=CYLINDRICAL_SURFACE ( 'NONE', #41764, 0.09999999999999939493 ) ;
#200709=DIRECTION ( 'NONE',  ( 0.000000000000000000, 0.000000000000000000, -1.000000000000000000 ) ) ;
#200724=CARTESIAN_POINT ( 'NONE',  ( -18.59999999999999787, 11.64999999999999680, -33.50000000000000000 ) ) ;
#200787=CARTESIAN_POINT ( 'NONE',  ( 21.00000000000000000, 9.749999999999998224, -12.25000000000000000 ) ) ;
#200798=CARTESIAN_POINT ( 'NONE',  ( 23.14999999999998437, 11.75000000000000000, 0.000000000000000000 ) ) ;
#200823=DIRECTION ( 'NONE',  ( 0.000000000000000000, 0.000000000000000000, 1.000000000000000000 ) ) ;
#200829=EDGE_LOOP ( 'NONE', ( #198281, #200568 ) ) ;
#200846=DIRECTION ( 'NONE',  ( 0.000000000000000000, 0.000000000000000000, -1.000000000000000000 ) ) ;
#200855=DIRECTION ( 'NONE',  ( 0.000000000000000000, 0.000000000000000000, -1.000000000000000000 ) ) ;
#200856=CYLINDRICAL_SURFACE ( 'NONE', #155532, 0.09999999999999939493 ) ;
#200859=ORIENTED_EDGE ( 'NONE', *, *, #67270, .T. ) ;
#200877=EDGE_CURVE ( 'NONE', #32374, #145748, #206760, .T. ) ;
#200950=TOROIDAL_SURFACE ( 'NONE', #5286, 12.77499999999999858, 0.1000000000000000056 ) ;
#200984=DIRECTION ( 'NONE',  ( 0.000000000000000000, 1.000000000000000000, 0.000000000000000000 ) ) ;
#200991=DIRECTION ( 'NONE',  ( 1.000000000000000000, 0.000000000000000000, 0.000000000000000000 ) ) ;
#201032=FACE_OUTER_BOUND ( 'NONE', #123027, .T. ) ;
#201075=EDGE_LOOP ( 'NONE', ( #113333, #112421, #194101, #151900 ) ) ;
#201090=CARTESIAN_POINT ( 'NONE',  ( 20.94999999999999929, -11.29603075033528192, -30.45210084033612929 ) ) ;
#201098=ORIENTED_EDGE ( 'NONE', *, *, #20511, .T. ) ;
#201101=DIRECTION ( 'NONE',  ( 0.000000000000000000, -1.000000000000000000, -2.891205793294679805E-16 ) ) ;
#201112=EDGE_CURVE ( 'NONE', #239652, #66968, #19522, .T. ) ;
#201129=CARTESIAN_POINT ( 'NONE',  ( 21.05000000000000071, 8.876614585087098774, -8.385080478844676222 ) ) ;
#201147=CARTESIAN_POINT ( 'NONE',  ( -20.94999999999999929, 0.000000000000000000, -33.50000000000000000 ) ) ;
#201148=EDGE_LOOP ( 'NONE', ( #71661, #58604, #242511, #39919, #197317, #94974, #185800, #239454, #42504, #15210, #105845, #106964, #100763, #62185, #10973, #85988, #222977, #162384 ) ) ;
#201152=CIRCLE ( 'NONE', #117945, 0.09999999999999939493 ) ;
#201155=ORIENTED_EDGE ( 'NONE', *, *, #132063, .F. ) ;
#201199=DIRECTION ( 'NONE',  ( -1.000000000000000000, -3.265361837132813093E-16, 0.000000000000000000 ) ) ;
#201201=DIRECTION ( 'NONE',  ( 0.000000000000000000, 0.000000000000000000, -1.000000000000000000 ) ) ;
#201232=CARTESIAN_POINT ( 'NONE',  ( 20.94999999999999929, 0.000000000000000000, -33.50000000000000000 ) ) ;
#201247=DIRECTION ( 'NONE',  ( 1.000000000000000000, -0.000000000000000000, -0.000000000000000000 ) ) ;
#201295=ORIENTED_EDGE ( 'NONE', *, *, #182768, .F. ) ;
#201299=EDGE_CURVE ( 'NONE', #10818, #3158, #171368, .T. ) ;
#201302=AXIS2_PLACEMENT_3D ( 'NONE', #32756, #195346, #10595 ) ;
#201312=FACE_OUTER_BOUND ( 'NONE', #115229, .T. ) ;
#201316=CONICAL_SURFACE ( 'NONE', #109729, 4.299999999999956302, 0.7853981633974466137 ) ;
#201332=AXIS2_PLACEMENT_3D ( 'NONE', #104661, #134519, #176260 ) ;
#201367=ORIENTED_EDGE ( 'NONE', *, *, #241183, .T. ) ;
#201387=CARTESIAN_POINT ( 'NONE',  ( 21.05000000000000071, 0.000000000000000000, -12.15000000000000036 ) ) ;
#201390=ORIENTED_EDGE ( 'NONE', *, *, #19173, .T. ) ;
#201472=ORIENTED_EDGE ( 'NONE', *, *, #224893, .T. ) ;
#201473=LINE ( 'NONE', #103643, #65042 ) ;
#201474=EDGE_CURVE ( 'NONE', #84969, #211780, #211415, .T. ) ;
#201504=DIRECTION ( 'NONE',  ( 0.000000000000000000, -0.1350103645451876944, -0.9908441862701601321 ) ) ;
#201505=ORIENTED_EDGE ( 'NONE', *, *, #227408, .T. ) ;
#201524=EDGE_LOOP ( 'NONE', ( #108982, #47381, #26700, #78018 ) ) ;
#201527=CARTESIAN_POINT ( 'NONE',  ( -23.15000000000000213, 4.349999999999999645, -12.15000000000000391 ) ) ;
#201598=ORIENTED_EDGE ( 'NONE', *, *, #135325, .F. ) ;
#201602=CARTESIAN_POINT ( 'NONE',  ( 21.05000000000000071, 1.349084418627015447, -7.986498963545480834 ) ) ;
#201605=DIRECTION ( 'NONE',  ( 1.000000000000000000, 0.000000000000000000, -0.000000000000000000 ) ) ;
#201638=VERTEX_POINT ( 'NONE', #6569 ) ;
#201648=CARTESIAN_POINT ( 'NONE',  ( -20.94999999999999929, -11.48912529307605546, -30.39999999999999503 ) ) ;
#201662=CARTESIAN_POINT ( 'NONE',  ( 18.49999999999999289, 10.20857864376269575, 11.75000000000000000 ) ) ;
#201685=DIRECTION ( 'NONE',  ( 1.000000000000000000, -0.000000000000000000, -0.000000000000000000 ) ) ;
#201687=TOROIDAL_SURFACE ( 'NONE', #18532, 0.4000000000000005773, 0.1000000000000000056 ) ;
#201691=CIRCLE ( 'NONE', #51831, 11.70000000000000284 ) ;
#201698=FACE_OUTER_BOUND ( 'NONE', #80510, .T. ) ;
#201749=CARTESIAN_POINT ( 'NONE',  ( -21.14999999999999858, 6.257814610476114758, 0.09779029130879343668 ) ) ;
#201752=VERTEX_POINT ( 'NONE', #251603 ) ;
#201763=CARTESIAN_POINT ( 'NONE',  ( -18.59999999999999787, 3.912899247233453615, -11.48182297301096888 ) ) ;
#201764=EDGE_CURVE ( 'NONE', #94186, #77399, #219763, .T. ) ;
#201863=CARTESIAN_POINT ( 'NONE',  ( 22.48660254037844197, 11.65000000000000746, 0.04999999999999796274 ) ) ;
#201886=ORIENTED_EDGE ( 'NONE', *, *, #217165, .F. ) ;
#201903=EDGE_CURVE ( 'NONE', #43421, #106103, #78084, .T. ) ;
#201913=AXIS2_PLACEMENT_3D ( 'NONE', #187310, #132452, #13791 ) ;
#201945=DIRECTION ( 'NONE',  ( -0.000000000000000000, -0.1298341882519805091, -0.9915357197604881545 ) ) ;
#201999=CIRCLE ( 'NONE', #14772, 0.09999999999999939493 ) ;
#202026=CIRCLE ( 'NONE', #251902, 0.09999999999999993616 ) ;
#202043=CARTESIAN_POINT ( 'NONE',  ( -21.33487959338958362, 6.725558151911188887, -1.166372555419965823E-16 ) ) ;
#202048=ORIENTED_EDGE ( 'NONE', *, *, #127259, .F. ) ;
#202071=FACE_OUTER_BOUND ( 'NONE', #102455, .T. ) ;
#202078=ORIENTED_EDGE ( 'NONE', *, *, #1009, .F. ) ;
#202106=EDGE_CURVE ( 'NONE', #118795, #70529, #228353, .T. ) ;
#202111=VERTEX_POINT ( 'NONE', #3687 ) ;
#202118=CARTESIAN_POINT ( 'NONE',  ( 20.94999999999999574, 1.162701749938009677, -8.099999999999999645 ) ) ;
#202141=STYLED_ITEM ( 'NONE', ( #209229 ), #104549 ) ;
#202142=AXIS2_PLACEMENT_3D ( 'NONE', #39087, #242389, #200709 ) ;
#202154=LINE ( 'NONE', #166915, #56468 ) ;
#202160=VERTEX_POINT ( 'NONE', #72682 ) ;
#202177=AXIS2_PLACEMENT_3D ( 'NONE', #117127, #58396, #79250 ) ;
#202187=AXIS2_PLACEMENT_3D ( 'NONE', #148537, #186387, #85952 ) ;
#202199=ORIENTED_EDGE ( 'NONE', *, *, #97858, .T. ) ;
#202203=VECTOR ( 'NONE', #96926, 1000.000000000000000 ) ;
#202221=EDGE_CURVE ( 'NONE', #131644, #223333, #195037, .T. ) ;
#202242=VERTEX_POINT ( 'NONE', #188743 ) ;
#202243=ADVANCED_FACE ( 'NONE', ( #93491 ), #40932, .T. ) ;
#202246=EDGE_LOOP ( 'NONE', ( #204335, #37824, #12746 ) ) ;
#202270=DIRECTION ( 'NONE',  ( 0.000000000000000000, 1.000000000000000000, 0.000000000000000000 ) ) ;
#202295=FACE_OUTER_BOUND ( 'NONE', #82870, .T. ) ;
#202299=ORIENTED_EDGE ( 'NONE', *, *, #136424, .F. ) ;
#202301=DIRECTION ( 'NONE',  ( 1.000000000000000000, 0.000000000000000000, 0.000000000000000000 ) ) ;
#202302=CARTESIAN_POINT ( 'NONE',  ( -21.05000000000000071, 11.59999999999999964, -26.57179676972449656 ) ) ;
#202324=DIRECTION ( 'NONE',  ( 1.000000000000000000, 0.000000000000000000, 0.000000000000000000 ) ) ;
#202356=CARTESIAN_POINT ( 'NONE',  ( -23.25000000000000000, -9.599999999999997868, -23.60603087734755690 ) ) ;
#202366=EDGE_CURVE ( 'NONE', #31072, #209903, #120047, .T. ) ;
#202368=ORIENTED_EDGE ( 'NONE', *, *, #218835, .T. ) ;
#202415=DIRECTION ( 'NONE',  ( -0.000000000000000000, 0.000000000000000000, -1.000000000000000000 ) ) ;
#202473=ADVANCED_FACE ( 'NONE', ( #131027 ), #108892, .F. ) ;
#202541=CIRCLE ( 'NONE', #256462, 0.09999999999999971412 ) ;
#202559=CIRCLE ( 'NONE', #131645, 0.1000000000000008937 ) ;
#202569=CARTESIAN_POINT ( 'NONE',  ( -21.05000000000000071, 5.899999999999947065, -10.21909976465641456 ) ) ;
#202573=CARTESIAN_POINT ( 'NONE',  ( -23.15000000000000213, 11.75000000000000000, -26.48519422934605672 ) ) ;
#202579=CARTESIAN_POINT ( 'NONE',  ( -18.55121869061588669, 10.32747123226657493, -39.07740328502493554 ) ) ;
#202602=DIRECTION ( 'NONE',  ( 0.000000000000000000, -0.9908441862701596881, -0.1350103645451904977 ) ) ;
#202612=AXIS2_PLACEMENT_3D ( 'NONE', #200312, #141613, #221141 ) ;
#202651=EDGE_CURVE ( 'NONE', #176398, #234302, #178679, .T. ) ;
#202657=CIRCLE ( 'NONE', #98555, 0.1000000000000028644 ) ;
#202690=EDGE_LOOP ( 'NONE', ( #241669, #141215, #146328, #245776 ) ) ;
#202739=EDGE_CURVE ( 'NONE', #23245, #166638, #245285, .T. ) ;
#202741=AXIS2_PLACEMENT_3D ( 'NONE', #95762, #158367, #237863 ) ;
#202779=ORIENTED_EDGE ( 'NONE', *, *, #155228, .T. ) ;
#202802=EDGE_LOOP ( 'NONE', ( #152808, #174993, #251856, #8758 ) ) ;
#202834=AXIS2_PLACEMENT_3D ( 'NONE', #186427, #29929, #31234 ) ;
#202931=DIRECTION ( 'NONE',  ( 0.000000000000000000, 0.000000000000000000, 1.000000000000000000 ) ) ;
#202948=DIRECTION ( 'NONE',  ( 0.000000000000000000, -0.1350103645451876666, 0.9908441862701600211 ) ) ;
#202952=CIRCLE ( 'NONE', #236276, 12.77499999999999858 ) ;
#202997=AXIS2_PLACEMENT_3D ( 'NONE', #218980, #179883, #255497 ) ;
#203009=FACE_OUTER_BOUND ( 'NONE', #136138, .T. ) ;
#203042=EDGE_CURVE ( 'NONE', #64464, #243852, #237088, .T. ) ;
#203061=LINE ( 'NONE', #27030, #205705 ) ;
#203063=EDGE_CURVE ( 'NONE', #142144, #253366, #45753, .T. ) ;
#203076=EDGE_LOOP ( 'NONE', ( #248513, #133512, #231196, #84666 ) ) ;
#203092=ADVANCED_FACE ( 'NONE', ( #139700 ), #141020, .T. ) ;
#203148=ORIENTED_EDGE ( 'NONE', *, *, #174858, .T. ) ;
#203187=CIRCLE ( 'NONE', #182359, 0.09999999999999939493 ) ;
#203222=CARTESIAN_POINT ( 'NONE',  ( -21.05000000000000071, 5.850000000000001421, -23.36750277572207679 ) ) ;
#203253=CIRCLE ( 'NONE', #40966, 0.1000000000000007272 ) ;
#203264=CARTESIAN_POINT ( 'NONE',  ( -20.94999999999999929, -1.162701749938009677, -8.099999999999999645 ) ) ;
#203277=CIRCLE ( 'NONE', #257368, 0.1000000000000016986 ) ;
#203286=EDGE_CURVE ( 'NONE', #32887, #128006, #207419, .T. ) ;
#203288=FACE_OUTER_BOUND ( 'NONE', #229519, .T. ) ;
#203297=PRODUCT ( 'Injection Molded Chain Links', 'Injection Molded Chain Links', '', ( #157797 ) ) ;
#203330=CARTESIAN_POINT ( 'NONE',  ( -18.50000000000000000, -26.43935341560094443, -18.14150860750746475 ) ) ;
#203335=DIRECTION ( 'NONE',  ( 1.000000000000000000, 3.265361837132813093E-16, -0.000000000000000000 ) ) ;
#203337=AXIS2_PLACEMENT_3D ( 'NONE', #211933, #131094, #136195 ) ;
#203392=CARTESIAN_POINT ( 'NONE',  ( -18.59999999999999787, -1.835341550224411922, -11.65515129256297833 ) ) ;
#203452=CARTESIAN_POINT ( 'NONE',  ( -20.64999999999999858, -9.400000000000005684, -9.893969122652444881 ) ) ;
#203463=EDGE_CURVE ( 'NONE', #130496, #214472, #137296, .T. ) ;
#203501=FACE_OUTER_BOUND ( 'NONE', #218931, .T. ) ;
#203544=CARTESIAN_POINT ( 'NONE',  ( -23.15000000000000213, 11.65000000000000036, 11.75000000000000000 ) ) ;
#203556=CARTESIAN_POINT ( 'NONE',  ( 20.85000000000000142, 11.65000000000000391, -26.71613433702190932 ) ) ;
#203570=ADVANCED_FACE ( 'NONE', ( #187224 ), #225020, .T. ) ;
#203572=DIRECTION ( 'NONE',  ( 1.000000000000000000, 0.000000000000000000, 0.000000000000000000 ) ) ;
#203579=AXIS2_PLACEMENT_3D ( 'NONE', #37095, #95735, #256053 ) ;
#203621=DIRECTION ( 'NONE',  ( 1.000000000000000000, 0.000000000000000000, 0.000000000000000000 ) ) ;
#203634=CARTESIAN_POINT ( 'NONE',  ( -23.25000000000000000, 0.000000000000000000, -33.50000000000000000 ) ) ;
#203662=ADVANCED_FACE ( 'NONE', ( #68546 ), #28653, .T. ) ;
#203669=ORIENTED_EDGE ( 'NONE', *, *, #229525, .T. ) ;
#203684=CARTESIAN_POINT ( 'NONE',  ( -20.90851465518106167, 10.32532329026770590, -39.06993430183595706 ) ) ;
#203727=AXIS2_PLACEMENT_3D ( 'NONE', #160087, #98762, #255256 ) ;
#203746=ORIENTED_EDGE ( 'NONE', *, *, #133585, .F. ) ;
#203773=CARTESIAN_POINT ( 'NONE',  ( -20.54999999999999716, -9.000000000000001776, -23.60603087734756045 ) ) ;
#203805=TOROIDAL_SURFACE ( 'NONE', #174832, 11.65000000000000036, 0.1000000000000000056 ) ;
#203811=DIRECTION ( 'NONE',  ( 0.000000000000000000, 1.265107689135680095E-16, -1.000000000000000000 ) ) ;
#203825=CARTESIAN_POINT ( 'NONE',  ( -20.64999999999999858, 1.999999999999998224, -20.27537807723789953 ) ) ;
#203862=CARTESIAN_POINT ( 'NONE',  ( -21.04386569057570355, 11.74999999999978506, -26.64283735177988532 ) ) ;
#203893=ADVANCED_FACE ( 'NONE', ( #166084 ), #145288, .F. ) ;
#203959=EDGE_LOOP ( 'NONE', ( #223121, #25134 ) ) ;
#203968=CIRCLE ( 'NONE', #150021, 0.5000000000000022204 ) ;
#203969=VERTEX_POINT ( 'NONE', #91649 ) ;
#203978=PLANE ( 'NONE',  #10955 ) ;
#203993=TOROIDAL_SURFACE ( 'NONE', #79071, 11.70000000000000639, 0.1000000000000000056 ) ;
#204016=CYLINDRICAL_SURFACE ( 'NONE', #223470, 0.09999999999999939493 ) ;
#204030=CARTESIAN_POINT ( 'NONE',  ( 20.94999999999999574, 6.550000000000003375, -9.843822089683131438 ) ) ;
#204077=CARTESIAN_POINT ( 'NONE',  ( 20.85000000000000142, -11.64999999999999147, -30.59999999999999432 ) ) ;
#204087=VECTOR ( 'NONE', #46052, 1000.000000000000000 ) ;
#204093=ORIENTED_EDGE ( 'NONE', *, *, #212736, .F. ) ;
#204096=EDGE_CURVE ( 'NONE', #101735, #219381, #24719, .T. ) ;
#204130=EDGE_LOOP ( 'NONE', ( #143243, #8791, #62478, #81816 ) ) ;
#204171=EDGE_LOOP ( 'NONE', ( #188634, #43088, #53507, #108114 ) ) ;
#204204=EDGE_CURVE ( 'NONE', #82492, #44319, #153736, .T. ) ;
#204209=CARTESIAN_POINT ( 'NONE',  ( -20.85000000000000142, -1.736705739467587772, -45.01742258762372728 ) ) ;
#204256=DIRECTION ( 'NONE',  ( 0.000000000000000000, 1.000000000000000000, 0.000000000000000000 ) ) ;
#204262=CARTESIAN_POINT ( 'NONE',  ( -23.25000000000000000, 11.75000000000000000, 11.75000000000000000 ) ) ;
#204263=CARTESIAN_POINT ( 'NONE',  ( -18.59999996769639097, -9.363273769830332327, -7.181493915465814837 ) ) ;
#204286=DIRECTION ( 'NONE',  ( 0.000000000000000000, -1.000000000000000000, 0.000000000000000000 ) ) ;
#204299=PRODUCT_DEFINITION_CONTEXT ( 'detailed design', #24210, 'design' ) ;
#204308=EDGE_CURVE ( 'NONE', #52704, #184931, #181473, .T. ) ;
#204325=EDGE_CURVE ( 'NONE', #253599, #19453, #174584, .T. ) ;
#204335=ORIENTED_EDGE ( 'NONE', *, *, #150204, .T. ) ;
#204338=AXIS2_PLACEMENT_3D ( 'NONE', #125447, #249248, #204953 ) ;
#204345=CARTESIAN_POINT ( 'NONE',  ( -21.03922262424671885, 11.62390063400470375, -6.859208042893458313 ) ) ;
#204463=CARTESIAN_POINT ( 'NONE',  ( -23.25000000000000000, -11.75000000000000000, -30.39999999999999858 ) ) ;
#204478=DIRECTION ( 'NONE',  ( 1.000000000000000000, 0.000000000000000000, -3.469446951953635015E-14 ) ) ;
#204537=ADVANCED_FACE ( 'NONE', ( #256778 ), #241358, .T. ) ;
#204557=AXIS2_PLACEMENT_3D ( 'NONE', #67130, #64556, #45002 ) ;
#204566=ORIENTED_EDGE ( 'NONE', *, *, #89613, .T. ) ;
#204571=CARTESIAN_POINT ( 'NONE',  ( -23.15000000000000213, -9.000000000000001776, -23.60603087734756045 ) ) ;
#204578=CARTESIAN_POINT ( 'NONE',  ( -21.05000000000000071, 0.000000000000000000, -21.80000000000000071 ) ) ;
#204628=ORIENTED_EDGE ( 'NONE', *, *, #146797, .T. ) ;
#204641=AXIS2_PLACEMENT_3D ( 'NONE', #154876, #117003, #56994 ) ;
#204670=DIRECTION ( 'NONE',  ( -1.000000000000000000, 0.000000000000000000, 0.000000000000000000 ) ) ;
#204697=AXIS2_PLACEMENT_3D ( 'NONE', #65609, #99573, #179173 ) ;
#204703=EDGE_LOOP ( 'NONE', ( #41076, #130649, #233931, #245826, #183737, #223969, #172677, #13181, #125793, #64655 ) ) ;
#204718=DIRECTION ( 'NONE',  ( 1.000000000000000000, 0.000000000000000000, 0.000000000000000000 ) ) ;
#204721=AXIS2_PLACEMENT_3D ( 'NONE', #20880, #198199, #139497 ) ;
#204728=CARTESIAN_POINT ( 'NONE',  ( -20.00857864376270001, 9.150000000000002132, -21.25000000000000000 ) ) ;
#204739=VERTEX_POINT ( 'NONE', #127601 ) ;
#204746=EDGE_LOOP ( 'NONE', ( #145262, #216452, #28134, #44417, #148270, #105255 ) ) ;
#204776=VERTEX_POINT ( 'NONE', #185005 ) ;
#204789=AXIS2_PLACEMENT_3D ( 'NONE', #184400, #48742, #187004 ) ;
#204796=FACE_OUTER_BOUND ( 'NONE', #87328, .T. ) ;
#204850=CARTESIAN_POINT ( 'NONE',  ( -23.15000000000000213, 11.75000000000000000, -12.24999999999999822 ) ) ;
#204862=DIRECTION ( 'NONE',  ( -1.000000000000000000, -0.000000000000000000, -0.000000000000000000 ) ) ;
#204879=CYLINDRICAL_SURFACE ( 'NONE', #248401, 0.5000000000000022204 ) ;
#204881=DIRECTION ( 'NONE',  ( 0.000000000000000000, 0.1350103645451876666, -0.9908441862701600211 ) ) ;
#204900=CYLINDRICAL_SURFACE ( 'NONE', #45770, 0.1000000000000000472 ) ;
#204936=FACE_OUTER_BOUND ( 'NONE', #24147, .T. ) ;
#204946=FACE_OUTER_BOUND ( 'NONE', #83098, .T. ) ;
#204949=AXIS2_PLACEMENT_3D ( 'NONE', #97098, #39769, #585 ) ;
#204953=DIRECTION ( 'NONE',  ( 0.000000000000000000, 0.000000000000000000, 1.000000000000000000 ) ) ;
#204962=DIRECTION ( 'NONE',  ( 1.000000000000000000, 0.000000000000000000, 0.000000000000000000 ) ) ;
#205025=CARTESIAN_POINT ( 'NONE',  ( 21.05000000000000071, -11.48912529307605546, -30.39999999999999503 ) ) ;
#205027=DIRECTION ( 'NONE',  ( 0.000000000000000000, 0.000000000000000000, -1.000000000000000000 ) ) ;
#205033=EDGE_LOOP ( 'NONE', ( #163492, #112671, #12023, #110790 ) ) ;
#205037=CIRCLE ( 'NONE', #138575, 0.5999999999999998668 ) ;
#205044=EDGE_CURVE ( 'NONE', #26537, #61614, #95757, .T. ) ;
#205060=CIRCLE ( 'NONE', #75918, 0.1000000000000012407 ) ;
#205063=CIRCLE ( 'NONE', #34255, 0.1000000000000002554 ) ;
#205074=CARTESIAN_POINT ( 'NONE',  ( 18.59999999999999076, 6.649999999999999467, -21.15000000000000213 ) ) ;
#205082=DIRECTION ( 'NONE',  ( -1.000000000000000000, 0.000000000000000000, 0.000000000000000000 ) ) ;
#205127=DIRECTION ( 'NONE',  ( 0.7071067811865388020, -0.7071067811865561215, 0.000000000000000000 ) ) ;
#205137=VECTOR ( 'NONE', #93276, 1000.000000000000000 ) ;
#205173=CYLINDRICAL_SURFACE ( 'NONE', #98922, 0.09999999999999971412 ) ;
#205181=CIRCLE ( 'NONE', #255016, 4.049999999999998934 ) ;
#205182=CIRCLE ( 'NONE', #92767, 0.09999999999999949207 ) ;
#205202=DIRECTION ( 'NONE',  ( -0.000000000000000000, 0.000000000000000000, 1.000000000000000000 ) ) ;
#205223=DIRECTION ( 'NONE',  ( 0.000000000000000000, 0.000000000000000000, -1.000000000000000000 ) ) ;
#205252=DIRECTION ( 'NONE',  ( 0.000000000000000000, 0.8660254037844411501, 0.4999999999999956701 ) ) ;
#205275=ADVANCED_FACE ( 'NONE', ( #149422 ), #150154, .T. ) ;
#205304=VERTEX_POINT ( 'NONE', #191120 ) ;
#205314=DIRECTION ( 'NONE',  ( 1.000000000000000000, 3.265361837132813093E-16, -0.000000000000000000 ) ) ;
#205334=DIRECTION ( 'NONE',  ( 0.000000000000000000, -0.9908441862701596881, 0.1350103645451904977 ) ) ;
#205336=AXIS2_PLACEMENT_3D ( 'NONE', #93817, #173418, #74298 ) ;
#205411=DIRECTION ( 'NONE',  ( 1.000000000000000000, 0.000000000000000000, 0.000000000000000000 ) ) ;
#205418=CARTESIAN_POINT ( 'NONE',  ( -22.39999999999999503, 7.790779598373403836, 0.09999999999999939493 ) ) ;
#205430=CARTESIAN_POINT ( 'NONE',  ( -23.25000000000000000, -0.09999999999999939493, 11.64957080754479968 ) ) ;
#205454=EDGE_LOOP ( 'NONE', ( #208652, #139231, #235674, #142475 ) ) ;
#205460=CARTESIAN_POINT ( 'NONE',  ( 23.24999999999999289, 11.75000000000000711, 11.75000000000000000 ) ) ;
#205461=CARTESIAN_POINT ( 'NONE',  ( 21.05000000000000071, 10.72371710470752149, -7.664913569087605794 ) ) ;
#205494=EDGE_CURVE ( 'NONE', #84065, #239961, #183642, .T. ) ;
#205514=CARTESIAN_POINT ( 'NONE',  ( 23.25000000000000000, -9.000000000000001776, -9.893969122652443104 ) ) ;
#205522=VECTOR ( 'NONE', #121493, 1000.000000000000000 ) ;
#205545=CARTESIAN_POINT ( 'NONE',  ( -18.60000000000000142, -9.321008403361288330, -7.235938249077881856 ) ) ;
#205547=LINE ( 'NONE', #247244, #147537 ) ;
#205551=ADVANCED_FACE ( 'NONE', ( #83928 ), #44860, .T. ) ;
#205560=ORIENTED_EDGE ( 'NONE', *, *, #175685, .F. ) ;
#205586=CARTESIAN_POINT ( 'NONE',  ( 21.05000000000000071, 0.000000000000000000, -33.50000000000000000 ) ) ;
#205626=CARTESIAN_POINT ( 'NONE',  ( -21.14999999893415250, 11.74999999999999645, -6.844495343526469711 ) ) ;
#205666=DIRECTION ( 'NONE',  ( -2.602085213965226419E-14, -0.000000000000000000, -1.000000000000000000 ) ) ;
#205672=LINE ( 'NONE', #27086, #226885 ) ;
#205696=AXIS2_PLACEMENT_3D ( 'NONE', #214560, #137579, #17642 ) ;
#205705=VECTOR ( 'NONE', #24461, 1000.000000000000000 ) ;
#205718=ORIENTED_EDGE ( 'NONE', *, *, #230827, .F. ) ;
#205730=CARTESIAN_POINT ( 'NONE',  ( 20.94999999999999929, 4.850467289719620823, -21.46573259099832498 ) ) ;
#205741=DIRECTION ( 'NONE',  ( 0.000000000000000000, -0.7397360091702744889, 0.6728971962616842051 ) ) ;
#205780=AXIS2_PLACEMENT_3D ( 'NONE', #105343, #88360, #87081 ) ;
#205802=DIRECTION ( 'NONE',  ( 1.000000000000000000, 0.000000000000000000, 0.000000000000000000 ) ) ;
#205847=ORIENTED_EDGE ( 'NONE', *, *, #164570, .T. ) ;
#205863=CARTESIAN_POINT ( 'NONE',  ( 21.14999999999999858, 10.71339244339988461, -12.35000000000000142 ) ) ;
#205869=CARTESIAN_POINT ( 'NONE',  ( 22.47007471830798409, 7.720710651926455448, -9.757819552369539906E-16 ) ) ;
#205875=ORIENTED_EDGE ( 'NONE', *, *, #66151, .T. ) ;
#205897=AXIS2_PLACEMENT_3D ( 'NONE', #49785, #141494, #87610 ) ;
#205936=CIRCLE ( 'NONE', #164261, 0.1999999999999987899 ) ;
#205947=DIRECTION ( 'NONE',  ( 1.000000000000000000, 0.000000000000000000, 0.000000000000000000 ) ) ;
#205958=CARTESIAN_POINT ( 'NONE',  ( -20.54999999999999716, 1.999999999999998224, -12.72462192276209869 ) ) ;
#205963=ORIENTED_EDGE ( 'NONE', *, *, #73238, .T. ) ;
#205974=ORIENTED_EDGE ( 'NONE', *, *, #218740, .T. ) ;
#205991=DIRECTION ( 'NONE',  ( 0.000000000000000000, 0.000000000000000000, -1.000000000000000000 ) ) ;
#206011=AXIS2_PLACEMENT_3D ( 'NONE', #249204, #155261, #234761 ) ;
#206016=CARTESIAN_POINT ( 'NONE',  ( -21.59780538579341425, 6.847090529943250736, 0.09897866959798369557 ) ) ;
#206018=VERTEX_POINT ( 'NONE', #71841 ) ;
#206032=DIRECTION ( 'NONE',  ( 1.000000000000000000, 0.000000000000000000, 0.000000000000000000 ) ) ;
#206052=ORIENTED_EDGE ( 'NONE', *, *, #244603, .T. ) ;
#206077=FACE_OUTER_BOUND ( 'NONE', #210774, .T. ) ;
#206101=CARTESIAN_POINT ( 'NONE',  ( -23.15000000000000213, 11.59999999999999964, -26.57179676972450011 ) ) ;
#206113=DIRECTION ( 'NONE',  ( -1.000000000000000000, -0.000000000000000000, 0.000000000000000000 ) ) ;
#206122=PLANE ( 'NONE',  #64501 ) ;
#206135=CARTESIAN_POINT ( 'NONE',  ( -18.45068461519105796, -9.486506529089087536, -7.068777168904707864 ) ) ;
#206157=DIRECTION ( 'NONE',  ( 0.000000000000000000, 1.224646799147363807E-16, 1.000000000000000000 ) ) ;
#206203=DIRECTION ( 'NONE',  ( 0.000000000000000000, 0.000000000000000000, -1.000000000000000000 ) ) ;
#206208=B_SPLINE_CURVE_WITH_KNOTS ( 'NONE', 3,
 ( #156051, #175602, #118182, #255052, #235546, #257621, #157339, #16529, #236830, #20384 ),
 .UNSPECIFIED., .F., .F.,
 ( 4, 3, 3, 4 ),
 ( 0.000000000000000000, 3.394313611810755905E-05, 6.779740500699913091E-05, 0.0001049857339142649037 ),
 .UNSPECIFIED. ) ;
#206215=ORIENTED_EDGE ( 'NONE', *, *, #242833, .F. ) ;
#206232=VERTEX_POINT ( 'NONE', #118672 ) ;
#206262=CARTESIAN_POINT ( 'NONE',  ( 20.94999999999999574, -11.48912529307605901, -3.100000000000000533 ) ) ;
#206270=CARTESIAN_POINT ( 'NONE',  ( -20.54999999999999716, 4.349999999999999645, -21.14999999999999858 ) ) ;
#206308=CIRCLE ( 'NONE', #218750, 0.5000000000000022204 ) ;
#206347=ORIENTED_EDGE ( 'NONE', *, *, #98569, .T. ) ;
#206348=DIRECTION ( 'NONE',  ( 0.000000000000000000, 0.000000000000000000, 1.000000000000000000 ) ) ;
#206355=CIRCLE ( 'NONE', #6421, 0.8750000000000007772 ) ;
#206375=VECTOR ( 'NONE', #65671, 1000.000000000000000 ) ;
#206381=CARTESIAN_POINT ( 'NONE',  ( -21.05000000000000071, 14.05000000000000071, -5.513695070760990191 ) ) ;
#206388=CARTESIAN_POINT ( 'NONE',  ( 23.25000000000000000, -9.600000000000001421, -23.60603087734755690 ) ) ;
#206415=DIRECTION ( 'NONE',  ( 0.000000000000000000, 0.000000000000000000, -1.000000000000000000 ) ) ;
#206419=DIRECTION ( 'NONE',  ( 1.000000000000000000, 0.000000000000000000, 0.000000000000000000 ) ) ;
#206461=CARTESIAN_POINT ( 'NONE',  ( 20.94560253601876809, 11.75000000000000355, -26.51008351251537576 ) ) ;
#206464=CARTESIAN_POINT ( 'NONE',  ( -18.59999999999999787, 11.75000000000000000, -33.50000000000000000 ) ) ;
#206470=AXIS2_PLACEMENT_3D ( 'NONE', #128017, #70635, #144984 ) ;
#206472=ORIENTED_EDGE ( 'NONE', *, *, #77688, .F. ) ;
#206488=DIRECTION ( 'NONE',  ( 1.000000000000000000, 0.000000000000000000, 0.000000000000000000 ) ) ;
#206517=CARTESIAN_POINT ( 'NONE',  ( -20.95000000000000284, 11.64999999999999680, -26.48519422934605316 ) ) ;
#206544=DIRECTION ( 'NONE',  ( -1.000000000000000000, -3.265361837132813093E-16, 0.000000000000000000 ) ) ;
#206578=CARTESIAN_POINT ( 'NONE',  ( 18.53317502108576420, 10.32263460346244166, -39.06059579686719729 ) ) ;
#206582=DIRECTION ( 'NONE',  ( -1.000000000000000000, 0.000000000000000000, 0.000000000000000000 ) ) ;
#206602=EDGE_CURVE ( 'NONE', #253366, #124163, #250777, .T. ) ;
#206613=DIRECTION ( 'NONE',  ( 0.000000000000000000, 0.000000000000000000, -1.000000000000000000 ) ) ;
#206628=EDGE_CURVE ( 'NONE', #106788, #103673, #25742, .T. ) ;
#206632=( BOUNDED_SURFACE ( )  B_SPLINE_SURFACE ( 3, 2, ( 
 ( #13884, #54274, #192522 ),
 ( #56818, #232952, #93404 ),
 ( #136354, #133819, #214632 ),
 ( #213346, #37311, #34755 ) ),
 .UNSPECIFIED., .F., .F., .T. ) 
 B_SPLINE_SURFACE_WITH_KNOTS ( ( 4, 4 ),
 ( 3, 3 ),
 ( -1.734723475976807094E-18, 0.001979672783031532438 ),
 ( 0.000000000000000000, 1.000000000000000000 ),
 .UNSPECIFIED. ) 
 GEOMETRIC_REPRESENTATION_ITEM ( )  RATIONAL_B_SPLINE_SURFACE ( (
 ( 1.000000000000000000, 0.7103081912008197829, 1.000000000000000000),
 ( 1.000000000000000000, 0.7104998333558695256, 1.000000000000000000),
 ( 1.000000000000000000, 0.7107238315755238789, 1.000000000000000000),
 ( 1.000000000000000000, 0.7110073749539377319, 1.000000000000000000) ) ) 
 REPRESENTATION_ITEM ( '' )  SURFACE ( )  );
#206637=DIRECTION ( 'NONE',  ( 1.000000000000000000, 7.304098846218134667E-16, 0.000000000000000000 ) ) ;
#206677=DIRECTION ( 'NONE',  ( 1.734723475976817507E-14, -1.000000000000000000, 0.000000000000000000 ) ) ;
#206681=CARTESIAN_POINT ( 'NONE',  ( -20.94999999999999929, -11.65000000000000036, -33.50000000000000000 ) ) ;
#206715=CIRCLE ( 'NONE', #111048, 0.09999999999999961697 ) ;
#206748=ORIENTED_EDGE ( 'NONE', *, *, #177489, .T. ) ;
#206756=ORIENTED_EDGE ( 'NONE', *, *, #239243, .T. ) ;
#206760=CIRCLE ( 'NONE', #23819, 0.1000000000000002554 ) ;
#206777=DIRECTION ( 'NONE',  ( 0.7071359030027766224, -0.7070776581709024011, 0.000000000000000000 ) ) ;
#206803=CARTESIAN_POINT ( 'NONE',  ( 20.85882249326303040, 10.33248238082519066, -39.09484654391314962 ) ) ;
#206824=DIRECTION ( 'NONE',  ( 1.000000000000000000, 0.000000000000000000, 0.000000000000000000 ) ) ;
#206825=CIRCLE ( 'NONE', #94378, 0.1000000000000012407 ) ;
#206827=VECTOR ( 'NONE', #36293, 1000.000000000000000 ) ;
#206831=AXIS2_PLACEMENT_3D ( 'NONE', #29388, #188415, #9777 ) ;
#206849=CARTESIAN_POINT ( 'NONE',  ( -18.45037301276663300, -9.490200447541971229, -7.012674136414320358 ) ) ;
#206875=AXIS2_PLACEMENT_3D ( 'NONE', #181112, #201945, #218917 ) ;
#206888=VECTOR ( 'NONE', #249057, 1000.000000000000000 ) ;
#206893=DIRECTION ( 'NONE',  ( 0.000000000000000000, 0.01562499999998609446, -0.9998779222360101304 ) ) ;
#206899=CARTESIAN_POINT ( 'NONE',  ( -18.50000000000000000, 0.000000000000000000, -33.50000000000000000 ) ) ;
#206916=CIRCLE ( 'NONE', #131905, 11.65000000000000036 ) ;
#206926=ADVANCED_FACE ( 'NONE', ( #204936 ), #25062, .F. ) ;
#206947=ORIENTED_EDGE ( 'NONE', *, *, #153466, .F. ) ;
#206952=CARTESIAN_POINT ( 'NONE',  ( 20.85000000000000142, 6.846123162352588665, -37.23772626684986164 ) ) ;
#206957=DIRECTION ( 'NONE',  ( -1.000000000000000000, 0.000000000000000000, -0.000000000000000000 ) ) ;
#207038=CYLINDRICAL_SURFACE ( 'NONE', #176018, 11.75000000000000000 ) ;
#207059=ORIENTED_EDGE ( 'NONE', *, *, #17698, .F. ) ;
#207063=AXIS2_PLACEMENT_3D ( 'NONE', #80580, #97575, #237123 ) ;
#207071=AXIS2_PLACEMENT_3D ( 'NONE', #138039, #160219, #175930 ) ;
#207083=CARTESIAN_POINT ( 'NONE',  ( 21.05000000000000071, 0.000000000000000000, -12.87500000000000000 ) ) ;
#207105=VERTEX_POINT ( 'NONE', #92698 ) ;
#207155=ADVANCED_FACE ( 'NONE', ( #116138 ), #250937, .F. ) ;
#207190=ADVANCED_FACE ( 'NONE', ( #28421 ), #167921, .T. ) ;
#207211=ORIENTED_EDGE ( 'NONE', *, *, #226737, .F. ) ;
#207246=CARTESIAN_POINT ( 'NONE',  ( -20.54999999999999716, 7.150000000000000355, -21.15000000000000213 ) ) ;
#207283=SPHERICAL_SURFACE ( 'NONE', #28165, 0.1000000000000000056 ) ;
#207284=CARTESIAN_POINT ( 'NONE',  ( -22.59066674512250472, 11.75000000000000000, 0.03050412363058079002 ) ) ;
#207303=EDGE_CURVE ( 'NONE', #57548, #53632, #196783, .T. ) ;
#207307=DIRECTION ( 'NONE',  ( -1.000000000000000000, -3.265361837132813093E-16, 0.000000000000000000 ) ) ;
#207311=ORIENTED_EDGE ( 'NONE', *, *, #44445, .F. ) ;
#207332=DIRECTION ( 'NONE',  ( 0.000000000000000000, 0.000000000000000000, 1.000000000000000000 ) ) ;
#207337=VERTEX_POINT ( 'NONE', #66423 ) ;
#207341=DIRECTION ( 'NONE',  ( 0.000000000000000000, 0.000000000000000000, -1.000000000000000000 ) ) ;
#207350=VERTEX_POINT ( 'NONE', #3878 ) ;
#207388=DIRECTION ( 'NONE',  ( 0.000000000000000000, -0.01283462868041981321, -0.9999176327611367654 ) ) ;
#207400=DIRECTION ( 'NONE',  ( 0.000000000000000000, 1.000000000000000000, 0.000000000000000000 ) ) ;
#207415=CARTESIAN_POINT ( 'NONE',  ( 23.14999999999999858, 5.900000000000005684, -23.28090023534362629 ) ) ;
#207419=LINE ( 'NONE', #69201, #33292 ) ;
#207446=ORIENTED_EDGE ( 'NONE', *, *, #92123, .F. ) ;
#207483=FACE_OUTER_BOUND ( 'NONE', #23939, .T. ) ;
#207498=DIRECTION ( 'NONE',  ( 0.000000000000000000, 5.329070518200751394E-15, 1.000000000000000000 ) ) ;
#207502=EDGE_CURVE ( 'NONE', #15628, #86491, #113590, .T. ) ;
#207506=CYLINDRICAL_SURFACE ( 'NONE', #105467, 0.09999999999999939493 ) ;
#207508=ORIENTED_EDGE ( 'NONE', *, *, #201764, .T. ) ;
#207511=VECTOR ( 'NONE', #222169, 1000.000000000000000 ) ;
#207533=ORIENTED_EDGE ( 'NONE', *, *, #54355, .T. ) ;
#207548=CARTESIAN_POINT ( 'NONE',  ( 21.05000000000000071, 4.813084112149524252, -11.94151775652382419 ) ) ;
#207550=ORIENTED_EDGE ( 'NONE', *, *, #214391, .T. ) ;
#207567=VECTOR ( 'NONE', #57395, 1000.000000000000000 ) ;
#207571=AXIS2_PLACEMENT_3D ( 'NONE', #95083, #92507, #130347 ) ;
#207599=DIRECTION ( 'NONE',  ( 1.000000000000000000, 3.265361837132813093E-16, -0.000000000000000000 ) ) ;
#207602=DIRECTION ( 'NONE',  ( 1.000000000000000000, 0.000000000000000000, 0.000000000000000000 ) ) ;
#207620=ORIENTED_EDGE ( 'NONE', *, *, #162551, .T. ) ;
#207678=CARTESIAN_POINT ( 'NONE',  ( -20.94999999999999929, -11.48912529307605546, -30.59999999999999432 ) ) ;
#207698=VERTEX_POINT ( 'NONE', #41434 ) ;
#207704=ORIENTED_EDGE ( 'NONE', *, *, #146748, .F. ) ;
#207771=CIRCLE ( 'NONE', #82796, 7.720710678118662962 ) ;
#207795=AXIS2_PLACEMENT_3D ( 'NONE', #234365, #76579, #151000 ) ;
#207805=DIRECTION ( 'NONE',  ( -0.000000000000000000, -1.000000000000000000, 6.308085367188393199E-16 ) ) ;
#207821=ORIENTED_EDGE ( 'NONE', *, *, #23538, .F. ) ;
#207852=ORIENTED_EDGE ( 'NONE', *, *, #207303, .T. ) ;
#207868=DIRECTION ( 'NONE',  ( 0.000000000000000000, -0.9908441862701596881, -0.1350103645451904977 ) ) ;
#207872=VECTOR ( 'NONE', #15065, 1000.000000000000227 ) ;
#207881=ORIENTED_EDGE ( 'NONE', *, *, #192484, .T. ) ;
#207887=EDGE_CURVE ( 'NONE', #126780, #157985, #76327, .T. ) ;
#207919=LINE ( 'NONE', #146614, #243556 ) ;
#207954=CARTESIAN_POINT ( 'NONE',  ( -20.00857864376270001, 9.350000000000001421, -21.15000000000000213 ) ) ;
#207961=DIRECTION ( 'NONE',  ( 0.000000000000000000, 0.000000000000000000, -1.000000000000000000 ) ) ;
#207967=ORIENTED_EDGE ( 'NONE', *, *, #60005, .F. ) ;
#207973=DIRECTION ( 'NONE',  ( 0.000000000000000000, 0.000000000000000000, -1.000000000000000000 ) ) ;
#207989=DIRECTION ( 'NONE',  ( 0.000000000000000000, 0.000000000000000000, -1.000000000000000000 ) ) ;
#208055=AXIS2_PLACEMENT_3D ( 'NONE', #202118, #41783, #120040 ) ;
#208075=CARTESIAN_POINT ( 'NONE',  ( 23.14999999999999503, 11.65000000000000746, -12.15000000000000036 ) ) ;
#208079=CARTESIAN_POINT ( 'NONE',  ( -21.65000000000000213, 7.708578643762696636, -12.34999999999999964 ) ) ;
#208105=CARTESIAN_POINT ( 'NONE',  ( 20.94999999999999929, 10.29288807858821286, -38.95800201601217339 ) ) ;
#208134=EDGE_CURVE ( 'NONE', #183417, #168131, #86297, .T. ) ;
#208148=CARTESIAN_POINT ( 'NONE',  ( 21.05000000000000071, -0.08561306080396914597, 6.413759733810287855 ) ) ;
#208159=DIRECTION ( 'NONE',  ( 1.000000000000000000, 0.000000000000000000, 0.000000000000000000 ) ) ;
#208200=CARTESIAN_POINT ( 'NONE',  ( -20.64999999999999858, -9.000000000000001776, -23.60603087734756045 ) ) ;
#208224=DIRECTION ( 'NONE',  ( 1.000000000000000000, -0.000000000000000000, -0.000000000000000000 ) ) ;
#208244=ORIENTED_EDGE ( 'NONE', *, *, #113552, .F. ) ;
#208263=CARTESIAN_POINT ( 'NONE',  ( -20.85000000000000142, -1.149570369575693807, -41.31591248450196474 ) ) ;
#208296=EDGE_CURVE ( 'NONE', #19688, #62457, #67736, .T. ) ;
#208302=CIRCLE ( 'NONE', #216473, 0.1999999999999987899 ) ;
#208307=ORIENTED_EDGE ( 'NONE', *, *, #230905, .T. ) ;
#208329=DIRECTION ( 'NONE',  ( 1.000000000000000000, 0.000000000000000000, 0.000000000000000000 ) ) ;
#208343=AXIS2_PLACEMENT_3D ( 'NONE', #231028, #71940, #150198 ) ;
#208368=ORIENTED_EDGE ( 'NONE', *, *, #239855, .T. ) ;
#208372=CIRCLE ( 'NONE', #8442, 0.09999999999999939493 ) ;
#208381=CARTESIAN_POINT ( 'NONE',  ( 21.07964655665547582, 8.774889614978558683, -12.22191658296405592 ) ) ;
#208383=ORIENTED_EDGE ( 'NONE', *, *, #200877, .T. ) ;
#208385=VERTEX_POINT ( 'NONE', #149738 ) ;
#208388=ORIENTED_EDGE ( 'NONE', *, *, #131123, .F. ) ;
#208410=DIRECTION ( 'NONE',  ( 0.000000000000000000, -1.000000000000000000, 0.000000000000000000 ) ) ;
#208425=CARTESIAN_POINT ( 'NONE',  ( 21.05000000000000071, 10.72371710470752149, -12.15000000000000036 ) ) ;
#208429=CARTESIAN_POINT ( 'NONE',  ( -21.05000000000000071, -11.48912529307605546, -30.39999999999999503 ) ) ;
#208479=AXIS2_PLACEMENT_3D ( 'NONE', #161360, #122223, #84310 ) ;
#208498=TOROIDAL_SURFACE ( 'NONE', #359, 7.800000000000000711, 0.1000000000000000056 ) ;
#208507=CIRCLE ( 'NONE', #16971, 0.09999999999999939493 ) ;
#208509=DIRECTION ( 'NONE',  ( 0.000000000000000000, 2.891205793294679805E-16, -1.000000000000000000 ) ) ;
#208526=CARTESIAN_POINT ( 'NONE',  ( 20.85000000000000142, -1.362429037193307435, -41.38888124792119783 ) ) ;
#208537=DIRECTION ( 'NONE',  ( 0.000000000000000000, -0.000000000000000000, 1.000000000000000000 ) ) ;
#208575=AXIS2_PLACEMENT_3D ( 'NONE', #214954, #114579, #118438 ) ;
#208578=DIRECTION ( 'NONE',  ( 0.000000000000000000, 1.000000000000000000, 0.000000000000000000 ) ) ;
#208579=DIRECTION ( 'NONE',  ( 1.000000000000000000, 0.000000000000000000, 0.000000000000000000 ) ) ;
#208588=AXIS2_PLACEMENT_3D ( 'NONE', #152066, #252404, #93344 ) ;
#208602=AXIS2_PLACEMENT_3D ( 'NONE', #157800, #237294, #58629 ) ;
#208613=ORIENTED_EDGE ( 'NONE', *, *, #15510, .F. ) ;
#208617=ORIENTED_EDGE ( 'NONE', *, *, #245643, .F. ) ;
#208625=CIRCLE ( 'NONE', #166952, 11.65000000000000036 ) ;
#208650=CARTESIAN_POINT ( 'NONE',  ( 21.05000000000000071, 2.449293598294710852E-16, -31.50000000000000000 ) ) ;
#208652=ORIENTED_EDGE ( 'NONE', *, *, #6457, .T. ) ;
#208672=DIRECTION ( 'NONE',  ( -1.000000000000000000, 0.000000000000000000, 0.000000000000000000 ) ) ;
#208674=DIRECTION ( 'NONE',  ( 1.000000000000000000, -0.000000000000000000, -0.000000000000000000 ) ) ;
#208724=ORIENTED_EDGE ( 'NONE', *, *, #117240, .T. ) ;
#208793=DIRECTION ( 'NONE',  ( 0.000000000000000000, 0.000000000000000000, -1.000000000000000000 ) ) ;
#208806=DIRECTION ( 'NONE',  ( 0.000000000000000000, 0.000000000000000000, -1.000000000000000000 ) ) ;
#208810=TOROIDAL_SURFACE ( 'NONE', #100438, 0.4000000000000015210, 0.1000000000000000056 ) ;
#208817=ORIENTED_EDGE ( 'NONE', *, *, #184356, .F. ) ;
#208882=VERTEX_POINT ( 'NONE', #161513 ) ;
#208897=EDGE_CURVE ( 'NONE', #185478, #161501, #160239, .T. ) ;
#208901=DIRECTION ( 'NONE',  ( -1.000000000000000000, 0.000000000000000000, 0.000000000000000000 ) ) ;
#208981=DIRECTION ( 'NONE',  ( 0.000000000000000000, 0.9654727137038715545, 0.2605042016806676242 ) ) ;
#208984=DIRECTION ( 'NONE',  ( 0.000000000000000000, 1.000000000000000000, 0.000000000000000000 ) ) ;
#208988=EDGE_LOOP ( 'NONE', ( #151178, #143995, #99688, #68908 ) ) ;
#209025=DIRECTION ( 'NONE',  ( -1.000000000000000000, 0.000000000000000000, 0.000000000000000000 ) ) ;
#209031=CARTESIAN_POINT ( 'NONE',  ( 20.85000000106584750, 11.75000000000000355, -26.65550465647362088 ) ) ;
#209046=DIRECTION ( 'NONE',  ( 0.000000000000000000, -1.000000000000000000, -1.734723475976807292E-15 ) ) ;
#209107=CARTESIAN_POINT ( 'NONE',  ( 23.24999999999999289, 11.65000000000000746, -12.15000000000000036 ) ) ;
#209124=ORIENTED_EDGE ( 'NONE', *, *, #43999, .T. ) ;
#209135=VERTEX_POINT ( 'NONE', #213447 ) ;
#209157=CARTESIAN_POINT ( 'NONE',  ( 20.94999999999999929, -11.64999999999999147, -33.50000000000000000 ) ) ;
#209163=AXIS2_PLACEMENT_3D ( 'NONE', #102488, #43842, #123378 ) ;
#209176=DIRECTION ( 'NONE',  ( 0.000000000000000000, 0.000000000000000000, -1.000000000000000000 ) ) ;
#209205=DIRECTION ( 'NONE',  ( 0.000000000000000000, 0.000000000000000000, -1.000000000000000000 ) ) ;
#209210=CARTESIAN_POINT ( 'NONE',  ( -20.54999999999999716, -11.75000000000000000, -21.15000000000000213 ) ) ;
#209229=PRESENTATION_STYLE_ASSIGNMENT (( #90558 ) ) ;
#209260=( BOUNDED_CURVE ( )  B_SPLINE_CURVE ( 3, ( #168437, #31470, #186675, #133111 ),
 .UNSPECIFIED., .F., .F. ) 
 B_SPLINE_CURVE_WITH_KNOTS ( ( 4, 4 ),
 ( 0.000000000000000000, 1.570796326794916320 ),
 .UNSPECIFIED. ) 
 CURVE ( )  GEOMETRIC_REPRESENTATION_ITEM ( )  RATIONAL_B_SPLINE_CURVE ( ( 1.000000000000000000, 0.8047378541243603856, 0.8047378541243603856, 1.000000000000000000 ) ) 
 REPRESENTATION_ITEM ( '' )  );
#209280=DIRECTION ( 'NONE',  ( 1.000000000000000000, 0.000000000000000000, 0.000000000000000000 ) ) ;
#209384=VECTOR ( 'NONE', #101313, 1000.000000000000000 ) ;
#209394=CARTESIAN_POINT ( 'NONE',  ( 22.32929514600007792, 7.578647565376482653, 0.09907567811391973511 ) ) ;
#209396=DIRECTION ( 'NONE',  ( 0.000000000000000000, 0.000000000000000000, -1.000000000000000000 ) ) ;
#209404=CARTESIAN_POINT ( 'NONE',  ( 21.04999999999951399, 10.50253167712597779, -7.558829817074861346 ) ) ;
#209422=ADVANCED_FACE ( 'NONE', ( #226258 ), #72046, .F. ) ;
#209448=CARTESIAN_POINT ( 'NONE',  ( -20.85000000000000142, 6.846123162352588665, -37.23772626684986164 ) ) ;
#209480=DIRECTION ( 'NONE',  ( 0.000000000000000000, 0.000000000000000000, -1.000000000000000000 ) ) ;
#209488=CARTESIAN_POINT ( 'NONE',  ( 23.14999999999999858, 2.100000000000002309, -33.50000000000000000 ) ) ;
#209495=AXIS2_PLACEMENT_3D ( 'NONE', #57891, #219538, #123032 ) ;
#209497=ORIENTED_EDGE ( 'NONE', *, *, #133171, .T. ) ;
#209533=DIRECTION ( 'NONE',  ( 1.000000000000000000, 0.000000000000000000, -3.469446951953635015E-14 ) ) ;
#209566=LINE ( 'NONE', #133871, #219499 ) ;
#209595=DIRECTION ( 'NONE',  ( -1.000000000000000000, 0.000000000000000000, 0.000000000000000000 ) ) ;
#209605=FACE_OUTER_BOUND ( 'NONE', #121425, .T. ) ;
#209608=DIRECTION ( 'NONE',  ( 1.000000000000000000, -0.000000000000000000, -0.000000000000000000 ) ) ;
#209618=ORIENTED_EDGE ( 'NONE', *, *, #62086, .F. ) ;
#209619=CARTESIAN_POINT ( 'NONE',  ( 21.05000000000000071, 8.815201804566768828, -8.420537496683621725 ) ) ;
#209672=DIRECTION ( 'NONE',  ( 1.000000000000000000, 0.000000000000000000, 0.000000000000000000 ) ) ;
#209690=DIRECTION ( 'NONE',  ( 1.000000000000000000, -0.000000000000000000, -0.000000000000000000 ) ) ;
#209718=CIRCLE ( 'NONE', #43123, 2.000000000000001776 ) ;
#209726=FACE_OUTER_BOUND ( 'NONE', #159051, .T. ) ;
#209752=EDGE_LOOP ( 'NONE', ( #108057, #146466, #5575, #59895 ) ) ;
#209763=VERTEX_POINT ( 'NONE', #101842 ) ;
#209855=CIRCLE ( 'NONE', #180812, 0.09999999999999892308 ) ;
#209874=CARTESIAN_POINT ( 'NONE',  ( -21.17356465864818205, 6.422803126241717564, 0.09891124101387023526 ) ) ;
#209903=VERTEX_POINT ( 'NONE', #136832 ) ;
#209923=DIRECTION ( 'NONE',  ( 0.000000000000000000, 0.000000000000000000, -1.000000000000000000 ) ) ;
#209938=FACE_OUTER_BOUND ( 'NONE', #36138, .T. ) ;
#209944=EDGE_CURVE ( 'NONE', #183282, #13885, #112168, .T. ) ;
#209950=DIRECTION ( 'NONE',  ( -1.000000000000000000, 0.000000000000000000, 0.000000000000000000 ) ) ;
#209961=CIRCLE ( 'NONE', #155796, 0.5000000000000004441 ) ;
#209989=CARTESIAN_POINT ( 'NONE',  ( 18.59999999999999076, 1.250000000000011546, -8.000000000000000000 ) ) ;
#209994=CARTESIAN_POINT ( 'NONE',  ( -18.39999999999999858, -9.500000000000005329, -7.032069396699667685 ) ) ;
#210036=FACE_OUTER_BOUND ( 'NONE', #122537, .T. ) ;
#210111=ORIENTED_EDGE ( 'NONE', *, *, #163657, .T. ) ;
#210130=EDGE_CURVE ( 'NONE', #157985, #105911, #42120, .T. ) ;
#210132=EDGE_CURVE ( 'NONE', #233325, #24291, #39517, .T. ) ;
#210134=LINE ( 'NONE', #172327, #223663 ) ;
#210143=CARTESIAN_POINT ( 'NONE',  ( -21.07946286933445279, 6.329037319007698947, 0.07668384325640564825 ) ) ;
#210144=DIRECTION ( 'NONE',  ( 1.000000000000000000, 0.000000000000000000, 0.000000000000000000 ) ) ;
#210153=ORIENTED_EDGE ( 'NONE', *, *, #131242, .F. ) ;
#210177=VERTEX_POINT ( 'NONE', #165400 ) ;
#210188=CARTESIAN_POINT ( 'NONE',  ( 18.49999999999999645, 1.637172712970381694, -11.58215336547201879 ) ) ;
#210198=AXIS2_PLACEMENT_3D ( 'NONE', #101723, #19665, #180025 ) ;
#210208=ORIENTED_EDGE ( 'NONE', *, *, #221025, .F. ) ;
#210213=FACE_OUTER_BOUND ( 'NONE', #39585, .T. ) ;
#210221=AXIS2_PLACEMENT_3D ( 'NONE', #27697, #49782, #47195 ) ;
#210228=ORIENTED_EDGE ( 'NONE', *, *, #106334, .F. ) ;
#210246=VERTEX_POINT ( 'NONE', #167995 ) ;
#210272=ORIENTED_EDGE ( 'NONE', *, *, #65909, .F. ) ;
#210292=LINE ( 'NONE', #107316, #161766 ) ;
#210299=CYLINDRICAL_SURFACE ( 'NONE', #113256, 4.049999999999998934 ) ;
#210374=CARTESIAN_POINT ( 'NONE',  ( 21.05000000000000071, -9.000000000000001776, -9.893969122652443104 ) ) ;
#210376=FACE_OUTER_BOUND ( 'NONE', #93444, .T. ) ;
#210380=DIRECTION ( 'NONE',  ( 1.000000000000000000, -0.000000000000000000, -0.000000000000000000 ) ) ;
#210381=CIRCLE ( 'NONE', #97899, 0.1999999999999987899 ) ;
#210444=ORIENTED_EDGE ( 'NONE', *, *, #127687, .T. ) ;
#210458=CIRCLE ( 'NONE', #23031, 0.1000000000000012407 ) ;
#210491=CARTESIAN_POINT ( 'NONE',  ( -20.00857864376270001, 9.250000000000001776, -21.25000000000000000 ) ) ;
#210494=ORIENTED_EDGE ( 'NONE', *, *, #156896, .T. ) ;
#210500=EDGE_LOOP ( 'NONE', ( #44940, #34017, #81422 ) ) ;
#210509=EDGE_CURVE ( 'NONE', #51098, #145748, #181147, .T. ) ;
#210510=CARTESIAN_POINT ( 'NONE',  ( -20.00857864376270001, 9.350000000000001421, -21.25000000000000000 ) ) ;
#210516=DIRECTION ( 'NONE',  ( 0.000000000000000000, -1.000000000000000000, 0.000000000000000000 ) ) ;
#210517=DIRECTION ( 'NONE',  ( 0.000000000000000000, 0.000000000000000000, 1.000000000000000000 ) ) ;
#210520=CARTESIAN_POINT ( 'NONE',  ( -22.50000000000000000, 0.000000000000000000, 11.64957080754479968 ) ) ;
#210525=( NAMED_UNIT ( * ) PLANE_ANGLE_UNIT ( ) SI_UNIT ( $, .RADIAN. ) );
#210533=DIRECTION ( 'NONE',  ( 0.000000000000000000, 0.000000000000000000, 1.000000000000000000 ) ) ;
#210575=DIRECTION ( 'NONE',  ( 0.000000000000000000, 0.000000000000000000, -1.000000000000000000 ) ) ;
#210611=EDGE_CURVE ( 'NONE', #226150, #45344, #152108, .T. ) ;
#210630=LINE ( 'NONE', #12452, #9470 ) ;
#210634=EDGE_CURVE ( 'NONE', #26951, #156138, #193600, .T. ) ;
#210650=CARTESIAN_POINT ( 'NONE',  ( 21.05000000000000071, 0.000000000000000000, -33.50000000000000000 ) ) ;
#210659=CARTESIAN_POINT ( 'NONE',  ( 21.13461538461538680, 8.885417037974457699, -12.34999999999999964 ) ) ;
#210660=DIRECTION ( 'NONE',  ( 0.000000000000000000, 0.000000000000000000, -1.000000000000000000 ) ) ;
#210667=CIRCLE ( 'NONE', #239713, 2.000000000000001776 ) ;
#210671=VERTEX_POINT ( 'NONE', #150654 ) ;
#210699=VERTEX_POINT ( 'NONE', #55358 ) ;
#210709=VECTOR ( 'NONE', #174470, 1000.000000000000000 ) ;
#210716=VERTEX_POINT ( 'NONE', #37143 ) ;
#210737=DIRECTION ( 'NONE',  ( -0.000000000000000000, -2.891205793294679805E-16, 1.000000000000000000 ) ) ;
#210767=FACE_OUTER_BOUND ( 'NONE', #211895, .T. ) ;
#210774=EDGE_LOOP ( 'NONE', ( #96010, #175734, #465, #151735, #187838, #99380, #8296, #16915 ) ) ;
#210796=FACE_OUTER_BOUND ( 'NONE', #112494, .T. ) ;
#210865=VERTEX_POINT ( 'NONE', #245600 ) ;
#210868=ORIENTED_EDGE ( 'NONE', *, *, #195307, .F. ) ;
#210905=VERTEX_POINT ( 'NONE', #44826 ) ;
#210912=EDGE_LOOP ( 'NONE', ( #183935, #50779, #42445 ) ) ;
#210949=DIRECTION ( 'NONE',  ( -1.000000000000000000, -2.952720810173289112E-16, 0.000000000000000000 ) ) ;
#210953=CARTESIAN_POINT ( 'NONE',  ( -21.05000000000000426, 11.60000000000000320, -6.928203230275554958 ) ) ;
#210967=CARTESIAN_POINT ( 'NONE',  ( 20.85000000000000142, -11.74999999999999112, -30.59999999999999432 ) ) ;
#210988=ORIENTED_EDGE ( 'NONE', *, *, #251912, .F. ) ;
#211027=FACE_OUTER_BOUND ( 'NONE', #103827, .T. ) ;
#211039=DIRECTION ( 'NONE',  ( -0.000000000000000000, -1.000000000000000000, -1.734723475976807292E-15 ) ) ;
#211044=ADVANCED_FACE ( 'NONE', ( #102859 ), #102161, .T. ) ;
#211047=CIRCLE ( 'NONE', #160986, 0.09999999999999939493 ) ;
#211056=DIRECTION ( 'NONE',  ( -0.000000000000000000, -0.000000000000000000, 1.000000000000000000 ) ) ;
#211069=CARTESIAN_POINT ( 'NONE',  ( 20.02499999999999858, 9.749999999999998224, -21.15000000000000213 ) ) ;
#211079=ORIENTED_EDGE ( 'NONE', *, *, #204308, .F. ) ;
#211087=CARTESIAN_POINT ( 'NONE',  ( 18.31325810956328937, -9.536388476007093828, -40.36844020630490348 ) ) ;
#211091=CARTESIAN_POINT ( 'NONE',  ( 20.85000000000000142, 0.000000000000000000, -33.50000000000000000 ) ) ;
#211093=ORIENTED_EDGE ( 'NONE', *, *, #184921, .F. ) ;
#211100=ADVANCED_FACE ( 'NONE', ( #164155 ), #38116, .T. ) ;
#211113=FACE_OUTER_BOUND ( 'NONE', #166253, .T. ) ;
#211164=ORIENTED_EDGE ( 'NONE', *, *, #137930, .F. ) ;
#211194=ORIENTED_EDGE ( 'NONE', *, *, #214189, .F. ) ;
#211216=EDGE_CURVE ( 'NONE', #239961, #235074, #225383, .T. ) ;
#211225=AXIS2_PLACEMENT_3D ( 'NONE', #45160, #242069, #162565 ) ;
#211233=EDGE_CURVE ( 'NONE', #6556, #241989, #88427, .T. ) ;
#211244=CARTESIAN_POINT ( 'NONE',  ( -21.05000000000000071, -0.1000000000000007688, 6.540656951701240729 ) ) ;
#211276=AXIS2_PLACEMENT_3D ( 'NONE', #183320, #125895, #63352 ) ;
#211296=EDGE_LOOP ( 'NONE', ( #45018, #69094, #161053 ) ) ;
#211301=CARTESIAN_POINT ( 'NONE',  ( -21.05000000000000071, 11.62071067811865177, -6.868416652341032602 ) ) ;
#211349=AXIS2_PLACEMENT_3D ( 'NONE', #254211, #198105, #116021 ) ;
#211358=SPHERICAL_SURFACE ( 'NONE', #85346, 0.1000000000000000056 ) ;
#211364=EDGE_CURVE ( 'NONE', #131148, #153971, #212278, .T. ) ;
#211366=ADVANCED_FACE ( 'NONE', ( #93595 ), #173170, .F. ) ;
#211389=CARTESIAN_POINT ( 'NONE',  ( -20.94999999999999929, 11.64999999999999680, -26.71613433702190576 ) ) ;
#211415=CIRCLE ( 'NONE', #48900, 0.1999999999999987899 ) ;
#211439=DIRECTION ( 'NONE',  ( -1.000000000000000000, -0.000000000000000000, -0.000000000000000000 ) ) ;
#211448=AXIS2_PLACEMENT_3D ( 'NONE', #79994, #201247, #43472 ) ;
#211457=EDGE_CURVE ( 'NONE', #226150, #31765, #177431, .T. ) ;
#211530=AXIS2_PLACEMENT_3D ( 'NONE', #152937, #69532, #232462 ) ;
#211535=AXIS2_PLACEMENT_3D ( 'NONE', #187471, #167922, #68799 ) ;
#211570=DIRECTION ( 'NONE',  ( 0.000000000000000000, 0.000000000000000000, 1.000000000000000000 ) ) ;
#211573=DIRECTION ( 'NONE',  ( 1.000000000000000000, 0.000000000000000000, 0.000000000000000000 ) ) ;
#211613=VERTEX_POINT ( 'NONE', #6029 ) ;
#211631=ADVANCED_FACE ( 'NONE', ( #110270 ), #145544, .T. ) ;
#211635=DIRECTION ( 'NONE',  ( -0.000000000000000000, 0.000000000000000000, 1.000000000000000000 ) ) ;
#211692=EDGE_LOOP ( 'NONE', ( #198399, #53678, #215872 ) ) ;
#211711=ORIENTED_EDGE ( 'NONE', *, *, #32116, .T. ) ;
#211759=CARTESIAN_POINT ( 'NONE',  ( -21.05000000000000071, 1.249999999999999334, -8.000000000000000000 ) ) ;
#211773=AXIS2_PLACEMENT_3D ( 'NONE', #170881, #232100, #32640 ) ;
#211780=VERTEX_POINT ( 'NONE', #192390 ) ;
#211832=VECTOR ( 'NONE', #204881, 1000.000000000000000 ) ;
#211875=FACE_OUTER_BOUND ( 'NONE', #103351, .T. ) ;
#211881=DIRECTION ( 'NONE',  ( -1.000000000000000000, 0.000000000000000000, 0.000000000000000000 ) ) ;
#211894=CYLINDRICAL_SURFACE ( 'NONE', #213943, 0.09999999999999939493 ) ;
#211895=EDGE_LOOP ( 'NONE', ( #147552, #245939, #257380, #156100 ) ) ;
#211902=AXIS2_PLACEMENT_3D ( 'NONE', #234715, #75659, #194330 ) ;
#211916=DIRECTION ( 'NONE',  ( 1.000000000000000000, 7.304098846218134667E-16, 0.000000000000000000 ) ) ;
#211919=ORIENTED_EDGE ( 'NONE', *, *, #234035, .T. ) ;
#211933=CARTESIAN_POINT ( 'NONE',  ( 20.94999999999999929, 4.999999999999997335, -21.09473398108690390 ) ) ;
#211936=CARTESIAN_POINT ( 'NONE',  ( 18.59999999999999787, -1.835341550224411922, -11.65515129256297833 ) ) ;
#211946=VECTOR ( 'NONE', #7994, 1000.000000000000000 ) ;
#211954=EDGE_CURVE ( 'NONE', #78587, #71514, #40234, .T. ) ;
#211960=DIRECTION ( 'NONE',  ( 0.000000000000000000, 1.224646799147316229E-16, 1.000000000000000000 ) ) ;
#211986=EDGE_CURVE ( 'NONE', #79953, #184680, #40610, .T. ) ;
#211994=CARTESIAN_POINT ( 'NONE',  ( 21.05000000000000071, 10.56271494672853528, -7.456802105644634082 ) ) ;
#212007=ADVANCED_FACE ( 'NONE', ( #203501 ), #238776, .F. ) ;
#212034=DIRECTION ( 'NONE',  ( 0.000000000000000000, -1.000000000000000000, 0.000000000000000000 ) ) ;
#212059=PLANE ( 'NONE',  #219618 ) ;
#212062=DIRECTION ( 'NONE',  ( 0.000000000000000000, 0.000000000000000000, -1.000000000000000000 ) ) ;
#212108=CARTESIAN_POINT ( 'NONE',  ( -21.53551880898957904, 0.09896973457166240162, 6.784797761416331952 ) ) ;
#212123=VECTOR ( 'NONE', #182172, 1000.000000000000227 ) ;
#212127=AXIS2_PLACEMENT_3D ( 'NONE', #13769, #93300, #209396 ) ;
#212161=ORIENTED_EDGE ( 'NONE', *, *, #106129, .T. ) ;
#212173=LINE ( 'NONE', #173081, #55364 ) ;
#212194=ADVANCED_FACE ( 'NONE', ( #129099 ), #111120, .T. ) ;
#212201=VERTEX_POINT ( 'NONE', #208650 ) ;
#212221=EDGE_LOOP ( 'NONE', ( #4246, #233305, #241940, #241361 ) ) ;
#212230=CARTESIAN_POINT ( 'NONE',  ( 21.05995757104869526, 8.775389244721274906, -12.19490512299120866 ) ) ;
#212237=ORIENTED_EDGE ( 'NONE', *, *, #19359, .T. ) ;
#212260=AXIS2_PLACEMENT_3D ( 'NONE', #166478, #7367, #186009 ) ;
#212278=LINE ( 'NONE', #136550, #210709 ) ;
#212279=DIRECTION ( 'NONE',  ( 0.000000000000000000, -0.000000000000000000, -1.000000000000000000 ) ) ;
#212311=CARTESIAN_POINT ( 'NONE',  ( 21.05000000000000071, 4.999999999999997335, -21.09473398108690390 ) ) ;
#212327=CARTESIAN_POINT ( 'NONE',  ( -18.44232395689901693, -9.552282557050347123, -40.34225198480720564 ) ) ;
#212354=CARTESIAN_POINT ( 'NONE',  ( 22.39999999999999503, 7.790779598373379855, 0.000000000000000000 ) ) ;
#212414=EDGE_CURVE ( 'NONE', #216736, #138911, #165487, .T. ) ;
#212448=DIRECTION ( 'NONE',  ( 1.000000000000000000, 0.000000000000000000, -0.000000000000000000 ) ) ;
#212457=AXIS2_PLACEMENT_3D ( 'NONE', #112460, #188129, #227244 ) ;
#212465=CARTESIAN_POINT ( 'NONE',  ( -18.59999999999999787, 9.350000000000001421, -12.25000000000000000 ) ) ;
#212474=VERTEX_POINT ( 'NONE', #218751 ) ;
#212483=ADVANCED_FACE ( 'NONE', ( #2270 ), #122244, .T. ) ;
#212494=SPHERICAL_SURFACE ( 'NONE', #2868, 0.1000000000000000056 ) ;
#212526=FACE_OUTER_BOUND ( 'NONE', #98017, .T. ) ;
#212528=AXIS2_PLACEMENT_3D ( 'NONE', #76491, #77765, #56903 ) ;
#212556=DIRECTION ( 'NONE',  ( -1.000000000000000000, 3.469446951953635015E-14, 0.000000000000000000 ) ) ;
#212567=DIRECTION ( 'NONE',  ( 0.000000000000000000, 0.000000000000000000, -1.000000000000000000 ) ) ;
#212569=CIRCLE ( 'NONE', #141793, 0.09999999999999939493 ) ;
#212573=AXIS2_PLACEMENT_3D ( 'NONE', #205586, #26996, #106473 ) ;
#212576=AXIS2_PLACEMENT_3D ( 'NONE', #99333, #74708, #253286 ) ;
#212584=CIRCLE ( 'NONE', #100110, 0.1999999999999996503 ) ;
#212586=CARTESIAN_POINT ( 'NONE',  ( 18.53691006697099652, 10.30215155715038122, -24.70219871729854333 ) ) ;
#212604=CYLINDRICAL_SURFACE ( 'NONE', #229913, 0.09999999999999939493 ) ;
#212653=DIRECTION ( 'NONE',  ( -0.7071067811865474617, -0.7071067811865474617, -2.044391222244499837E-16 ) ) ;
#212658=CARTESIAN_POINT ( 'NONE',  ( -20.54999999999999716, -9.000000000000003553, -9.393969122652443104 ) ) ;
#212677=DIRECTION ( 'NONE',  ( 1.000000000000000000, 0.000000000000000000, -0.000000000000000000 ) ) ;
#212680=CARTESIAN_POINT ( 'NONE',  ( 21.14250536705908345, 6.518172176880724145, -1.950243336660753025E-16 ) ) ;
#212681=AXIS2_PLACEMENT_3D ( 'NONE', #64390, #143910, #223441 ) ;
#212689=CARTESIAN_POINT ( 'NONE',  ( -23.15000000000000213, 2.499999999999998668, -20.27537807723790309 ) ) ;
#212691=DIRECTION ( 'NONE',  ( 0.000000000000000000, 0.000000000000000000, -1.000000000000000000 ) ) ;
#212718=ADVANCED_FACE ( 'NONE', ( #231622 ), #212059, .F. ) ;
#212736=EDGE_CURVE ( 'NONE', #47066, #183282, #136322, .T. ) ;
#212740=DIRECTION ( 'NONE',  ( 3.265361837132813093E-16, -1.000000000000000000, -0.000000000000000000 ) ) ;
#212741=VECTOR ( 'NONE', #250517, 1000.000000000000000 ) ;
#212765=AXIS2_PLACEMENT_3D ( 'NONE', #128863, #208410, #170600 ) ;
#212771=ORIENTED_EDGE ( 'NONE', *, *, #119733, .T. ) ;
#212775=ORIENTED_EDGE ( 'NONE', *, *, #216250, .F. ) ;
#212779=ADVANCED_FACE ( 'NONE', ( #196320 ), #176788, .F. ) ;
#212784=ORIENTED_EDGE ( 'NONE', *, *, #147138, .T. ) ;
#212815=LINE ( 'NONE', #164395, #215395 ) ;
#212817=CYLINDRICAL_SURFACE ( 'NONE', #58051, 0.5000000000000022204 ) ;
#212883=DIRECTION ( 'NONE',  ( 0.000000000000000000, -1.000000000000000000, 0.000000000000000000 ) ) ;
#212898=AXIS2_PLACEMENT_3D ( 'NONE', #47828, #64836, #144351 ) ;
#212920=DIRECTION ( 'NONE',  ( 0.000000000000000000, 0.000000000000000000, -1.000000000000000000 ) ) ;
#212943=AXIS2_PLACEMENT_3D ( 'NONE', #58037, #217110, #77596 ) ;
#212983=EDGE_LOOP ( 'NONE', ( #41866, #234193, #35545, #37029 ) ) ;
#213001=DIRECTION ( 'NONE',  ( 1.836970198721029934E-16, -1.000000000000000000, -0.000000000000000000 ) ) ;
#213024=CIRCLE ( 'NONE', #92216, 0.1000000000000028644 ) ;
#213042=EDGE_CURVE ( 'NONE', #219381, #45344, #140711, .T. ) ;
#213047=ORIENTED_EDGE ( 'NONE', *, *, #201474, .T. ) ;
#213048=ORIENTED_EDGE ( 'NONE', *, *, #26392, .F. ) ;
#213069=CIRCLE ( 'NONE', #58922, 0.1000000000000001860 ) ;
#213102=CARTESIAN_POINT ( 'NONE',  ( 22.47071067811865319, 0.000000000000000000, 0.000000000000000000 ) ) ;
#213107=DIRECTION ( 'NONE',  ( -1.000000000000000000, -0.000000000000000000, -0.000000000000000000 ) ) ;
#213112=VERTEX_POINT ( 'NONE', #119067 ) ;
#213130=ADVANCED_FACE ( 'NONE', ( #378 ), #141191, .T. ) ;
#213156=EDGE_CURVE ( 'NONE', #223333, #213112, #203253, .T. ) ;
#213187=ORIENTED_EDGE ( 'NONE', *, *, #77516, .F. ) ;
#213192=DIRECTION ( 'NONE',  ( 0.000000000000000000, 0.000000000000000000, 1.000000000000000000 ) ) ;
#213208=DIRECTION ( 'NONE',  ( 0.000000000000000000, 0.1575844902526452040, 0.9875055080513798211 ) ) ;
#213234=DIRECTION ( 'NONE',  ( 0.000000000000000000, -0.8660254037844459241, -0.4999999999999873990 ) ) ;
#213238=ADVANCED_FACE ( 'NONE', ( #223277 ), #68071, .T. ) ;
#213249=CARTESIAN_POINT ( 'NONE',  ( 21.05000000000000071, 10.54375127549566926, -7.556387808664851491 ) ) ;
#213251=EDGE_LOOP ( 'NONE', ( #41612, #211919, #49600, #74176, #195388, #70142, #157943, #232421, #48268, #58202, #120156, #238409, #203148, #102062, #108354, #82257 ) ) ;
#213258=CARTESIAN_POINT ( 'NONE',  ( -23.15000000000000213, 2.600000000000000089, 11.75000000000000000 ) ) ;
#213315=VERTEX_POINT ( 'NONE', #148907 ) ;
#213317=DIRECTION ( 'NONE',  ( 1.000000000000000000, 0.000000000000000000, 0.000000000000000000 ) ) ;
#213327=ORIENTED_EDGE ( 'NONE', *, *, #202739, .T. ) ;
#213346=CARTESIAN_POINT ( 'NONE',  ( 21.00023020733503643, -5.827586677109586333E-16, 6.390869245268367749 ) ) ;
#213367=DIRECTION ( 'NONE',  ( 0.000000000000000000, 0.000000000000000000, 1.000000000000000000 ) ) ;
#213403=LINE ( 'NONE', #72647, #154957 ) ;
#213430=CARTESIAN_POINT ( 'NONE',  ( 20.93284271247462414, 11.75000000000000355, -26.48519422934606382 ) ) ;
#213447=CARTESIAN_POINT ( 'NONE',  ( -20.64999999999999858, 4.349999999999999645, -21.25000000000000000 ) ) ;
#213455=CARTESIAN_POINT ( 'NONE',  ( -20.54999999999999716, -9.000000000000001776, -23.60603087734756045 ) ) ;
#213462=CARTESIAN_POINT ( 'NONE',  ( 20.95512820512820440, 8.876151316288117599, -8.558628995140949769 ) ) ;
#213470=DIRECTION ( 'NONE',  ( 0.000000000000000000, 0.4930308989875230585, 0.8700118002898322711 ) ) ;
#213474=CIRCLE ( 'NONE', #238423, 0.1000000000000028644 ) ;
#213510=CARTESIAN_POINT ( 'NONE',  ( -21.59142135623730852, 7.850000000000003197, -21.25000000000000000 ) ) ;
#213517=CARTESIAN_POINT ( 'NONE',  ( 21.13461538461538680, 10.61458296202553875, -12.35000000000000142 ) ) ;
#213529=DIRECTION ( 'NONE',  ( 1.000000000000000000, 0.000000000000000000, 0.000000000000000000 ) ) ;
#213536=EDGE_LOOP ( 'NONE', ( #4330, #31506, #207059, #152193 ) ) ;
#213540=CARTESIAN_POINT ( 'NONE',  ( 18.58719872626880942, -9.566644397598638605, -40.32247819639701447 ) ) ;
#213550=EDGE_LOOP ( 'NONE', ( #199768, #112271, #122551 ) ) ;
#213579=CARTESIAN_POINT ( 'NONE',  ( -18.50000000000000000, -9.480686695278974341, -40.44111516875785384 ) ) ;
#213598=VERTEX_POINT ( 'NONE', #63920 ) ;
#213647=FACE_OUTER_BOUND ( 'NONE', #55501, .T. ) ;
#213652=AXIS2_PLACEMENT_3D ( 'NONE', #87788, #249469, #70849 ) ;
#213754=DIRECTION ( 'NONE',  ( 0.000000000000000000, 0.000000000000000000, 1.000000000000000000 ) ) ;
#213783=CARTESIAN_POINT ( 'NONE',  ( -20.54999999999999716, -8.663551401869161950, -9.524101118067305194 ) ) ;
#213809=CARTESIAN_POINT ( 'NONE',  ( 22.39999999999999503, 0.000000000000000000, 7.750000000000007105 ) ) ;
#213828=LINE ( 'NONE', #168333, #199934 ) ;
#213858=DIRECTION ( 'NONE',  ( 0.000000000000000000, 0.000000000000000000, -1.000000000000000000 ) ) ;
#213916=ORIENTED_EDGE ( 'NONE', *, *, #219331, .F. ) ;
#213920=ADVANCED_FACE ( 'NONE', ( #183232 ), #2001, .F. ) ;
#213936=ORIENTED_EDGE ( 'NONE', *, *, #95023, .F. ) ;
#213940=ADVANCED_FACE ( 'NONE', ( #241902 ), #25447, .F. ) ;
#213942=CARTESIAN_POINT ( 'NONE',  ( -23.25000000000000000, 11.75000000000000000, -21.34999999999999787 ) ) ;
#213943=AXIS2_PLACEMENT_3D ( 'NONE', #133615, #33278, #112779 ) ;
#213948=EDGE_CURVE ( 'NONE', #119315, #18766, #144762, .T. ) ;
#213953=AXIS2_PLACEMENT_3D ( 'NONE', #71519, #11534, #51902 ) ;
#213973=EDGE_CURVE ( 'NONE', #140135, #178016, #17377, .T. ) ;
#213975=CARTESIAN_POINT ( 'NONE',  ( -20.94999999999999929, 1.749999999999999778, -11.66951155790164307 ) ) ;
#213985=ORIENTED_EDGE ( 'NONE', *, *, #239888, .T. ) ;
#214000=VERTEX_POINT ( 'NONE', #147954 ) ;
#214033=VERTEX_POINT ( 'NONE', #150528 ) ;
#214079=VERTEX_POINT ( 'NONE', #188362 ) ;
#214101=CIRCLE ( 'NONE', #81167, 0.09999999999999939493 ) ;
#214105=ORIENTED_EDGE ( 'NONE', *, *, #240695, .T. ) ;
#214118=VECTOR ( 'NONE', #254328, 1000.000000000000000 ) ;
#214167=VERTEX_POINT ( 'NONE', #18711 ) ;
#214171=DIRECTION ( 'NONE',  ( -0.7071067811865388020, 0.7071067811865561215, 0.000000000000000000 ) ) ;
#214189=EDGE_CURVE ( 'NONE', #251285, #213112, #254705, .T. ) ;
#214200=CARTESIAN_POINT ( 'NONE',  ( -22.39999999999999858, 7.790779598373403836, 0.09999999999999939493 ) ) ;
#214235=EDGE_CURVE ( 'NONE', #223036, #139879, #193514, .T. ) ;
#214304=DIRECTION ( 'NONE',  ( 1.000000000000000000, -0.000000000000000000, -0.000000000000000000 ) ) ;
#214311=CARTESIAN_POINT ( 'NONE',  ( 21.05000000000000071, 5.499999999999998224, -21.09473398108690390 ) ) ;
#214317=CYLINDRICAL_SURFACE ( 'NONE', #140927, 0.5000000000000004441 ) ;
#214377=TOROIDAL_SURFACE ( 'NONE', #206011, 0.2000000000000000111, 0.1000000000000000056 ) ;
#214382=CARTESIAN_POINT ( 'NONE',  ( -20.64999999999999858, 0.000000000000000000, 0.000000000000000000 ) ) ;
#214391=EDGE_CURVE ( 'NONE', #7751, #31598, #124145, .T. ) ;
#214393=CARTESIAN_POINT ( 'NONE',  ( 21.05000000000000071, -1.162701749938009677, -8.099999999999999645 ) ) ;
#214416=CARTESIAN_POINT ( 'NONE',  ( 21.10642757222115407, 10.72315628915859520, -12.24069752378520093 ) ) ;
#214422=CIRCLE ( 'NONE', #52108, 0.5000000000000004441 ) ;
#214429=CIRCLE ( 'NONE', #127137, 0.09999999999999939493 ) ;
#214454=ORIENTED_EDGE ( 'NONE', *, *, #26423, .T. ) ;
#214465=ORIENTED_EDGE ( 'NONE', *, *, #124135, .F. ) ;
#214472=VERTEX_POINT ( 'NONE', #86354 ) ;
#214498=DIRECTION ( 'NONE',  ( 0.000000000000000000, 8.673617379883787770E-15, -1.000000000000000000 ) ) ;
#214499=CARTESIAN_POINT ( 'NONE',  ( -20.85000000000000142, 0.000000000000000000, -33.50000000000000000 ) ) ;
#214526=EDGE_CURVE ( 'NONE', #26951, #55509, #169964, .T. ) ;
#214533=ADVANCED_FACE ( 'NONE', ( #66831 ), #168548, .F. ) ;
#214560=CARTESIAN_POINT ( 'NONE',  ( -21.14999999999999858, 11.65000000000000036, -0.1000000000000028644 ) ) ;
#214568=TOROIDAL_SURFACE ( 'NONE', #243625, 12.97499999999999609, 0.1000000000000000056 ) ;
#214575=DIRECTION ( 'NONE',  ( 0.000000000000000000, -0.8068669527896844551, -0.5907332058517525963 ) ) ;
#214585=ORIENTED_EDGE ( 'NONE', *, *, #82310, .T. ) ;
#214599=DIRECTION ( 'NONE',  ( 0.000000000000000000, -0.000000000000000000, -1.000000000000000000 ) ) ;
#214604=CARTESIAN_POINT ( 'NONE',  ( -23.15000000000000213, -11.48912529307605546, -30.39999999999999503 ) ) ;
#214632=CARTESIAN_POINT ( 'NONE',  ( 21.53752568622133978, 0.09897446126636881558, 6.786807874548579811 ) ) ;
#214664=EDGE_CURVE ( 'NONE', #154965, #193883, #16006, .T. ) ;
#214667=DIRECTION ( 'NONE',  ( 0.000000000000000000, 0.000000000000000000, -1.000000000000000000 ) ) ;
#214669=VERTEX_POINT ( 'NONE', #54939 ) ;
#214680=AXIS2_PLACEMENT_3D ( 'NONE', #253086, #190581, #150167 ) ;
#214699=EDGE_CURVE ( 'NONE', #214669, #116070, #163078, .T. ) ;
#214713=ORIENTED_EDGE ( 'NONE', *, *, #184122, .T. ) ;
#214729=EDGE_LOOP ( 'NONE', ( #196175, #93798, #96749, #123668 ) ) ;
#214735=LINE ( 'NONE', #217286, #7232 ) ;
#214739=DIRECTION ( 'NONE',  ( 0.000000000000000000, 1.000000000000000000, 0.000000000000000000 ) ) ;
#214749=CARTESIAN_POINT ( 'NONE',  ( 21.05000000000000071, -9.000000000000000000, -23.60603087734755690 ) ) ;
#214763=AXIS2_PLACEMENT_3D ( 'NONE', #119631, #59610, #199154 ) ;
#214773=ORIENTED_EDGE ( 'NONE', *, *, #41835, .F. ) ;
#214807=EDGE_CURVE ( 'NONE', #133804, #243786, #257516, .T. ) ;
#214840=CARTESIAN_POINT ( 'NONE',  ( 23.25000000000000000, -11.74999999999999112, 11.75000000000000000 ) ) ;
#214888=EDGE_CURVE ( 'NONE', #242879, #227113, #28499, .T. ) ;
#214914=CARTESIAN_POINT ( 'NONE',  ( 18.49999999999999645, 0.000000000000000000, 0.000000000000000000 ) ) ;
#214915=ADVANCED_FACE ( 'NONE', ( #33861 ), #36862, .T. ) ;
#214930=CARTESIAN_POINT ( 'NONE',  ( 18.47135592147654748, -9.471088613265669309, -40.18359493984359432 ) ) ;
#214954=CARTESIAN_POINT ( 'NONE',  ( 20.94999999999999929, 8.776282895292471409, -8.558628995140949769 ) ) ;
#214976=FACE_OUTER_BOUND ( 'NONE', #389, .T. ) ;
#215010=EDGE_CURVE ( 'NONE', #147515, #77132, #232034, .T. ) ;
#215020=AXIS2_PLACEMENT_3D ( 'NONE', #96979, #157022, #99564 ) ;
#215057=ORIENTED_EDGE ( 'NONE', *, *, #223629, .T. ) ;
#215071=CIRCLE ( 'NONE', #102603, 0.09999999999999939493 ) ;
#215076=ORIENTED_EDGE ( 'NONE', *, *, #209944, .F. ) ;
#215080=DIRECTION ( 'NONE',  ( 0.000000000000000000, 0.000000000000000000, 1.000000000000000000 ) ) ;
#215110=DIRECTION ( 'NONE',  ( 0.000000000000000000, 0.000000000000000000, -1.000000000000000000 ) ) ;
#215124=ADVANCED_FACE ( 'NONE', ( #220159 ), #18094, .T. ) ;
#215139=DIRECTION ( 'NONE',  ( 1.000000000000000000, 0.000000000000000000, 0.000000000000000000 ) ) ;
#215219=DIRECTION ( 'NONE',  ( 0.000000000000000000, 0.9654727137038715545, -0.2605042016806676242 ) ) ;
#215234=EDGE_LOOP ( 'NONE', ( #224286, #227311, #143092, #48071 ) ) ;
#215275=CARTESIAN_POINT ( 'NONE',  ( 20.95561247346651967, 10.59500736520355346, -7.593782766981634680 ) ) ;
#215286=LINE ( 'NONE', #78331, #164201 ) ;
#215299=ADVANCED_FACE ( 'NONE', ( #4918 ), #87030, .F. ) ;
#215329=CARTESIAN_POINT ( 'NONE',  ( 21.14999999999999858, 11.65000000000000391, -0.1000000000000028644 ) ) ;
#215358=DIRECTION ( 'NONE',  ( 1.000000000000000000, 0.000000000000000000, 0.000000000000000000 ) ) ;
#215363=DIRECTION ( 'NONE',  ( 0.000000000000000000, -1.000000000000000000, 0.000000000000000000 ) ) ;
#215374=EDGE_LOOP ( 'NONE', ( #60204, #206756, #92712, #190771 ) ) ;
#215395=VECTOR ( 'NONE', #243912, 1000.000000000000000 ) ;
#215399=AXIS2_PLACEMENT_3D ( 'NONE', #218951, #181136, #143270 ) ;
#215406=ORIENTED_EDGE ( 'NONE', *, *, #104171, .T. ) ;
#215450=VECTOR ( 'NONE', #189850, 1000.000000000000000 ) ;
#215465=CARTESIAN_POINT ( 'NONE',  ( -22.50000000000000000, 11.65000000000000036, -3.469446951953614189E-15 ) ) ;
#215498=CARTESIAN_POINT ( 'NONE',  ( -18.50000000000000000, -9.400000000000005684, -40.38204184817266906 ) ) ;
#215535=EDGE_CURVE ( 'NONE', #144794, #19688, #245961, .T. ) ;
#215572=ORIENTED_EDGE ( 'NONE', *, *, #176143, .T. ) ;
#215611=CIRCLE ( 'NONE', #211535, 0.1000000000000002554 ) ;
#215626=ORIENTED_EDGE ( 'NONE', *, *, #119588, .T. ) ;
#215628=EDGE_LOOP ( 'NONE', ( #85446, #98539, #14030, #241623 ) ) ;
#215652=CARTESIAN_POINT ( 'NONE',  ( -21.14999999999999503, 11.74999999999999467, -6.919147245958762404 ) ) ;
#215656=DIRECTION ( 'NONE',  ( 0.000000000000000000, 0.000000000000000000, -1.000000000000000000 ) ) ;
#215666=ORIENTED_EDGE ( 'NONE', *, *, #72815, .T. ) ;
#215744=CARTESIAN_POINT ( 'NONE',  ( -23.15000000000000213, 0.000000000000000000, -21.69999999999999929 ) ) ;
#215773=ORIENTED_EDGE ( 'NONE', *, *, #196185, .F. ) ;
#215817=CARTESIAN_POINT ( 'NONE',  ( 23.15000000000000213, -9.599999999999999645, -23.60603087734755690 ) ) ;
#215872=ORIENTED_EDGE ( 'NONE', *, *, #84414, .T. ) ;
#215875=CIRCLE ( 'NONE', #24389, 12.97499999999999787 ) ;
#215878=CIRCLE ( 'NONE', #157502, 0.2000000000000005107 ) ;
#215884=CARTESIAN_POINT ( 'NONE',  ( -20.00857864376270001, 9.150000000000002132, -21.25000000000000000 ) ) ;
#215905=DIRECTION ( 'NONE',  ( 0.000000000000000000, -1.000000000000000000, 0.000000000000000000 ) ) ;
#215944=AXIS2_PLACEMENT_3D ( 'NONE', #18266, #199492, #57369 ) ;
#215948=AXIS2_PLACEMENT_3D ( 'NONE', #205430, #188448, #9811 ) ;
#215959=AXIS2_PLACEMENT_3D ( 'NONE', #61189, #100290, #117315 ) ;
#216067=DIRECTION ( 'NONE',  ( 0.000000000000000000, 1.000000000000000000, 0.000000000000000000 ) ) ;
#216082=CARTESIAN_POINT ( 'NONE',  ( 21.09551895715246772, 10.62143732716875100, -12.23712466589941883 ) ) ;
#216096=CARTESIAN_POINT ( 'NONE',  ( -22.39999999999999858, -0.1008583690987135961, 11.74956712348939192 ) ) ;
#216146=CARTESIAN_POINT ( 'NONE',  ( -20.64999999999999858, 0.000000000000000000, -12.87499999999999822 ) ) ;
#216163=CARTESIAN_POINT ( 'NONE',  ( 21.05000000000000071, -1.124859753953710850E-15, 6.540656951701244282 ) ) ;
#216177=DIRECTION ( 'NONE',  ( -1.000000000000000000, 0.000000000000000000, 0.000000000000000000 ) ) ;
#216182=CARTESIAN_POINT ( 'NONE',  ( 18.50000000000000000, -9.399999999999979039, -7.297259759663266898 ) ) ;
#216186=EDGE_CURVE ( 'NONE', #211780, #68319, #36037, .T. ) ;
#216198=( BOUNDED_CURVE ( )  B_SPLINE_CURVE ( 3, ( #202302, #103178, #182754, #4094 ),
 .UNSPECIFIED., .F., .F. ) 
 B_SPLINE_CURVE_WITH_KNOTS ( ( 4, 4 ),
 ( 3.141592653589793116, 4.712388980384689674 ),
 .UNSPECIFIED. ) 
 CURVE ( )  GEOMETRIC_REPRESENTATION_ITEM ( )  RATIONAL_B_SPLINE_CURVE ( ( 1.000000000000000000, 0.8047378541243649375, 0.8047378541243649375, 1.000000000000000000 ) ) 
 REPRESENTATION_ITEM ( '' )  );
#216223=CARTESIAN_POINT ( 'NONE',  ( -21.59142135623730852, 7.850000000000003197, -21.15000000000000213 ) ) ;
#216250=EDGE_CURVE ( 'NONE', #182491, #248548, #22130, .T. ) ;
#216309=CYLINDRICAL_SURFACE ( 'NONE', #243408, 0.09999999999999976963 ) ;
#216320=VERTEX_POINT ( 'NONE', #163679 ) ;
#216329=ADVANCED_FACE ( 'NONE', ( #120719 ), #63276, .T. ) ;
#216352=EDGE_CURVE ( 'NONE', #103069, #73708, #21605, .T. ) ;
#216361=CARTESIAN_POINT ( 'NONE',  ( 20.11144452914042091, 9.933610851122994134, -7.890293453954491554 ) ) ;
#216366=DIRECTION ( 'NONE',  ( -1.000000000000000000, 0.000000000000000000, 0.000000000000000000 ) ) ;
#216384=CARTESIAN_POINT ( 'NONE',  ( 18.59999999999999787, -11.74999999999999289, -21.35000000000000142 ) ) ;
#216402=CARTESIAN_POINT ( 'NONE',  ( 23.24999999999999289, -4.149999999999999467, 0.000000000000000000 ) ) ;
#216424=DIRECTION ( 'NONE',  ( 0.000000000000000000, -1.000000000000000000, 0.000000000000000000 ) ) ;
#216431=CARTESIAN_POINT ( 'NONE',  ( 21.14999999999999858, 6.649999999999999467, -12.15000000000000036 ) ) ;
#216439=DIRECTION ( 'NONE',  ( 2.952720810173289112E-16, -1.000000000000000000, 0.000000000000000000 ) ) ;
#216444=CARTESIAN_POINT ( 'NONE',  ( -18.59999999999999787, 1.249999999999999334, -8.000000000000000000 ) ) ;
#216452=ORIENTED_EDGE ( 'NONE', *, *, #184376, .T. ) ;
#216473=AXIS2_PLACEMENT_3D ( 'NONE', #16376, #256178, #193716 ) ;
#216496=DIRECTION ( 'NONE',  ( 0.000000000000000000, 0.000000000000000000, -1.000000000000000000 ) ) ;
#216499=ORIENTED_EDGE ( 'NONE', *, *, #257293, .F. ) ;
#216539=CYLINDRICAL_SURFACE ( 'NONE', #237697, 0.8750000000000007772 ) ;
#216542=EDGE_CURVE ( 'NONE', #94181, #103069, #195784, .T. ) ;
#216568=CARTESIAN_POINT ( 'NONE',  ( -21.05000000000000071, 11.75000000000000000, -26.48519422934605316 ) ) ;
#216623=FACE_OUTER_BOUND ( 'NONE', #132619, .T. ) ;
#216641=ORIENTED_EDGE ( 'NONE', *, *, #191687, .T. ) ;
#216648=AXIS2_PLACEMENT_3D ( 'NONE', #116659, #157091, #41007 ) ;
#216657=CARTESIAN_POINT ( 'NONE',  ( 23.24999999999999645, 0.000000000000000000, -33.50000000000000000 ) ) ;
#216703=CARTESIAN_POINT ( 'NONE',  ( -20.54999999999999716, 0.000000000000000000, -33.50000000000000000 ) ) ;
#216733=FACE_OUTER_BOUND ( 'NONE', #43135, .T. ) ;
#216736=VERTEX_POINT ( 'NONE', #46926 ) ;
#216761=AXIS2_PLACEMENT_3D ( 'NONE', #134935, #91984, #170293 ) ;
#216781=CARTESIAN_POINT ( 'NONE',  ( -18.50000000000000000, -9.400000000000005684, -7.297259759663287326 ) ) ;
#216786=EDGE_CURVE ( 'NONE', #162975, #140018, #66521, .T. ) ;
#216788=VECTOR ( 'NONE', #137530, 1000.000000000000000 ) ;
#216821=TOROIDAL_SURFACE ( 'NONE', #113339, 4.149999999999999467, 0.1000000000000000056 ) ;
#216863=CARTESIAN_POINT ( 'NONE',  ( -23.15000000000000213, 1.910280373831780176, -12.63136785519894012 ) ) ;
#216880=VERTEX_POINT ( 'NONE', #113341 ) ;
#216900=EDGE_LOOP ( 'NONE', ( #143095, #63689, #211164, #180693 ) ) ;
#216907=DIRECTION ( 'NONE',  ( 0.000000000000000000, 0.000000000000000000, -1.000000000000000000 ) ) ;
#216925=VECTOR ( 'NONE', #161041, 1000.000000000000000 ) ;
#216942=DIRECTION ( 'NONE',  ( -1.000000000000000000, -0.000000000000000000, -0.000000000000000000 ) ) ;
#216956=CIRCLE ( 'NONE', #104521, 0.1000000000000028644 ) ;
#216970=ORIENTED_EDGE ( 'NONE', *, *, #165431, .F. ) ;
#216975=CARTESIAN_POINT ( 'NONE',  ( 21.07189867249812210, 10.72498027009314825, -12.21245144227673940 ) ) ;
#216988=TOROIDAL_SURFACE ( 'NONE', #62889, 0.2000000000000000111, 0.1000000000000000056 ) ;
#216989=ORIENTED_EDGE ( 'NONE', *, *, #114602, .T. ) ;
#217012=CARTESIAN_POINT ( 'NONE',  ( 22.39999999999999503, 0.09999999999999939493, 7.790779598373383408 ) ) ;
#217056=DIRECTION ( 'NONE',  ( 0.000000000000000000, 0.000000000000000000, -1.000000000000000000 ) ) ;
#217110=DIRECTION ( 'NONE',  ( 0.000000000000000000, -0.000000000000000000, 1.000000000000000000 ) ) ;
#217165=EDGE_CURVE ( 'NONE', #59020, #244526, #53052, .T. ) ;
#217228=EDGE_LOOP ( 'NONE', ( #98607, #119776, #32788 ) ) ;
#217232=CARTESIAN_POINT ( 'NONE',  ( 20.94999999999999929, 4.850467289719617270, -12.03426740900167857 ) ) ;
#217256=ORIENTED_EDGE ( 'NONE', *, *, #242833, .T. ) ;
#217273=ORIENTED_EDGE ( 'NONE', *, *, #247089, .T. ) ;
#217286=CARTESIAN_POINT ( 'NONE',  ( -18.39999999999999858, -9.500000000000005329, -6.999285677838848585 ) ) ;
#217290=CARTESIAN_POINT ( 'NONE',  ( -22.47071067811865319, 7.720074744498064412, 0.09909245470260744093 ) ) ;
#217291=VERTEX_POINT ( 'NONE', #136411 ) ;
#217298=DIRECTION ( 'NONE',  ( 0.000000000000000000, 0.000000000000000000, -1.000000000000000000 ) ) ;
#217371=EDGE_CURVE ( 'NONE', #24982, #32549, #226656, .T. ) ;
#217379=ORIENTED_EDGE ( 'NONE', *, *, #42190, .T. ) ;
#217381=CARTESIAN_POINT ( 'NONE',  ( 21.05000000000000071, 0.000000000000000000, -37.60000000000000142 ) ) ;
#217400=EDGE_CURVE ( 'NONE', #63983, #197300, #101791, .T. ) ;
#217414=DIRECTION ( 'NONE',  ( -0.000000000000000000, 0.000000000000000000, -1.000000000000000000 ) ) ;
#217421=VERTEX_POINT ( 'NONE', #140273 ) ;
#217422=DIRECTION ( 'NONE',  ( 1.000000000000000000, 0.000000000000000000, -0.000000000000000000 ) ) ;
#217440=SPHERICAL_SURFACE ( 'NONE', #54518, 0.1000000000000000056 ) ;
#217452=CARTESIAN_POINT ( 'NONE',  ( 21.05000000000000071, 0.000000000000000000, -33.50000000000000000 ) ) ;
#217453=DIRECTION ( 'NONE',  ( 0.000000000000000000, 0.000000000000000000, -1.000000000000000000 ) ) ;
#217461=CARTESIAN_POINT ( 'NONE',  ( 18.49713797159854423, -9.446482327578955562, -7.071458121610131542 ) ) ;
#217475=ORIENTED_EDGE ( 'NONE', *, *, #42670, .F. ) ;
#217516=CARTESIAN_POINT ( 'NONE',  ( -23.25000000000000000, 4.150000000000001243, -12.35000000000000142 ) ) ;
#217526=ORIENTED_EDGE ( 'NONE', *, *, #28307, .T. ) ;
#217543=CARTESIAN_POINT ( 'NONE',  ( -21.12757541349819590, 0.005161215809727781600, 6.473380571251563964 ) ) ;
#217604=EDGE_LOOP ( 'NONE', ( #69329, #18779, #248267, #108272 ) ) ;
#217618=FACE_OUTER_BOUND ( 'NONE', #198258, .T. ) ;
#217624=CARTESIAN_POINT ( 'NONE',  ( 20.51284917709620359, 10.31088662284490631, -7.672473185591987210 ) ) ;
#217627=DIRECTION ( 'NONE',  ( 1.000000000000000000, 0.000000000000000000, 0.000000000000000000 ) ) ;
#217631=VERTEX_POINT ( 'NONE', #168892 ) ;
#217637=DIRECTION ( 'NONE',  ( 0.000000000000000000, -1.000000000000000000, -6.938893903907222067E-15 ) ) ;
#217655=CARTESIAN_POINT ( 'NONE',  ( -20.94999999999999929, 11.65000000000000036, -7.014805770654001016 ) ) ;
#217679=CARTESIAN_POINT ( 'NONE',  ( -21.05000000000000071, 1.736257131597397585, -11.56865232901749962 ) ) ;
#217700=B_SPLINE_CURVE_WITH_KNOTS ( 'NONE', 3,
 ( #144839, #4052, #224379, #108303, #24930, #86130, #125297, #105693, #242660, #66607 ),
 .UNSPECIFIED., .F., .F.,
 ( 4, 2, 2, 2, 4 ),
 ( 0.000000000000000000, 0.0001584437871625043689, 0.0002376656807437589386, 0.0002772766275343880801, 0.0003168875743250173030 ),
 .UNSPECIFIED. ) ;
#217716=DIRECTION ( 'NONE',  ( 0.000000000000000000, 0.000000000000000000, -1.000000000000000000 ) ) ;
#217717=VECTOR ( 'NONE', #230065, 1000.000000000000000 ) ;
#217736=DIRECTION ( 'NONE',  ( 0.000000000000000000, 1.000000000000000000, 0.000000000000000000 ) ) ;
#217759=DIRECTION ( 'NONE',  ( 1.000000000000000000, -0.000000000000000000, -0.000000000000000000 ) ) ;
#217765=CARTESIAN_POINT ( 'NONE',  ( -21.05000000000000071, -11.48912529307605901, -3.100000000000000533 ) ) ;
#217785=ORIENTED_EDGE ( 'NONE', *, *, #181744, .F. ) ;
#217788=CARTESIAN_POINT ( 'NONE',  ( -18.59999999999999787, -1.164121893241208960, -41.41484808557160591 ) ) ;
#217836=CIRCLE ( 'NONE', #134448, 0.09999999999999939493 ) ;
#217897=DIRECTION ( 'NONE',  ( 0.000000000000000000, 0.000000000000000000, -1.000000000000000000 ) ) ;
#217934=CARTESIAN_POINT ( 'NONE',  ( -23.25000000000000000, 4.349999999999999645, -12.25000000000000000 ) ) ;
#217945=DIRECTION ( 'NONE',  ( 0.000000000000000000, 0.9915357197604882655, -0.1298341882519793711 ) ) ;
#217969=ORIENTED_EDGE ( 'NONE', *, *, #60855, .F. ) ;
#218046=CARTESIAN_POINT ( 'NONE',  ( -18.39999999999999858, -9.500000000000005329, -40.10018939122204529 ) ) ;
#218050=ORIENTED_EDGE ( 'NONE', *, *, #124153, .T. ) ;
#218056=ORIENTED_EDGE ( 'NONE', *, *, #192364, .F. ) ;
#218070=ORIENTED_EDGE ( 'NONE', *, *, #252847, .T. ) ;
#218095=EDGE_CURVE ( 'NONE', #111006, #143109, #134679, .T. ) ;
#218099=EDGE_CURVE ( 'NONE', #237441, #183242, #108574, .T. ) ;
#218134=LINE ( 'NONE', #214311, #34853 ) ;
#218138=ADVANCED_FACE ( 'NONE', ( #191990 ), #152875, .T. ) ;
#218148=CARTESIAN_POINT ( 'NONE',  ( -20.85000000000000142, -11.75000000000000000, -33.50000000000000000 ) ) ;
#218178=DIRECTION ( 'NONE',  ( -1.000000000000000000, -0.000000000000000000, -0.000000000000000000 ) ) ;
#218184=ORIENTED_EDGE ( 'NONE', *, *, #90771, .F. ) ;
#218190=EDGE_LOOP ( 'NONE', ( #100713, #194519, #229967, #190762 ) ) ;
#218202=ORIENTED_EDGE ( 'NONE', *, *, #28283, .F. ) ;
#218224=CIRCLE ( 'NONE', #189038, 0.5000000000000022204 ) ;
#218228=LINE ( 'NONE', #39651, #249109 ) ;
#218249=VERTEX_POINT ( 'NONE', #101817 ) ;
#218315=CARTESIAN_POINT ( 'NONE',  ( 23.25000000000000000, -9.600000000000006750, 11.75000000000000000 ) ) ;
#218332=CARTESIAN_POINT ( 'NONE',  ( 20.94999999999999929, 0.000000000000000000, -35.40000000000000568 ) ) ;
#218337=CARTESIAN_POINT ( 'NONE',  ( 21.05000000000000071, 8.776282895292469632, -12.15000000000000036 ) ) ;
#218398=ADVANCED_FACE ( 'NONE', ( #149661 ), #50509, .F. ) ;
#218407=ORIENTED_EDGE ( 'NONE', *, *, #230112, .F. ) ;
#218436=FACE_OUTER_BOUND ( 'NONE', #191019, .T. ) ;
#218454=ORIENTED_EDGE ( 'NONE', *, *, #207303, .F. ) ;
#218504=CIRCLE ( 'NONE', #243468, 0.5000000000000004441 ) ;
#218511=ORIENTED_EDGE ( 'NONE', *, *, #196082, .T. ) ;
#218515=FACE_OUTER_BOUND ( 'NONE', #30489, .T. ) ;
#218517=LINE ( 'NONE', #93449, #110940 ) ;
#218544=EDGE_LOOP ( 'NONE', ( #42327, #153713, #168835, #233676 ) ) ;
#218584=DIRECTION ( 'NONE',  ( 1.000000000000000000, -0.000000000000000000, -0.000000000000000000 ) ) ;
#218588=ORIENTED_EDGE ( 'NONE', *, *, #91006, .T. ) ;
#218725=DIRECTION ( 'NONE',  ( 1.000000000000000000, 0.000000000000000000, 0.000000000000000000 ) ) ;
#218734=CARTESIAN_POINT ( 'NONE',  ( 22.50927854361889047, -0.1008580735255082683, 11.74956712602691233 ) ) ;
#218740=EDGE_CURVE ( 'NONE', #154965, #117101, #170232, .T. ) ;
#218750=AXIS2_PLACEMENT_3D ( 'NONE', #132513, #157236, #212062 ) ;
#218751=CARTESIAN_POINT ( 'NONE',  ( 18.49999999999999289, 11.65000000000000036, -33.50000000000000000 ) ) ;
#218754=DIRECTION ( 'NONE',  ( -4.336808689942053235E-15, -0.8660254037844482555, -0.4999999999999836797 ) ) ;
#218792=EDGE_CURVE ( 'NONE', #145230, #240969, #6053, .T. ) ;
#218793=DIRECTION ( 'NONE',  ( 1.000000000000000000, 0.000000000000000000, 0.000000000000000000 ) ) ;
#218809=DIRECTION ( 'NONE',  ( 0.000000000000000000, 0.000000000000000000, 1.000000000000000000 ) ) ;
#218830=CARTESIAN_POINT ( 'NONE',  ( -21.08035267497491816, 0.08268862477602348382, 6.331706839783040941 ) ) ;
#218835=EDGE_CURVE ( 'NONE', #254325, #79894, #185139, .T. ) ;
#218859=DIRECTION ( 'NONE',  ( -0.000000000000000000, -0.000000000000000000, 1.000000000000000000 ) ) ;
#218917=DIRECTION ( 'NONE',  ( 0.000000000000000000, 0.9915357197604883766, -0.1298341882519788160 ) ) ;
#218920=CARTESIAN_POINT ( 'NONE',  ( 20.74897398619109268, 10.59569302166641336, -7.679311456256082913 ) ) ;
#218931=EDGE_LOOP ( 'NONE', ( #85246, #153845, #246763, #121780, #224871, #190628, #125353, #101015, #164785, #81750 ) ) ;
#218951=CARTESIAN_POINT ( 'NONE',  ( 23.14999999999999858, 0.000000000000000000, -33.50000000000000000 ) ) ;
#218953=FACE_OUTER_BOUND ( 'NONE', #104365, .T. ) ;
#218958=EDGE_CURVE ( 'NONE', #177256, #139796, #72748, .T. ) ;
#218962=ORIENTED_EDGE ( 'NONE', *, *, #82963, .T. ) ;
#218975=CARTESIAN_POINT ( 'NONE',  ( 21.05000000000000071, 1.360870587192041681, -8.072997927090961312 ) ) ;
#218980=CARTESIAN_POINT ( 'NONE',  ( 20.85000000000000142, 0.000000000000000000, -33.50000000000000000 ) ) ;
#219014=FACE_OUTER_BOUND ( 'NONE', #129566, .T. ) ;
#219021=AXIS2_PLACEMENT_3D ( 'NONE', #198072, #98945, #199381 ) ;
#219022=CARTESIAN_POINT ( 'NONE',  ( 23.24999999999999289, 6.450000000000001066, 11.75000000000000000 ) ) ;
#219026=SPHERICAL_SURFACE ( 'NONE', #152347, 0.1000000000000000056 ) ;
#219088=DIRECTION ( 'NONE',  ( -7.304098846218134667E-16, -1.000000000000000000, 0.000000000000000000 ) ) ;
#219098=AXIS2_PLACEMENT_3D ( 'NONE', #215884, #252449, #116812 ) ;
#219104=AXIS2_PLACEMENT_3D ( 'NONE', #112285, #133121, #156565 ) ;
#219105=EDGE_CURVE ( 'NONE', #20887, #72537, #162193, .T. ) ;
#219109=CARTESIAN_POINT ( 'NONE',  ( 20.95325940946048249, 10.52339007069628707, -7.564462129240085986 ) ) ;
#219202=ORIENTED_EDGE ( 'NONE', *, *, #210509, .T. ) ;
#219323=VERTEX_POINT ( 'NONE', #66480 ) ;
#219331=EDGE_CURVE ( 'NONE', #94835, #235074, #89442, .T. ) ;
#219381=VERTEX_POINT ( 'NONE', #89876 ) ;
#219420=CIRCLE ( 'NONE', #65319, 0.2000000000000000944 ) ;
#219422=CARTESIAN_POINT ( 'NONE',  ( -20.94999999999999929, -11.39257802170567224, -3.073949579831933843 ) ) ;
#219424=DIRECTION ( 'NONE',  ( 0.000000000000000000, 0.000000000000000000, -1.000000000000000000 ) ) ;
#219425=CIRCLE ( 'NONE', #177777, 0.09999999999999939493 ) ;
#219429=DIRECTION ( 'NONE',  ( -1.000000000000000000, 0.000000000000000000, 0.000000000000000000 ) ) ;
#219442=ADVANCED_FACE ( 'NONE', ( #172037 ), #72932, .F. ) ;
#219453=VECTOR ( 'NONE', #135614, 1000.000000000000000 ) ;
#219499=VECTOR ( 'NONE', #174340, 999.9999999999998863 ) ;
#219506=AXIS2_PLACEMENT_3D ( 'NONE', #31872, #188349, #86647 ) ;
#219512=CYLINDRICAL_SURFACE ( 'NONE', #16232, 0.09999999999999939493 ) ;
#219537=DIRECTION ( 'NONE',  ( 0.000000000000000000, 0.000000000000000000, 1.000000000000000000 ) ) ;
#219538=DIRECTION ( 'NONE',  ( -1.000000000000000000, -0.000000000000000000, -0.000000000000000000 ) ) ;
#219539=EDGE_CURVE ( 'NONE', #122037, #60900, #239670, .T. ) ;
#219560=AXIS2_PLACEMENT_3D ( 'NONE', #78160, #22071, #241124 ) ;
#219618=AXIS2_PLACEMENT_3D ( 'NONE', #94655, #95928, #174247 ) ;
#219619=TOROIDAL_SURFACE ( 'NONE', #15672, 12.77499999999999858, 0.1000000000000000056 ) ;
#219666=DIRECTION ( 'NONE',  ( 1.000000000000000000, 0.000000000000000000, 0.000000000000000000 ) ) ;
#219691=ORIENTED_EDGE ( 'NONE', *, *, #119559, .F. ) ;
#219701=AXIS2_PLACEMENT_3D ( 'NONE', #33424, #210737, #51625 ) ;
#219704=ORIENTED_EDGE ( 'NONE', *, *, #116788, .T. ) ;
#219737=ORIENTED_EDGE ( 'NONE', *, *, #91006, .F. ) ;
#219763=CIRCLE ( 'NONE', #3275, 11.65000000000000036 ) ;
#219764=DIRECTION ( 'NONE',  ( 0.000000000000000000, 0.000000000000000000, -1.000000000000000000 ) ) ;
#219800=VERTEX_POINT ( 'NONE', #136545 ) ;
#219820=DIRECTION ( 'NONE',  ( -1.000000000000000000, -2.952720810173289112E-16, 0.000000000000000000 ) ) ;
#219841=CARTESIAN_POINT ( 'NONE',  ( -21.05000000000000071, 11.64999999999999680, -0.1000000000000028644 ) ) ;
#219849=DIRECTION ( 'NONE',  ( 0.000000000000000000, 0.000000000000000000, 1.000000000000000000 ) ) ;
#219920=EDGE_LOOP ( 'NONE', ( #114651, #112970, #125721, #94613 ) ) ;
#219946=DIRECTION ( 'NONE',  ( -0.000000000000000000, -0.000000000000000000, -1.000000000000000000 ) ) ;
#219947=ORIENTED_EDGE ( 'NONE', *, *, #241196, .F. ) ;
#219982=DIRECTION ( 'NONE',  ( 2.915501640297155269E-16, -1.000000000000000000, 0.000000000000000000 ) ) ;
#220003=FACE_OUTER_BOUND ( 'NONE', #245574, .T. ) ;
#220029=CARTESIAN_POINT ( 'NONE',  ( 21.05000000000000071, 0.05148288188168551049, 6.300179817914542291 ) ) ;
#220050=EDGE_CURVE ( 'NONE', #223036, #18401, #76172, .T. ) ;
#220131=CARTESIAN_POINT ( 'NONE',  ( 20.94999999999999929, 4.999999999999997335, -12.40526601891309788 ) ) ;
#220132=ADVANCED_FACE ( 'NONE', ( #34299 ), #55082, .F. ) ;
#220159=FACE_OUTER_BOUND ( 'NONE', #198212, .T. ) ;
#220161=CARTESIAN_POINT ( 'NONE',  ( -21.05000000000000071, -11.75000000000000000, -30.50000000000000000 ) ) ;
#220186=ORIENTED_EDGE ( 'NONE', *, *, #42276, .F. ) ;
#220206=EDGE_CURVE ( 'NONE', #224018, #174229, #2688, .T. ) ;
#220207=ORIENTED_EDGE ( 'NONE', *, *, #51178, .F. ) ;
#220221=ADVANCED_FACE ( 'NONE', ( #62814, #139762 ), #21152, .T. ) ;
#220225=ORIENTED_EDGE ( 'NONE', *, *, #102475, .F. ) ;
#220271=CARTESIAN_POINT ( 'NONE',  ( 20.94999999999999929, -9.500000000000000000, -23.60603087734755690 ) ) ;
#220287=EDGE_CURVE ( 'NONE', #178738, #170516, #152590, .T. ) ;
#220319=VECTOR ( 'NONE', #134039, 1000.000000000000000 ) ;
#220320=CIRCLE ( 'NONE', #107867, 0.09999999999999993616 ) ;
#220341=CONICAL_SURFACE ( 'NONE', #145480, 4.049999999999998934, 0.7853981633974604915 ) ;
#220385=VERTEX_POINT ( 'NONE', #44549 ) ;
#220399=ADVANCED_FACE ( 'NONE', ( #45820 ), #204879, .F. ) ;
#220404=FACE_OUTER_BOUND ( 'NONE', #60156, .T. ) ;
#220448=B_SPLINE_CURVE_WITH_KNOTS ( 'NONE', 3,
 ( #248651, #33502, #111709, #231676, #249940, #28362, #71323, #212108, #112998, #152147 ),
 .UNSPECIFIED., .F., .F.,
 ( 4, 3, 3, 4 ),
 ( 4.906538933386797396E-18, 0.0002000000000002859679, 0.001000000000045107602, 0.001967863649472130407 ),
 .UNSPECIFIED. ) ;
#220449=ORIENTED_EDGE ( 'NONE', *, *, #241044, .T. ) ;
#220459=CIRCLE ( 'NONE', #8077, 0.09999999999999939493 ) ;
#220461=DIRECTION ( 'NONE',  ( 1.000000000000000000, 0.000000000000000000, -0.000000000000000000 ) ) ;
#220463=VERTEX_POINT ( 'NONE', #113498 ) ;
#220493=DIRECTION ( 'NONE',  ( 0.000000000000000000, -0.4930308989875248349, -0.8700118002898312719 ) ) ;
#220533=ORIENTED_EDGE ( 'NONE', *, *, #107077, .T. ) ;
#220543=CYLINDRICAL_SURFACE ( 'NONE', #187416, 0.09999999999999939493 ) ;
#220544=EDGE_LOOP ( 'NONE', ( #26978, #83400, #92858, #46323 ) ) ;
#220547=ORIENTED_EDGE ( 'NONE', *, *, #231477, .F. ) ;
#220553=CARTESIAN_POINT ( 'NONE',  ( -21.14999999999999858, 6.540656951701240729, -0.09999999999999939493 ) ) ;
#220562=LINE ( 'NONE', #22380, #205522 ) ;
#220599=CARTESIAN_POINT ( 'NONE',  ( 23.24999999999999645, 3.899999999999999467, -33.50000000000000000 ) ) ;
#220659=DIRECTION ( 'NONE',  ( 0.000000000000000000, 0.000000000000000000, -1.000000000000000000 ) ) ;
#220676=ORIENTED_EDGE ( 'NONE', *, *, #119559, .T. ) ;
#220682=CARTESIAN_POINT ( 'NONE',  ( -20.88420186297724257, 10.33025634371521662, -39.08709292826387838 ) ) ;
#220702=ORIENTED_EDGE ( 'NONE', *, *, #192808, .T. ) ;
#220716=CARTESIAN_POINT ( 'NONE',  ( 20.85000000000000142, -1.263275465217258198, -41.40186466674640542 ) ) ;
#220726=DIRECTION ( 'NONE',  ( 1.000000000000000000, 0.000000000000000000, -0.000000000000000000 ) ) ;
#220759=CIRCLE ( 'NONE', #70764, 0.09999999999999939493 ) ;
#220776=DIRECTION ( 'NONE',  ( 0.7071067811865475727, 0.7071067811865475727, 0.000000000000000000 ) ) ;
#220830=DIRECTION ( 'NONE',  ( 0.000000000000000000, -1.000000000000000000, 0.000000000000000000 ) ) ;
#220857=CARTESIAN_POINT ( 'NONE',  ( -21.05000000000000071, 11.59999999999999787, -26.57179676972450011 ) ) ;
#220866=DIRECTION ( 'NONE',  ( 1.000000000000000000, 0.000000000000000000, -0.000000000000000000 ) ) ;
#220867=FACE_OUTER_BOUND ( 'NONE', #241760, .T. ) ;
#220877=EDGE_CURVE ( 'NONE', #99784, #74339, #243717, .T. ) ;
#220975=DIRECTION ( 'NONE',  ( 0.000000000000000000, -0.8660254037844411501, -0.4999999999999956701 ) ) ;
#220988=CARTESIAN_POINT ( 'NONE',  ( 18.51697539158856642, 10.31565961586830760, -39.03641941191783360 ) ) ;
#220992=CARTESIAN_POINT ( 'NONE',  ( 20.94999999999999929, 5.399999999999998579, -23.60603087734755690 ) ) ;
#220993=LINE ( 'NONE', #42372, #36597 ) ;
#221000=ORIENTED_EDGE ( 'NONE', *, *, #74192, .T. ) ;
#221017=VERTEX_POINT ( 'NONE', #158763 ) ;
#221025=EDGE_CURVE ( 'NONE', #244526, #190309, #238261, .T. ) ;
#221035=EDGE_LOOP ( 'NONE', ( #626, #146917, #67510, #26370 ) ) ;
#221063=EDGE_LOOP ( 'NONE', ( #92519, #180689, #30049, #249222, #11683 ) ) ;
#221069=DIRECTION ( 'NONE',  ( -0.000000000000000000, -0.000000000000000000, -1.000000000000000000 ) ) ;
#221075=CYLINDRICAL_SURFACE ( 'NONE', #33958, 11.79999999999999716 ) ;
#221083=CARTESIAN_POINT ( 'NONE',  ( -18.50000000000000000, 9.250000000000001776, -12.34999999999999964 ) ) ;
#221102=DIRECTION ( 'NONE',  ( 1.000000000000000000, -0.000000000000000000, -0.000000000000000000 ) ) ;
#221141=DIRECTION ( 'NONE',  ( 0.000000000000000000, 3.469446951953614189E-14, 1.000000000000000000 ) ) ;
#221183=EDGE_CURVE ( 'NONE', #54887, #210905, #146847, .T. ) ;
#221224=FACE_OUTER_BOUND ( 'NONE', #240197, .T. ) ;
#221247=EDGE_CURVE ( 'NONE', #192659, #103735, #54180, .T. ) ;
#221255=FACE_OUTER_BOUND ( 'NONE', #245783, .T. ) ;
#221263=AXIS2_PLACEMENT_3D ( 'NONE', #32468, #92390, #192796 ) ;
#221273=EDGE_CURVE ( 'NONE', #245627, #83974, #234090, .T. ) ;
#221287=EDGE_LOOP ( 'NONE', ( #73974, #74857, #380, #119704 ) ) ;
#221291=CARTESIAN_POINT ( 'NONE',  ( -18.59999999999999787, -1.162701749938009677, -8.099999999999999645 ) ) ;
#221314=ADVANCED_FACE ( 'NONE', ( #52898 ), #171605, .F. ) ;
#221317=ORIENTED_EDGE ( 'NONE', *, *, #104446, .F. ) ;
#221330=EDGE_LOOP ( 'NONE', ( #228788, #112565, #222998, #121793 ) ) ;
#221331=FACE_OUTER_BOUND ( 'NONE', #55791, .T. ) ;
#221337=ORIENTED_EDGE ( 'NONE', *, *, #92670, .T. ) ;
#221353=FACE_OUTER_BOUND ( 'NONE', #32841, .T. ) ;
#221365=DIRECTION ( 'NONE',  ( -1.000000000000000000, -2.952720810173289112E-16, 0.000000000000000000 ) ) ;
#221373=DIRECTION ( 'NONE',  ( 1.000000000000000000, 2.952720810173289112E-16, -0.000000000000000000 ) ) ;
#221376=DIRECTION ( 'NONE',  ( 0.000000000000000000, 0.000000000000000000, -1.000000000000000000 ) ) ;
#221380=DIRECTION ( 'NONE',  ( 0.000000000000000000, -1.000000000000000000, 6.308085367188393199E-16 ) ) ;
#221390=AXIS2_PLACEMENT_3D ( 'NONE', #243079, #125701, #205223 ) ;
#221410=CARTESIAN_POINT ( 'NONE',  ( -22.47007471830798409, 7.720710651926475876, 8.715969027246751475E-16 ) ) ;
#221418=EDGE_LOOP ( 'NONE', ( #11697, #72989, #81905, #188079 ) ) ;
#221435=AXIS2_PLACEMENT_3D ( 'NONE', #104093, #147079, #162832 ) ;
#221451=ORIENTED_EDGE ( 'NONE', *, *, #128981, .F. ) ;
#221455=DIRECTION ( 'NONE',  ( -1.000000000000000000, 0.000000000000000000, -3.469446951953635015E-14 ) ) ;
#221461=DIRECTION ( 'NONE',  ( 0.000000000000000000, 0.000000000000000000, -1.000000000000000000 ) ) ;
#221500=( BOUNDED_CURVE ( )  B_SPLINE_CURVE ( 3, ( #45167, #225067, #8619, #67300 ),
 .UNSPECIFIED., .F., .F. ) 
 B_SPLINE_CURVE_WITH_KNOTS ( ( 4, 4 ),
 ( 3.141592653589791784, 4.712388980384688786 ),
 .UNSPECIFIED. ) 
 CURVE ( )  GEOMETRIC_REPRESENTATION_ITEM ( )  RATIONAL_B_SPLINE_CURVE ( ( 1.000000000000000000, 0.8047378541243649375, 0.8047378541243649375, 1.000000000000000000 ) ) 
 REPRESENTATION_ITEM ( '' )  );
#221534=DIRECTION ( 'NONE',  ( 1.000000000000000000, 0.000000000000000000, 0.000000000000000000 ) ) ;
#221564=DIRECTION ( 'NONE',  ( 0.000000000000000000, -0.1568667991644863147, -0.9876197685951252359 ) ) ;
#221568=EDGE_CURVE ( 'NONE', #66968, #57845, #198876, .T. ) ;
#221577=DIRECTION ( 'NONE',  ( 1.000000000000000000, -0.000000000000000000, -0.000000000000000000 ) ) ;
#221592=CIRCLE ( 'NONE', #229994, 0.09999999999999939493 ) ;
#221604=DIRECTION ( 'NONE',  ( 1.000000000000000000, 0.000000000000000000, 0.000000000000000000 ) ) ;
#221610=ORIENTED_EDGE ( 'NONE', *, *, #197743, .T. ) ;
#221619=CARTESIAN_POINT ( 'NONE',  ( 21.05000000000000071, -8.663551401869154844, -23.97589888193268948 ) ) ;
#221671=CARTESIAN_POINT ( 'NONE',  ( -23.15000000000000213, 0.000000000000000000, 0.000000000000000000 ) ) ;
#221673=EDGE_CURVE ( 'NONE', #233325, #167773, #234770, .T. ) ;
#221680=EDGE_LOOP ( 'NONE', ( #138026, #39647, #76027, #86981, #64846 ) ) ;
#221739=LINE ( 'NONE', #142225, #256605 ) ;
#221742=VECTOR ( 'NONE', #110376, 1000.000000000000114 ) ;
#221773=ORIENTED_EDGE ( 'NONE', *, *, #182837, .F. ) ;
#221779=CARTESIAN_POINT ( 'NONE',  ( -21.14999999999999858, 11.75000000000000000, -0.1000000000000028644 ) ) ;
#221785=AXIS2_PLACEMENT_3D ( 'NONE', #228124, #230692, #54598 ) ;
#221794=CARTESIAN_POINT ( 'NONE',  ( -20.85000000000000142, -1.362429037193307435, -41.38888124792119783 ) ) ;
#221832=ADVANCED_FACE ( 'NONE', ( #62559 ), #138210, .F. ) ;
#221906=TOROIDAL_SURFACE ( 'NONE', #59582, 1.900000000000002576, 0.1000000000000000056 ) ;
#221936=CARTESIAN_POINT ( 'NONE',  ( 18.59999999999999076, 11.65000000000000391, -24.85000000000000142 ) ) ;
#221984=ORIENTED_EDGE ( 'NONE', *, *, #60524, .T. ) ;
#222087=FACE_OUTER_BOUND ( 'NONE', #202690, .T. ) ;
#222091=DIRECTION ( 'NONE',  ( 1.000000000000000000, 0.000000000000000000, 0.000000000000000000 ) ) ;
#222095=CARTESIAN_POINT ( 'NONE',  ( 20.94999999999999574, -11.41227409414968719, -3.000000000000002665 ) ) ;
#222110=CARTESIAN_POINT ( 'NONE',  ( -18.57399277249657032, 10.33112638555853913, -39.09012289269747953 ) ) ;
#222114=DIRECTION ( 'NONE',  ( -0.7071067811865475727, -0.7071067811865475727, -0.000000000000000000 ) ) ;
#222115=ORIENTED_EDGE ( 'NONE', *, *, #192484, .F. ) ;
#222116=EDGE_LOOP ( 'NONE', ( #166659, #238444, #228772, #257893, #247492 ) ) ;
#222117=CARTESIAN_POINT ( 'NONE',  ( -21.02374657821575354, 11.60000000082034433, -26.57179677019813013 ) ) ;
#222139=ORIENTED_EDGE ( 'NONE', *, *, #223359, .F. ) ;
#222141=FACE_OUTER_BOUND ( 'NONE', #186130, .T. ) ;
#222146=ADVANCED_FACE ( 'NONE', ( #190212 ), #153511, .F. ) ;
#222167=SPHERICAL_SURFACE ( 'NONE', #3628, 0.1000000000000000056 ) ;
#222169=DIRECTION ( 'NONE',  ( 0.000000000000000000, 1.000000000000000000, 2.891205793294679805E-16 ) ) ;
#222173=CIRCLE ( 'NONE', #109763, 0.1000000000000028644 ) ;
#222174=DIRECTION ( 'NONE',  ( 1.000000000000000000, 0.000000000000000000, 0.000000000000000000 ) ) ;
#222187=CARTESIAN_POINT ( 'NONE',  ( -23.15000000000000213, 0.000000000000000000, -35.60000000000000853 ) ) ;
#222197=ORIENTED_EDGE ( 'NONE', *, *, #55829, .T. ) ;
#222217=DIRECTION ( 'NONE',  ( -0.000000000000000000, 0.000000000000000000, -1.000000000000000000 ) ) ;
#222226=DIRECTION ( 'NONE',  ( 0.000000000000000000, 0.000000000000000000, 1.000000000000000000 ) ) ;
#222229=FACE_OUTER_BOUND ( 'NONE', #139322, .T. ) ;
#222246=DIRECTION ( 'NONE',  ( 0.000000000000000000, 0.000000000000000000, -1.000000000000000000 ) ) ;
#222255=CARTESIAN_POINT ( 'NONE',  ( 18.54148534481893762, 10.32532329026771123, -39.06993430183595706 ) ) ;
#222304=LINE ( 'NONE', #123239, #226291 ) ;
#222330=ORIENTED_EDGE ( 'NONE', *, *, #107077, .F. ) ;
#222379=ORIENTED_EDGE ( 'NONE', *, *, #154771, .T. ) ;
#222405=CARTESIAN_POINT ( 'NONE',  ( -23.15000000000000213, 0.000000000000000000, -33.50000000000000000 ) ) ;
#222421=ORIENTED_EDGE ( 'NONE', *, *, #23685, .F. ) ;
#222450=CARTESIAN_POINT ( 'NONE',  ( 20.94999999999999574, -11.64999999999999147, -3.100000000000001865 ) ) ;
#222477=EDGE_CURVE ( 'NONE', #242536, #61026, #161471, .T. ) ;
#222481=DIRECTION ( 'NONE',  ( 0.000000000000000000, 1.000000000000000000, 0.000000000000000000 ) ) ;
#222483=EDGE_CURVE ( 'NONE', #130735, #31072, #66156, .T. ) ;
#222484=ORIENTED_EDGE ( 'NONE', *, *, #85959, .T. ) ;
#222538=CARTESIAN_POINT ( 'NONE',  ( -18.59999999999999787, 0.000000000000000000, -33.50000000000000000 ) ) ;
#222554=ORIENTED_EDGE ( 'NONE', *, *, #100010, .T. ) ;
#222576=CARTESIAN_POINT ( 'NONE',  ( 20.94999999999999929, 0.000000000000000000, -37.60000000000000142 ) ) ;
#222611=CARTESIAN_POINT ( 'NONE',  ( -21.05000000000000071, 11.63687328910405938, -6.821759213324853022 ) ) ;
#222633=ORIENTED_EDGE ( 'NONE', *, *, #35184, .F. ) ;
#222660=DIRECTION ( 'NONE',  ( 0.000000000000000000, 0.000000000000000000, -1.000000000000000000 ) ) ;
#222673=FACE_OUTER_BOUND ( 'NONE', #166975, .T. ) ;
#222675=ORIENTED_EDGE ( 'NONE', *, *, #169165, .F. ) ;
#222686=CARTESIAN_POINT ( 'NONE',  ( -21.44999999999999929, 7.349999999999998757, -12.34999999999999964 ) ) ;
#222703=CARTESIAN_POINT ( 'NONE',  ( 19.75857864376268935, 11.65000000000000391, -24.85000000000000142 ) ) ;
#222728=ORIENTED_EDGE ( 'NONE', *, *, #100861, .T. ) ;
#222744=DIRECTION ( 'NONE',  ( 1.000000000000000000, -0.000000000000000000, -0.000000000000000000 ) ) ;
#222745=EDGE_CURVE ( 'NONE', #32887, #201638, #69900, .T. ) ;
#222757=ADVANCED_FACE ( 'NONE', ( #35965 ), #257502, .F. ) ;
#222761=ORIENTED_EDGE ( 'NONE', *, *, #169699, .F. ) ;
#222777=EDGE_LOOP ( 'NONE', ( #254235, #51800, #101902, #21771 ) ) ;
#222778=CARTESIAN_POINT ( 'NONE',  ( 21.05000000000000071, 6.477067021124756963, -0.09999999999999967248 ) ) ;
#222783=FACE_OUTER_BOUND ( 'NONE', #234935, .T. ) ;
#222802=AXIS2_PLACEMENT_3D ( 'NONE', #95983, #236782, #213367 ) ;
#222808=VERTEX_POINT ( 'NONE', #240573 ) ;
#222843=EDGE_CURVE ( 'NONE', #33602, #74587, #141467, .T. ) ;
#222853=EDGE_CURVE ( 'NONE', #164389, #16503, #220993, .T. ) ;
#222855=AXIS2_PLACEMENT_3D ( 'NONE', #242565, #220461, #100466 ) ;
#222918=AXIS2_PLACEMENT_3D ( 'NONE', #72284, #73588, #209205 ) ;
#222931=ORIENTED_EDGE ( 'NONE', *, *, #29701, .F. ) ;
#222951=EDGE_LOOP ( 'NONE', ( #218511, #192874, #9031, #2720 ) ) ;
#222962=ADVANCED_FACE ( 'NONE', ( #68365 ), #129621, .T. ) ;
#222977=ORIENTED_EDGE ( 'NONE', *, *, #198849, .T. ) ;
#222998=ORIENTED_EDGE ( 'NONE', *, *, #257768, .F. ) ;
#223024=EDGE_CURVE ( 'NONE', #217291, #199045, #128334, .T. ) ;
#223032=ORIENTED_EDGE ( 'NONE', *, *, #151126, .T. ) ;
#223036=VERTEX_POINT ( 'NONE', #51329 ) ;
#223049=ORIENTED_EDGE ( 'NONE', *, *, #135045, .T. ) ;
#223064=EDGE_CURVE ( 'NONE', #55133, #235552, #57384, .T. ) ;
#223070=AXIS2_PLACEMENT_3D ( 'NONE', #148879, #228418, #193139 ) ;
#223081=ORIENTED_EDGE ( 'NONE', *, *, #52512, .F. ) ;
#223084=VECTOR ( 'NONE', #208674, 1000.000000000000000 ) ;
#223091=FACE_OUTER_BOUND ( 'NONE', #179933, .T. ) ;
#223097=DIRECTION ( 'NONE',  ( -2.252264143451594314E-15, -0.1298341882520124002, -0.9915357197604841577 ) ) ;
#223098=ORIENTED_EDGE ( 'NONE', *, *, #126989, .T. ) ;
#223116=ADVANCED_FACE ( 'NONE', ( #119050 ), #173930, .T. ) ;
#223121=ORIENTED_EDGE ( 'NONE', *, *, #245277, .T. ) ;
#223142=CARTESIAN_POINT ( 'NONE',  ( 21.07928932188134397, 0.09889514565439641580, 6.328516656393307294 ) ) ;
#223144=DIRECTION ( 'NONE',  ( 0.000000000000000000, 0.000000000000000000, -1.000000000000000000 ) ) ;
#223148=DIRECTION ( 'NONE',  ( 0.000000000000000000, 0.000000000000000000, 1.000000000000000000 ) ) ;
#223199=CIRCLE ( 'NONE', #64987, 0.09999999999999939493 ) ;
#223228=CARTESIAN_POINT ( 'NONE',  ( -20.94999675878240808, 10.29307482167955357, -38.95864214669402514 ) ) ;
#223263=CARTESIAN_POINT ( 'NONE',  ( -18.50000000000000000, 11.64999999999999680, -7.014805770654001016 ) ) ;
#223265=DIRECTION ( 'NONE',  ( -1.000000000000000000, 0.000000000000000000, 0.000000000000000000 ) ) ;
#223277=FACE_OUTER_BOUND ( 'NONE', #38770, .T. ) ;
#223280=FACE_OUTER_BOUND ( 'NONE', #221330, .T. ) ;
#223283=ORIENTED_EDGE ( 'NONE', *, *, #255058, .T. ) ;
#223302=ORIENTED_EDGE ( 'NONE', *, *, #53180, .T. ) ;
#223329=EDGE_CURVE ( 'NONE', #237621, #233645, #36963, .T. ) ;
#223333=VERTEX_POINT ( 'NONE', #118617 ) ;
#223345=CIRCLE ( 'NONE', #85958, 0.09999999999999939493 ) ;
#223359=EDGE_CURVE ( 'NONE', #94374, #124226, #32693, .T. ) ;
#223393=LINE ( 'NONE', #222095, #186025 ) ;
#223398=ORIENTED_EDGE ( 'NONE', *, *, #215010, .F. ) ;
#223407=CARTESIAN_POINT ( 'NONE',  ( -18.59117750673696889, 10.33248238082519066, -39.09484654391314962 ) ) ;
#223410=DIRECTION ( 'NONE',  ( 1.000000000000000000, 0.000000000000000000, 0.000000000000000000 ) ) ;
#223416=CARTESIAN_POINT ( 'NONE',  ( -20.85000000106584750, 11.74999999999999645, -26.65550465647363154 ) ) ;
#223419=ORIENTED_EDGE ( 'NONE', *, *, #144375, .F. ) ;
#223441=DIRECTION ( 'NONE',  ( -3.265361837132813093E-16, 1.000000000000000000, 0.000000000000000000 ) ) ;
#223444=ORIENTED_EDGE ( 'NONE', *, *, #142834, .F. ) ;
#223464=CARTESIAN_POINT ( 'NONE',  ( 21.05000000000000071, 10.42338541491290727, -7.492051923870097774 ) ) ;
#223470=AXIS2_PLACEMENT_3D ( 'NONE', #184452, #85329, #164900 ) ;
#223481=ORIENTED_EDGE ( 'NONE', *, *, #243284, .T. ) ;
#223553=DIRECTION ( 'NONE',  ( 6.938893903907030216E-14, 0.000000000000000000, 1.000000000000000000 ) ) ;
#223576=DIRECTION ( 'NONE',  ( 0.000000000000000000, -0.9908441862701596881, -0.1350103645451904977 ) ) ;
#223605=ADVANCED_FACE ( 'NONE', ( #12316 ), #247031, .F. ) ;
#223629=EDGE_CURVE ( 'NONE', #223036, #228001, #107645, .T. ) ;
#223647=CIRCLE ( 'NONE', #73859, 11.75000000000000000 ) ;
#223649=CIRCLE ( 'NONE', #169558, 0.09999999999999939493 ) ;
#223656=ORIENTED_EDGE ( 'NONE', *, *, #7672, .F. ) ;
#223658=DIRECTION ( 'NONE',  ( 0.000000000000000000, 0.000000000000000000, -1.000000000000000000 ) ) ;
#223661=CARTESIAN_POINT ( 'NONE',  ( -20.54999999999999716, 1.999999999999998224, -13.22462192276210224 ) ) ;
#223663=VECTOR ( 'NONE', #152748, 1000.000000000000000 ) ;
#223687=LINE ( 'NONE', #29399, #58846 ) ;
#223706=CARTESIAN_POINT ( 'NONE',  ( -23.15000000000000213, 4.959819536546777642E-16, 4.049999999999998934 ) ) ;
#223752=DIRECTION ( 'NONE',  ( -0.7070776581708965169, -0.7071359030027827286, -0.000000000000000000 ) ) ;
#223775=CIRCLE ( 'NONE', #7304, 0.1000000000000002970 ) ;
#223779=CIRCLE ( 'NONE', #140997, 0.09999999999999939493 ) ;
#223790=DIRECTION ( 'NONE',  ( -1.000000000000000000, -2.952720810173289112E-16, 0.000000000000000000 ) ) ;
#223823=CARTESIAN_POINT ( 'NONE',  ( -18.54159361262949091, -9.463132135493086849, -7.049122216292921905 ) ) ;
#223826=DIRECTION ( 'NONE',  ( 0.000000000000000000, -1.000000000000000000, 0.000000000000000000 ) ) ;
#223843=CARTESIAN_POINT ( 'NONE',  ( -20.64999999999999858, -9.000000000000001776, -23.60603087734756045 ) ) ;
#223867=EDGE_LOOP ( 'NONE', ( #168216, #75813, #122335, #244406 ) ) ;
#223885=DIRECTION ( 'NONE',  ( 0.000000000000000000, -1.000000000000000000, 6.308085367188393199E-16 ) ) ;
#223889=CYLINDRICAL_SURFACE ( 'NONE', #2401, 0.09999999999999939493 ) ;
#223903=ORIENTED_EDGE ( 'NONE', *, *, #223024, .T. ) ;
#223954=CARTESIAN_POINT ( 'NONE',  ( 21.13461538461538325, 8.885417037974459475, -12.35000000000000320 ) ) ;
#223969=ORIENTED_EDGE ( 'NONE', *, *, #58089, .T. ) ;
#223973=CIRCLE ( 'NONE', #199053, 0.6000000000000015321 ) ;
#223999=DIRECTION ( 'NONE',  ( 0.000000000000000000, -1.000000000000000000, -2.891205793294679805E-16 ) ) ;
#224009=CARTESIAN_POINT ( 'NONE',  ( -22.39999999999999858, 0.000000000000000000, 7.790779598373403836 ) ) ;
#224010=VERTEX_POINT ( 'NONE', #86352 ) ;
#224012=CARTESIAN_POINT ( 'NONE',  ( 20.94999999999999574, 1.835341550224413698, -11.55515129256298046 ) ) ;
#224016=ORIENTED_EDGE ( 'NONE', *, *, #75807, .T. ) ;
#224018=VERTEX_POINT ( 'NONE', #165952 ) ;
#224046=VECTOR ( 'NONE', #80640, 1000.000000000000000 ) ;
#224064=DIRECTION ( 'NONE',  ( 1.000000000000000000, 0.000000000000000000, 0.000000000000000000 ) ) ;
#224070=CIRCLE ( 'NONE', #169965, 0.09999999999999939493 ) ;
#224091=AXIS2_PLACEMENT_3D ( 'NONE', #158225, #162053, #220726 ) ;
#224093=VECTOR ( 'NONE', #1493, 1000.000000000000000 ) ;
#224101=CARTESIAN_POINT ( 'NONE',  ( 18.49999999999999645, -1.835859311443640340, -45.00443916879852679 ) ) ;
#224112=DIRECTION ( 'NONE',  ( 0.000000000000000000, 0.000000000000000000, -1.000000000000000000 ) ) ;
#224118=LINE ( 'NONE', #45491, #109389 ) ;
#224126=DIRECTION ( 'NONE',  ( 1.000000000000000000, 0.000000000000000000, 0.000000000000000000 ) ) ;
#224147=DIRECTION ( 'NONE',  ( -1.000000000000000000, 0.000000000000000000, 0.000000000000000000 ) ) ;
#224207=DIRECTION ( 'NONE',  ( 1.000000000000000000, 0.000000000000000000, 0.000000000000000000 ) ) ;
#224214=ORIENTED_EDGE ( 'NONE', *, *, #85522, .F. ) ;
#224219=CARTESIAN_POINT ( 'NONE',  ( 20.04142135391667168, 11.75000000000000711, -24.70250686562997089 ) ) ;
#224221=EDGE_CURVE ( 'NONE', #56815, #4098, #157957, .T. ) ;
#224247=CARTESIAN_POINT ( 'NONE',  ( -20.85000000000000142, -1.164121893241208960, -41.41484808557160591 ) ) ;
#224286=ORIENTED_EDGE ( 'NONE', *, *, #44275, .F. ) ;
#224309=ORIENTED_EDGE ( 'NONE', *, *, #173343, .F. ) ;
#224366=ORIENTED_EDGE ( 'NONE', *, *, #7693, .T. ) ;
#224368=DIRECTION ( 'NONE',  ( 1.000000000000000000, -7.304098846218134667E-16, -4.217023435051625732E-16 ) ) ;
#224379=CARTESIAN_POINT ( 'NONE',  ( 18.49505832270840955, -9.438028062782890970, -7.198473174893858406 ) ) ;
#224402=CIRCLE ( 'NONE', #111994, 0.1000000000000008937 ) ;
#224414=EDGE_CURVE ( 'NONE', #135192, #3158, #112313, .T. ) ;
#224483=CARTESIAN_POINT ( 'NONE',  ( 19.97071067811864609, 11.72071067811865674, -24.75000000000000000 ) ) ;
#224487=CIRCLE ( 'NONE', #20312, 0.1000000000000017958 ) ;
#224524=DIRECTION ( 'NONE',  ( 0.000000000000000000, -0.4930308989875165082, -0.8700118002898358238 ) ) ;
#224530=VERTEX_POINT ( 'NONE', #212465 ) ;
#224533=CYLINDRICAL_SURFACE ( 'NONE', #206470, 4.049999999999998934 ) ;
#224608=CARTESIAN_POINT ( 'NONE',  ( -18.50000000000000000, 7.021664781900089913, -37.33356540189728889 ) ) ;
#224683=CARTESIAN_POINT ( 'NONE',  ( -18.59999999999999787, 11.74999999999999645, 11.75000000000000000 ) ) ;
#224705=ORIENTED_EDGE ( 'NONE', *, *, #8325, .T. ) ;
#224706=VECTOR ( 'NONE', #81398, 1000.000000000000000 ) ;
#224724=CARTESIAN_POINT ( 'NONE',  ( 20.99749315643149217, 11.75000000000000355, -26.48519423124078997 ) ) ;
#224751=AXIS2_PLACEMENT_3D ( 'NONE', #55126, #232544, #53883 ) ;
#224776=CARTESIAN_POINT ( 'NONE',  ( -20.64999999999999858, 1.999999999999998224, -12.72462192276209869 ) ) ;
#224785=CARTESIAN_POINT ( 'NONE',  ( -23.15000000000000213, 0.000000000000000000, -33.50000000000000000 ) ) ;
#224839=AXIS2_PLACEMENT_3D ( 'NONE', #167333, #13378, #231158 ) ;
#224850=DIRECTION ( 'NONE',  ( 1.000000000000000000, -0.000000000000000000, -0.000000000000000000 ) ) ;
#224871=ORIENTED_EDGE ( 'NONE', *, *, #162211, .T. ) ;
#224882=DIRECTION ( 'NONE',  ( -3.265361837132813093E-16, 1.000000000000000000, 0.000000000000000000 ) ) ;
#224893=EDGE_CURVE ( 'NONE', #92153, #33930, #75094, .T. ) ;
#224914=ORIENTED_EDGE ( 'NONE', *, *, #160758, .T. ) ;
#224920=CARTESIAN_POINT ( 'NONE',  ( -23.25000000000000000, 0.000000000000000000, -33.50000000000000000 ) ) ;
#224945=AXIS2_PLACEMENT_3D ( 'NONE', #175622, #196441, #17797 ) ;
#224960=CARTESIAN_POINT ( 'NONE',  ( -20.54999999999999716, 7.150000000000000355, -12.25000000000000000 ) ) ;
#224976=EDGE_LOOP ( 'NONE', ( #216970, #26666, #42520, #132229 ) ) ;
#224983=AXIS2_PLACEMENT_3D ( 'NONE', #22145, #221577, #3844 ) ;
#225012=FACE_OUTER_BOUND ( 'NONE', #184920, .T. ) ;
#225020=SPHERICAL_SURFACE ( 'NONE', #70704, 0.1000000000000000056 ) ;
#225044=CARTESIAN_POINT ( 'NONE',  ( -21.52071067811865746, 7.779289321881349473, -12.34999999999999964 ) ) ;
#225062=DIRECTION ( 'NONE',  ( 0.000000000000000000, 0.000000000000000000, -1.000000000000000000 ) ) ;
#225067=CARTESIAN_POINT ( 'NONE',  ( -20.93284271247462058, 11.74999999999999645, -26.48519422934604961 ) ) ;
#225116=CARTESIAN_POINT ( 'NONE',  ( -18.50000000000000000, 11.65000000000000036, -33.50000000000000000 ) ) ;
#225122=ADVANCED_FACE ( 'NONE', ( #108561 ), #171149, .F. ) ;
#225148=CARTESIAN_POINT ( 'NONE',  ( 18.57071067811864040, 10.17928932188134539, -21.25000000000000000 ) ) ;
#225169=CARTESIAN_POINT ( 'NONE',  ( -21.05000000000000071, 1.360870587192041681, -8.072997927090961312 ) ) ;
#225175=ADVANCED_FACE ( 'NONE', ( #88975 ), #6883, .F. ) ;
#225181=CARTESIAN_POINT ( 'NONE',  ( -21.00219873199058540, 11.60538868787663702, -6.912647428294775409 ) ) ;
#225187=DIRECTION ( 'NONE',  ( 0.000000000000000000, 0.000000000000000000, -1.000000000000000000 ) ) ;
#225190=ORIENTED_EDGE ( 'NONE', *, *, #204204, .F. ) ;
#225227=CARTESIAN_POINT ( 'NONE',  ( 21.14999999999999858, 6.649999999999999467, -12.15000000000000036 ) ) ;
#225235=DIRECTION ( 'NONE',  ( -0.000000000000000000, -0.8700118002898321601, 0.4930308989875230030 ) ) ;
#225259=EDGE_LOOP ( 'NONE', ( #13161, #81719, #254849, #202078 ) ) ;
#225269=CARTESIAN_POINT ( 'NONE',  ( -20.64999999999999858, 7.249999999999999112, -12.25000000000000000 ) ) ;
#225292=AXIS2_PLACEMENT_3D ( 'NONE', #255811, #194634, #236290 ) ;
#225295=DIRECTION ( 'NONE',  ( 1.000000000000000000, 1.836970198721029934E-16, 0.000000000000000000 ) ) ;
#225307=LINE ( 'NONE', #165367, #114972 ) ;
#225312=DIRECTION ( 'NONE',  ( -0.000000000000000000, 0.8660254037844411501, 0.4999999999999956146 ) ) ;
#225322=DIRECTION ( 'NONE',  ( 0.000000000000000000, 0.000000000000000000, -1.000000000000000000 ) ) ;
#225326=CARTESIAN_POINT ( 'NONE',  ( 21.05000000000000071, -8.663551401869158397, -9.524101118067305194 ) ) ;
#225340=AXIS2_PLACEMENT_3D ( 'NONE', #142645, #222174, #66982 ) ;
#225352=CARTESIAN_POINT ( 'NONE',  ( -18.59999999999999787, -1.835859311443637010, -45.00443916879852679 ) ) ;
#225383=LINE ( 'NONE', #247538, #152299 ) ;
#225386=AXIS2_PLACEMENT_3D ( 'NONE', #59235, #38437, #214498 ) ;
#225388=DIRECTION ( 'NONE',  ( 0.000000000000000000, -0.8660254037844412611, -0.4999999999999956701 ) ) ;
#225402=CARTESIAN_POINT ( 'NONE',  ( 20.94999999999999929, 8.776282895292474961, -21.25000000000000000 ) ) ;
#225411=DIRECTION ( 'NONE',  ( -0.000000000000000000, 0.000000000000000000, 1.000000000000000000 ) ) ;
#225478=ORIENTED_EDGE ( 'NONE', *, *, #30824, .T. ) ;
#225504=EDGE_LOOP ( 'NONE', ( #45814, #105, #66379, #185451 ) ) ;
#225538=VERTEX_POINT ( 'NONE', #84803 ) ;
#225541=EDGE_CURVE ( 'NONE', #250767, #243771, #133505, .T. ) ;
#225606=CARTESIAN_POINT ( 'NONE',  ( -22.59999999999999787, 11.64957080754479968, 0.09999999999999592548 ) ) ;
#225617=CARTESIAN_POINT ( 'NONE',  ( 22.39999999999999858, 0.09999999999999939493, 7.790779598373383408 ) ) ;
#225636=ADVANCED_FACE ( 'NONE', ( #206077 ), #49568, .T. ) ;
#225651=DIRECTION ( 'NONE',  ( -1.000000000000000000, -0.000000000000000000, -0.000000000000000000 ) ) ;
#225666=VERTEX_POINT ( 'NONE', #96374 ) ;
#225677=FACE_OUTER_BOUND ( 'NONE', #248757, .T. ) ;
#225685=CARTESIAN_POINT ( 'NONE',  ( 23.14999999999999503, 11.75000000000000711, -21.35000000000000142 ) ) ;
#225755=AXIS2_PLACEMENT_3D ( 'NONE', #145818, #205802, #144533 ) ;
#225790=CIRCLE ( 'NONE', #167576, 0.5000000000000013323 ) ;
#225795=EDGE_CURVE ( 'NONE', #127472, #251836, #98930, .T. ) ;
#225817=LINE ( 'NONE', #4217, #196343 ) ;
#225852=CARTESIAN_POINT ( 'NONE',  ( 20.85000000000000142, -11.64999999999999147, -33.50000000000000000 ) ) ;
#225858=EDGE_CURVE ( 'NONE', #28028, #233325, #141932, .T. ) ;
#225869=DIRECTION ( 'NONE',  ( 0.000000000000000000, 0.000000000000000000, -1.000000000000000000 ) ) ;
#225896=ORIENTED_EDGE ( 'NONE', *, *, #124201, .T. ) ;
#225897=TOROIDAL_SURFACE ( 'NONE', #13560, 0.2000000000000000111, 0.1000000000000000056 ) ;
#225905=DIRECTION ( 'NONE',  ( 0.000000000000000000, 0.6728971962616783209, 0.7397360091702797069 ) ) ;
#225921=ORIENTED_EDGE ( 'NONE', *, *, #85576, .T. ) ;
#225922=ORIENTED_EDGE ( 'NONE', *, *, #146143, .T. ) ;
#225929=ADVANCED_FACE ( 'NONE', ( #165360 ), #105339, .T. ) ;
#225952=DIRECTION ( 'NONE',  ( 0.000000000000000000, 0.000000000000000000, -1.000000000000000000 ) ) ;
#225957=CARTESIAN_POINT ( 'NONE',  ( 20.94999999999999929, -9.000000000000001776, -9.893969122652443104 ) ) ;
#225973=ORIENTED_EDGE ( 'NONE', *, *, #67837, .F. ) ;
#225979=FACE_OUTER_BOUND ( 'NONE', #183173, .T. ) ;
#226040=DIRECTION ( 'NONE',  ( -1.000000000000000000, 7.304098846218133681E-16, -4.217023435051677994E-16 ) ) ;
#226043=ADVANCED_FACE ( 'NONE', ( #248752 ), #47964, .F. ) ;
#226056=CYLINDRICAL_SURFACE ( 'NONE', #221390, 0.09999999999999939493 ) ;
#226061=ADVANCED_FACE ( 'NONE', ( #92225 ), #39480, .F. ) ;
#226088=EDGE_CURVE ( 'NONE', #79663, #235074, #149667, .T. ) ;
#226110=CARTESIAN_POINT ( 'NONE',  ( 18.49999999999998934, 10.29288807858825905, -38.95800201601215917 ) ) ;
#226142=EDGE_CURVE ( 'NONE', #73461, #117400, #72118, .T. ) ;
#226150=VERTEX_POINT ( 'NONE', #175640 ) ;
#226152=ORIENTED_EDGE ( 'NONE', *, *, #176869, .F. ) ;
#226186=DIRECTION ( 'NONE',  ( 0.000000000000000000, 0.000000000000000000, -1.000000000000000000 ) ) ;
#226210=CARTESIAN_POINT ( 'NONE',  ( -20.85000000000000142, -1.835859311443637010, -45.10443916879852821 ) ) ;
#226218=AXIS2_PLACEMENT_3D ( 'NONE', #159538, #156983, #56539 ) ;
#226258=FACE_OUTER_BOUND ( 'NONE', #37207, .T. ) ;
#226278=ORIENTED_EDGE ( 'NONE', *, *, #63806, .F. ) ;
#226282=CARTESIAN_POINT ( 'NONE',  ( 20.94999999999999929, 7.021664781900089913, -37.33356540189728889 ) ) ;
#226285=VERTEX_POINT ( 'NONE', #29425 ) ;
#226291=VECTOR ( 'NONE', #84057, 1000.000000000000000 ) ;
#226295=CARTESIAN_POINT ( 'NONE',  ( -21.14999999999999858, 11.75000000000000000, -0.1000000000000028644 ) ) ;
#226310=CARTESIAN_POINT ( 'NONE',  ( 22.39999999999999503, 7.790779598373379855, 0.09999999999999939493 ) ) ;
#226383=DIRECTION ( 'NONE',  ( 0.000000000000000000, -0.9999631594459056361, -0.008583690987124413183 ) ) ;
#226428=ORIENTED_EDGE ( 'NONE', *, *, #117039, .T. ) ;
#226429=ORIENTED_EDGE ( 'NONE', *, *, #251071, .F. ) ;
#226449=DIRECTION ( 'NONE',  ( 0.000000000000000000, 1.000000000000000000, 0.000000000000000000 ) ) ;
#226476=ORIENTED_EDGE ( 'NONE', *, *, #3514, .T. ) ;
#226479=DIRECTION ( 'NONE',  ( -0.7071067811865388020, 0.7071067811865561215, 0.000000000000000000 ) ) ;
#226488=FACE_OUTER_BOUND ( 'NONE', #210912, .T. ) ;
#226493=ORIENTED_EDGE ( 'NONE', *, *, #59914, .F. ) ;
#226507=ORIENTED_EDGE ( 'NONE', *, *, #12603, .F. ) ;
#226533=DIRECTION ( 'NONE',  ( 3.265361837132813093E-16, -1.000000000000000000, -0.000000000000000000 ) ) ;
#226537=AXIS2_PLACEMENT_3D ( 'NONE', #197980, #221380, #42768 ) ;
#226555=ADVANCED_FACE ( 'NONE', ( #132331 ), #211894, .T. ) ;
#226600=VERTEX_POINT ( 'NONE', #257354 ) ;
#226648=DIRECTION ( 'NONE',  ( 1.000000000000000000, -0.000000000000000000, -0.000000000000000000 ) ) ;
#226656=CIRCLE ( 'NONE', #114230, 0.1000000000000000472 ) ;
#226663=ORIENTED_EDGE ( 'NONE', *, *, #247474, .T. ) ;
#226696=DIRECTION ( 'NONE',  ( 1.000000000000000000, 0.000000000000000000, -0.000000000000000000 ) ) ;
#226727=ADVANCED_FACE ( 'NONE', ( #184293 ), #124339, .F. ) ;
#226737=EDGE_CURVE ( 'NONE', #3158, #250243, #209855, .T. ) ;
#226741=CIRCLE ( 'NONE', #230871, 0.09999999999999939493 ) ;
#226759=CARTESIAN_POINT ( 'NONE',  ( 21.14999999999999858, 6.540656951701244282, 0.000000000000000000 ) ) ;
#226810=VERTEX_POINT ( 'NONE', #216568 ) ;
#226854=CARTESIAN_POINT ( 'NONE',  ( -21.07928932188134041, 6.328516656393293083, 0.09889514565439641580 ) ) ;
#226880=EDGE_CURVE ( 'NONE', #133463, #77132, #164055, .T. ) ;
#226885=VECTOR ( 'NONE', #7482, 1000.000000000000000 ) ;
#226895=DIRECTION ( 'NONE',  ( 0.000000000000000000, 0.9998779222360096863, -0.01562500000001061998 ) ) ;
#226931=DIRECTION ( 'NONE',  ( 0.000000000000000000, -0.9999176327611369874, 0.01283462868041987913 ) ) ;
#226958=CARTESIAN_POINT ( 'NONE',  ( -23.25000000000000000, 4.349999999999999645, -12.35000000000000142 ) ) ;
#226990=CARTESIAN_POINT ( 'NONE',  ( -23.25000000000000000, -1.835859311443637010, -45.10443916879852821 ) ) ;
#226999=ORIENTED_EDGE ( 'NONE', *, *, #237805, .F. ) ;
#227021=CARTESIAN_POINT ( 'NONE',  ( -21.05000000000000071, 0.2561057920922211739, 0.03489644167229202787 ) ) ;
#227082=CARTESIAN_POINT ( 'NONE',  ( 21.13498764882293557, 6.495618143473869566, 0.001656394731334435771 ) ) ;
#227111=CARTESIAN_POINT ( 'NONE',  ( -20.94999999999999929, -1.835341550224413698, -11.55515129256298223 ) ) ;
#227113=VERTEX_POINT ( 'NONE', #115539 ) ;
#227131=CARTESIAN_POINT ( 'NONE',  ( 18.59999999999997655, 0.000000000000000000, -33.50000000000000000 ) ) ;
#227151=EDGE_CURVE ( 'NONE', #33602, #97347, #155881, .T. ) ;
#227165=VERTEX_POINT ( 'NONE', #77680 ) ;
#227202=ORIENTED_EDGE ( 'NONE', *, *, #92749, .T. ) ;
#227236=VERTEX_POINT ( 'NONE', #115873 ) ;
#227241=CARTESIAN_POINT ( 'NONE',  ( 21.05000000000000071, 6.257814610476124528, 0.09779029130879343668 ) ) ;
#227244=DIRECTION ( 'NONE',  ( 0.000000000000000000, 0.000000000000000000, 1.000000000000000000 ) ) ;
#227264=DIRECTION ( 'NONE',  ( 0.000000000000000000, 1.000000000000000000, 0.000000000000000000 ) ) ;
#227272=CIRCLE ( 'NONE', #48206, 0.09999999999999939493 ) ;
#227301=CARTESIAN_POINT ( 'NONE',  ( 21.05000000000000071, 11.75000000000000355, -26.48519422934606027 ) ) ;
#227304=ORIENTED_EDGE ( 'NONE', *, *, #142740, .T. ) ;
#227311=ORIENTED_EDGE ( 'NONE', *, *, #61107, .T. ) ;
#227317=LINE ( 'NONE', #52522, #184424 ) ;
#227363=AXIS2_PLACEMENT_3D ( 'NONE', #225227, #144403, #81852 ) ;
#227366=DIRECTION ( 'NONE',  ( 0.000000000000000000, 0.000000000000000000, 1.000000000000000000 ) ) ;
#227371=ADVANCED_FACE ( 'NONE', ( #226488 ), #127418, .T. ) ;
#227384=CARTESIAN_POINT ( 'NONE',  ( 21.05000000000000071, 11.65000000000000391, -0.1000000000000028644 ) ) ;
#227385=DIRECTION ( 'NONE',  ( 0.000000000000000000, 0.000000000000000000, -1.000000000000000000 ) ) ;
#227396=DIRECTION ( 'NONE',  ( 0.000000000000000000, 0.4999999999999956701, -0.8660254037844411501 ) ) ;
#227408=EDGE_CURVE ( 'NONE', #218249, #233645, #62310, .T. ) ;
#227426=DIRECTION ( 'NONE',  ( 0.000000000000000000, 0.000000000000000000, -1.000000000000000000 ) ) ;
#227429=CARTESIAN_POINT ( 'NONE',  ( 18.49999999999999289, 10.20857864376269575, -21.35000000000000142 ) ) ;
#227574=AXIS2_PLACEMENT_3D ( 'NONE', #35827, #154509, #14979 ) ;
#227603=CARTESIAN_POINT ( 'NONE',  ( 20.94999999999999574, -11.64999999999999147, -2.900000000000003464 ) ) ;
#227672=PLANE ( 'NONE',  #195391 ) ;
#227681=CARTESIAN_POINT ( 'NONE',  ( -22.49806830649814415, 11.64988965483908068, 0.07746431632550303259 ) ) ;
#227688=DIRECTION ( 'NONE',  ( 0.000000000000000000, 0.000000000000000000, -1.000000000000000000 ) ) ;
#227717=EDGE_CURVE ( 'NONE', #115921, #105026, #181187, .T. ) ;
#227813=CYLINDRICAL_SURFACE ( 'NONE', #231848, 0.1000000000000000472 ) ;
#227836=CARTESIAN_POINT ( 'NONE',  ( -18.39999999999999858, -9.500000000000005329, -40.10018939122204529 ) ) ;
#227839=CARTESIAN_POINT ( 'NONE',  ( 18.59999999999999076, 6.550000000000000711, -21.25000000000000000 ) ) ;
#227853=DIRECTION ( 'NONE',  ( 0.000000000000000000, 0.000000000000000000, -1.000000000000000000 ) ) ;
#227897=DIRECTION ( 'NONE',  ( 0.000000000000000000, 1.000000000000000000, 0.000000000000000000 ) ) ;
#227902=EDGE_CURVE ( 'NONE', #191690, #132561, #198633, .T. ) ;
#227924=CARTESIAN_POINT ( 'NONE',  ( 21.05543885634738643, 8.775771046847536283, -12.18438447071468822 ) ) ;
#227942=CARTESIAN_POINT ( 'NONE',  ( 23.14999999999999858, 6.649999999999999467, -12.35000000000000320 ) ) ;
#227954=DIRECTION ( 'NONE',  ( 0.000000000000000000, 0.000000000000000000, -1.000000000000000000 ) ) ;
#227984=DIRECTION ( 'NONE',  ( 0.000000000000000000, 1.776356839400250465E-15, 1.000000000000000000 ) ) ;
#228001=VERTEX_POINT ( 'NONE', #139928 ) ;
#228021=CARTESIAN_POINT ( 'NONE',  ( -18.59999994787167310, -9.523637689761692116, -40.38244953477238397 ) ) ;
#228124=CARTESIAN_POINT ( 'NONE',  ( -23.15000000000000213, 11.65000000000000036, -26.48519422934605316 ) ) ;
#228125=PLANE ( 'NONE',  #197368 ) ;
#228180=ORIENTED_EDGE ( 'NONE', *, *, #6892, .T. ) ;
#228185=VECTOR ( 'NONE', #95671, 999.9999999999998863 ) ;
#228195=ORIENTED_EDGE ( 'NONE', *, *, #77184, .T. ) ;
#228206=DIRECTION ( 'NONE',  ( 1.000000000000000000, 0.000000000000000000, 0.000000000000000000 ) ) ;
#228243=AXIS2_PLACEMENT_3D ( 'NONE', #121965, #99798, #179387 ) ;
#228269=CIRCLE ( 'NONE', #136651, 0.1000000000000028644 ) ;
#228272=CARTESIAN_POINT ( 'NONE',  ( 18.59999999999999432, 1.162701749938009677, -8.099999999999999645 ) ) ;
#228279=ORIENTED_EDGE ( 'NONE', *, *, #39113, .F. ) ;
#228282=AXIS2_PLACEMENT_3D ( 'NONE', #203825, #22649, #102126 ) ;
#228288=DIRECTION ( 'NONE',  ( 0.000000000000000000, 0.000000000000000000, -1.000000000000000000 ) ) ;
#228291=EDGE_LOOP ( 'NONE', ( #36722, #201598, #23324, #145810 ) ) ;
#228294=CARTESIAN_POINT ( 'NONE',  ( -20.54999999999999716, 7.150000000000000355, -12.34999999999999964 ) ) ;
#228353=CIRCLE ( 'NONE', #74255, 0.1000000000000000472 ) ;
#228372=AXIS2_PLACEMENT_3D ( 'NONE', #125215, #123940, #86045 ) ;
#228378=ORIENTED_EDGE ( 'NONE', *, *, #157854, .F. ) ;
#228389=ORIENTED_EDGE ( 'NONE', *, *, #199870, .T. ) ;
#228414=AXIS2_PLACEMENT_3D ( 'NONE', #45862, #142392, #220659 ) ;
#228418=DIRECTION ( 'NONE',  ( 1.000000000000000000, -0.000000000000000000, 0.000000000000000000 ) ) ;
#228446=SPHERICAL_SURFACE ( 'NONE', #205897, 0.1000000000000000056 ) ;
#228452=VECTOR ( 'NONE', #253573, 1000.000000000000000 ) ;
#228469=CARTESIAN_POINT ( 'NONE',  ( -18.59999999999999787, 7.021664781900089913, -37.33356540189728889 ) ) ;
#228482=EDGE_LOOP ( 'NONE', ( #251641, #148682, #38744, #102165 ) ) ;
#228494=CARTESIAN_POINT ( 'NONE',  ( 18.59999999999999076, 6.450000000000001066, -10.01702717044002000 ) ) ;
#228551=FACE_OUTER_BOUND ( 'NONE', #118787, .T. ) ;
#228563=AXIS2_PLACEMENT_3D ( 'NONE', #66246, #205741, #28440 ) ;
#228573=CARTESIAN_POINT ( 'NONE',  ( 18.49999999999999645, 0.000000000000000000, -33.50000000000000000 ) ) ;
#228578=CARTESIAN_POINT ( 'NONE',  ( -21.05000000000000071, 0.000000000000000000, 0.000000000000000000 ) ) ;
#228580=ORIENTED_EDGE ( 'NONE', *, *, #204204, .T. ) ;
#228710=ADVANCED_FACE ( 'NONE', ( #218515 ), #255031, .F. ) ;
#228762=CYLINDRICAL_SURFACE ( 'NONE', #159654, 0.09999999999999939493 ) ;
#228772=ORIENTED_EDGE ( 'NONE', *, *, #65496, .F. ) ;
#228785=CIRCLE ( 'NONE', #116365, 0.09999999999999939493 ) ;
#228788=ORIENTED_EDGE ( 'NONE', *, *, #77368, .T. ) ;
#228825=DIRECTION ( 'NONE',  ( 0.000000000000000000, -0.000000000000000000, 1.000000000000000000 ) ) ;
#228826=ORIENTED_EDGE ( 'NONE', *, *, #160593, .F. ) ;
#228855=CARTESIAN_POINT ( 'NONE',  ( -18.59999999999999787, 11.64999999999999680, -7.014805770654001016 ) ) ;
#228862=CARTESIAN_POINT ( 'NONE',  ( -22.39999999999999858, 0.09999999999999939493, 7.790779598373403836 ) ) ;
#228884=AXIS2_PLACEMENT_3D ( 'NONE', #53164, #234360, #91008 ) ;
#228885=EDGE_LOOP ( 'NONE', ( #133137, #200480, #119644, #213916 ) ) ;
#228889=EDGE_CURVE ( 'NONE', #185054, #117327, #6747, .T. ) ;
#228909=DIRECTION ( 'NONE',  ( -1.000000000000000000, -0.000000000000000000, -0.000000000000000000 ) ) ;
#228936=CARTESIAN_POINT ( 'NONE',  ( 20.93302460841142931, 10.31565961586829872, -39.03641941191782649 ) ) ;
#229006=ADVANCED_FACE ( 'NONE', ( #76149 ), #456, .T. ) ;
#229025=EDGE_CURVE ( 'NONE', #107696, #137697, #148594, .T. ) ;
#229056=VECTOR ( 'NONE', #103443, 1000.000000000000000 ) ;
#229057=CYLINDRICAL_SURFACE ( 'NONE', #102159, 0.09999999999999939493 ) ;
#229064=DIRECTION ( 'NONE',  ( 0.000000000000000000, 0.000000000000000000, 1.000000000000000000 ) ) ;
#229100=DIRECTION ( 'NONE',  ( 0.000000000000000000, 1.000000000000000000, 0.000000000000000000 ) ) ;
#229108=FACE_OUTER_BOUND ( 'NONE', #223867, .T. ) ;
#229124=ORIENTED_EDGE ( 'NONE', *, *, #5388, .F. ) ;
#229146=EDGE_CURVE ( 'NONE', #83974, #143516, #102753, .T. ) ;
#229184=DIRECTION ( 'NONE',  ( -7.304098846218134667E-16, 1.000000000000000000, -0.000000000000000000 ) ) ;
#229202=AXIS2_PLACEMENT_3D ( 'NONE', #129405, #86391, #31624 ) ;
#229249=DIRECTION ( 'NONE',  ( 0.000000000000000000, 0.9908441862701596881, 0.1350103645451904977 ) ) ;
#229268=ORIENTED_EDGE ( 'NONE', *, *, #20235, .F. ) ;
#229285=VECTOR ( 'NONE', #20483, 1000.000000000000000 ) ;
#229287=DIRECTION ( 'NONE',  ( -2.952720810173288619E-16, 1.000000000000000000, 0.000000000000000000 ) ) ;
#229293=ADVANCED_FACE ( 'NONE', ( #31631 ), #156981, .F. ) ;
#229313=CARTESIAN_POINT ( 'NONE',  ( -18.54260524012581612, -9.624219390073767144, -40.24077304577079417 ) ) ;
#229343=DIRECTION ( 'NONE',  ( 0.000000000000000000, 0.000000000000000000, 1.000000000000000000 ) ) ;
#229344=ADVANCED_FACE ( 'NONE', ( #87697 ), #57152, .F. ) ;
#229360=FACE_OUTER_BOUND ( 'NONE', #29089, .T. ) ;
#229377=CARTESIAN_POINT ( 'NONE',  ( 18.50000000000000355, -9.480686695278970788, -40.44111516875785384 ) ) ;
#229435=AXIS2_PLACEMENT_3D ( 'NONE', #41673, #101587, #102883 ) ;
#229436=EDGE_CURVE ( 'NONE', #210699, #172995, #152896, .T. ) ;
#229460=EDGE_CURVE ( 'NONE', #250767, #216880, #256857, .T. ) ;
#229518=ORIENTED_EDGE ( 'NONE', *, *, #93584, .F. ) ;
#229519=EDGE_LOOP ( 'NONE', ( #41358, #31409, #86461, #160354 ) ) ;
#229522=CARTESIAN_POINT ( 'NONE',  ( -18.50000000000000711, 11.64999999999999680, -7.014805770653998351 ) ) ;
#229525=EDGE_CURVE ( 'NONE', #53632, #176194, #212815, .T. ) ;
#229532=CARTESIAN_POINT ( 'NONE',  ( -21.04999999999999716, 0.01485563489362509877, 6.344359042043403285 ) ) ;
#229541=ORIENTED_EDGE ( 'NONE', *, *, #1416, .F. ) ;
#229549=CARTESIAN_POINT ( 'NONE',  ( -21.09107601085575112, 6.363877975359904404, 0.03930716471739981871 ) ) ;
#229559=DIRECTION ( 'NONE',  ( 1.000000000000000000, 0.000000000000000000, 0.000000000000000000 ) ) ;
#229574=CIRCLE ( 'NONE', #187884, 0.09999999999999939493 ) ;
#229578=LINE ( 'NONE', #50898, #190560 ) ;
#229603=DIRECTION ( 'NONE',  ( -0.000000000000000000, 1.000000000000000000, -0.000000000000000000 ) ) ;
#229636=ORIENTED_EDGE ( 'NONE', *, *, #232700, .T. ) ;
#229646=AXIS2_PLACEMENT_3D ( 'NONE', #97197, #95949, #158531 ) ;
#229696=CIRCLE ( 'NONE', #67369, 3.999999999999996447 ) ;
#229721=AXIS2_PLACEMENT_3D ( 'NONE', #147979, #149283, #112705 ) ;
#229742=DIRECTION ( 'NONE',  ( -2.940209281316621509E-16, 1.000000000000000000, 0.000000000000000000 ) ) ;
#229800=EDGE_CURVE ( 'NONE', #86957, #112457, #252992, .T. ) ;
#229831=EDGE_LOOP ( 'NONE', ( #177036, #41765, #25328, #50557 ) ) ;
#229877=CARTESIAN_POINT ( 'NONE',  ( 23.14999999999999858, 11.60000000000000675, -26.57179676972450011 ) ) ;
#229881=CARTESIAN_POINT ( 'NONE',  ( 21.02374657821574644, 11.60000000082048643, -26.57179677019820829 ) ) ;
#229913=AXIS2_PLACEMENT_3D ( 'NONE', #96469, #232172, #54786 ) ;
#229935=LINE ( 'NONE', #192114, #55267 ) ;
#229966=DIRECTION ( 'NONE',  ( 0.000000000000000000, 1.000000000000000000, 0.000000000000000000 ) ) ;
#229967=ORIENTED_EDGE ( 'NONE', *, *, #72597, .F. ) ;
#229994=AXIS2_PLACEMENT_3D ( 'NONE', #89922, #189041, #169519 ) ;
#229997=CARTESIAN_POINT ( 'NONE',  ( -20.94999999999999929, -11.75000000000000000, -30.39999999999999503 ) ) ;
#230001=VECTOR ( 'NONE', #177304, 1000.000000000000000 ) ;
#230019=LINE ( 'NONE', #189623, #111693 ) ;
#230051=CIRCLE ( 'NONE', #84244, 0.2000000000000005107 ) ;
#230065=DIRECTION ( 'NONE',  ( 0.000000000000000000, -1.000000000000000000, -0.000000000000000000 ) ) ;
#230112=EDGE_CURVE ( 'NONE', #141594, #15975, #6903, .T. ) ;
#230113=CARTESIAN_POINT ( 'NONE',  ( 18.59999999999999076, 11.75000000000000355, 11.75000000000000000 ) ) ;
#230123=EDGE_CURVE ( 'NONE', #117566, #9216, #253169, .T. ) ;
#230131=ORIENTED_EDGE ( 'NONE', *, *, #252847, .F. ) ;
#230140=DIRECTION ( 'NONE',  ( 0.000000000000000000, -1.000000000000000000, 0.000000000000000000 ) ) ;
#230171=AXIS2_PLACEMENT_3D ( 'NONE', #214382, #194848, #252211 ) ;
#230181=EDGE_CURVE ( 'NONE', #62691, #11112, #233983, .T. ) ;
#230207=EDGE_CURVE ( 'NONE', #176194, #95630, #244786, .T. ) ;
#230209=CARTESIAN_POINT ( 'NONE',  ( 20.94999999999999929, 10.29270135740183179, -38.95736188715193293 ) ) ;
#230218=DIRECTION ( 'NONE',  ( 0.9880948137434723000, 0.1538461538461484146, -0.000000000000000000 ) ) ;
#230251=DIRECTION ( 'NONE',  ( -1.000000000000000000, -0.000000000000000000, -0.000000000000000000 ) ) ;
#230252=DIRECTION ( 'NONE',  ( 0.000000000000000000, 1.000000000000000000, 0.000000000000000000 ) ) ;
#230261=B_SPLINE_CURVE_WITH_KNOTS ( 'NONE', 3,
 ( #5631, #223407, #143874, #222110, #162192, #64359, #202579, #145152, #100857, #181736, #1789, #245567, #183030, #106017, #241705, #240422, #142582, #43512, #104720 ),
 .UNSPECIFIED., .F., .F.,
 ( 4, 3, 3, 3, 3, 3, 4 ),
 ( 0.000000000000000000, 2.646747978908405163E-05, 5.271166642128515082E-05, 9.008788829884125608E-05, 0.0001426648776560996530, 0.0001897378458659833658, 0.0001917382627806356570 ),
 .UNSPECIFIED. ) ;
#230264=ORIENTED_EDGE ( 'NONE', *, *, #203463, .T. ) ;
#230284=DIRECTION ( 'NONE',  ( 1.000000000000000000, 0.000000000000000000, 0.000000000000000000 ) ) ;
#230288=VERTEX_POINT ( 'NONE', #115320 ) ;
#230291=DIRECTION ( 'NONE',  ( 1.000000000000000000, 0.000000000000000000, 0.000000000000000000 ) ) ;
#230321=FACE_OUTER_BOUND ( 'NONE', #32462, .T. ) ;
#230347=ORIENTED_EDGE ( 'NONE', *, *, #66730, .F. ) ;
#230348=ORIENTED_EDGE ( 'NONE', *, *, #151561, .F. ) ;
#230451=PLANE ( 'NONE',  #103438 ) ;
#230458=VECTOR ( 'NONE', #240298, 1000.000000000000114 ) ;
#230464=EDGE_CURVE ( 'NONE', #167773, #183080, #206825, .T. ) ;
#230467=ORIENTED_EDGE ( 'NONE', *, *, #130993, .T. ) ;
#230470=ORIENTED_EDGE ( 'NONE', *, *, #245411, .T. ) ;
#230476=DIRECTION ( 'NONE',  ( 0.000000000000000000, -0.4999999999999929501, 0.8660254037844427044 ) ) ;
#230477=VERTEX_POINT ( 'NONE', #126891 ) ;
#230484=ORIENTED_EDGE ( 'NONE', *, *, #142962, .F. ) ;
#230498=ORIENTED_EDGE ( 'NONE', *, *, #1477, .F. ) ;
#230519=CARTESIAN_POINT ( 'NONE',  ( 23.14999999999999858, 4.775700934579435675, -21.65123189595403375 ) ) ;
#230582=AXIS2_PLACEMENT_3D ( 'NONE', #49639, #50895, #127903 ) ;
#230596=CARTESIAN_POINT ( 'NONE',  ( -18.31572283045144900, -9.548437830885816879, -40.35062565105839383 ) ) ;
#230597=VECTOR ( 'NONE', #193546, 1000.000000000000000 ) ;
#230606=ORIENTED_EDGE ( 'NONE', *, *, #201112, .F. ) ;
#230619=( BOUNDED_SURFACE ( )  B_SPLINE_SURFACE ( 3, 2, ( 
 ( #161291, #240814, #216096 ),
 ( #62179, #42605, #122150 ),
 ( #17895, #97407, #77868 ),
 ( #58296, #178296, #10868 ) ),
 .UNSPECIFIED., .F., .F., .F. ) 
 B_SPLINE_SURFACE_WITH_KNOTS ( ( 4, 4 ),
 ( 3, 3 ),
 ( -1.355252715606880543E-20, 0.0003124336117481267463 ),
 ( 0.000000000000000000, 1.000000000000000000 ),
 .UNSPECIFIED. ) 
 GEOMETRIC_REPRESENTATION_ITEM ( )  RATIONAL_B_SPLINE_SURFACE ( (
 ( 1.000000000000000000, 0.7040654476015973939, 1.000000000000000000),
 ( 1.000000000000000000, 0.7039193538781929327, 1.000000000000000000),
 ( 1.000000000000000000, 0.7089171279145388693, 1.000000000000000000),
 ( 1.000000000000000000, 0.7071067811865567876, 1.000000000000000000) ) ) 
 REPRESENTATION_ITEM ( '' )  SURFACE ( )  );
#230626=DIRECTION ( 'NONE',  ( 1.000000000000000000, 0.000000000000000000, 0.000000000000000000 ) ) ;
#230658=CARTESIAN_POINT ( 'NONE',  ( 18.31572054635735114, -9.548475435778739140, -40.35057016474856795 ) ) ;
#230676=LINE ( 'NONE', #231969, #104 ) ;
#230689=DIRECTION ( 'NONE',  ( -0.000000000000000000, -0.000000000000000000, 1.000000000000000000 ) ) ;
#230692=DIRECTION ( 'NONE',  ( 0.000000000000000000, 1.000000000000000000, 0.000000000000000000 ) ) ;
#230711=AXIS2_PLACEMENT_3D ( 'NONE', #87567, #103273, #224524 ) ;
#230729=AXIS2_PLACEMENT_3D ( 'NONE', #198214, #159124, #216496 ) ;
#230759=LINE ( 'NONE', #93785, #194440 ) ;
#230763=EDGE_LOOP ( 'NONE', ( #153187, #163531, #176304, #73839, #40564, #119880, #99700, #38168 ) ) ;
#230789=EDGE_CURVE ( 'NONE', #120448, #62457, #23695, .T. ) ;
#230808=DIRECTION ( 'NONE',  ( 0.000000000000000000, -1.000000000000000000, -2.891205793294679805E-16 ) ) ;
#230827=EDGE_CURVE ( 'NONE', #242875, #108030, #123624, .T. ) ;
#230870=CARTESIAN_POINT ( 'NONE',  ( -20.94999999999999929, 1.249999999999999334, -8.000000000000000000 ) ) ;
#230871=AXIS2_PLACEMENT_3D ( 'NONE', #110378, #101032, #80205 ) ;
#230905=EDGE_CURVE ( 'NONE', #31765, #219381, #2980, .T. ) ;
#230939=FACE_OUTER_BOUND ( 'NONE', #115305, .T. ) ;
#230971=DIRECTION ( 'NONE',  ( -2.827886303505248766E-16, 0.8660254037844411501, 0.4999999999999956146 ) ) ;
#231019=AXIS2_PLACEMENT_3D ( 'NONE', #111345, #112628, #94330 ) ;
#231028=CARTESIAN_POINT ( 'NONE',  ( 21.14999999999999858, 11.65000000000000391, -12.15000000000000036 ) ) ;
#231108=AXIS2_PLACEMENT_3D ( 'NONE', #188931, #89811, #168130 ) ;
#231115=ORIENTED_EDGE ( 'NONE', *, *, #14804, .F. ) ;
#231158=DIRECTION ( 'NONE',  ( 0.000000000000000000, 0.000000000000000000, -1.000000000000000000 ) ) ;
#231159=EDGE_CURVE ( 'NONE', #6293, #115921, #173920, .T. ) ;
#231168=CARTESIAN_POINT ( 'NONE',  ( 20.94999999999999929, 4.999999999999997335, -21.49473398108690603 ) ) ;
#231196=ORIENTED_EDGE ( 'NONE', *, *, #151246, .F. ) ;
#231207=EDGE_CURVE ( 'NONE', #250275, #256624, #140535, .T. ) ;
#231209=AXIS2_PLACEMENT_3D ( 'NONE', #204077, #221069, #198943 ) ;
#231246=EDGE_CURVE ( 'NONE', #4508, #141594, #157144, .T. ) ;
#231299=DIRECTION ( 'NONE',  ( -3.265361837132813093E-16, 1.000000000000000000, 0.000000000000000000 ) ) ;
#231324=ORIENTED_EDGE ( 'NONE', *, *, #154764, .F. ) ;
#231405=DIRECTION ( 'NONE',  ( 0.000000000000000000, 0.000000000000000000, -1.000000000000000000 ) ) ;
#231422=FACE_OUTER_BOUND ( 'NONE', #103759, .T. ) ;
#231458=CARTESIAN_POINT ( 'NONE',  ( -22.50000000000000000, 11.64999999999997549, -3.469446951953614189E-15 ) ) ;
#231471=VECTOR ( 'NONE', #49181, 1000.000000000000000 ) ;
#231477=EDGE_CURVE ( 'NONE', #255460, #81419, #242293, .T. ) ;
#231484=VECTOR ( 'NONE', #74620, 1000.000000000000000 ) ;
#231495=EDGE_LOOP ( 'NONE', ( #243848, #121554, #256780, #19693 ) ) ;
#231506=CARTESIAN_POINT ( 'NONE',  ( 23.24999999999999645, 4.999999999999997335, -21.09473398108690390 ) ) ;
#231521=CARTESIAN_POINT ( 'NONE',  ( 20.95512828230152280, 8.876151312325294640, -12.20243026550310361 ) ) ;
#231522=CARTESIAN_POINT ( 'NONE',  ( -20.05000000000000426, 9.250000000000001776, -12.34999999999999964 ) ) ;
#231535=EDGE_LOOP ( 'NONE', ( #190304, #198076, #2106, #209124 ) ) ;
#231543=DIRECTION ( 'NONE',  ( -0.000000000000000000, -0.000000000000000000, 1.000000000000000000 ) ) ;
#231553=CARTESIAN_POINT ( 'NONE',  ( 21.05000000000000071, 10.68429367438713484, -7.526673938637355121 ) ) ;
#231572=CARTESIAN_POINT ( 'NONE',  ( 20.94999999999999574, 5.899999999999947065, -10.21909976465641456 ) ) ;
#231589=LINE ( 'NONE', #95904, #196102 ) ;
#231602=CARTESIAN_POINT ( 'NONE',  ( 18.49999999999999289, 7.120270961697594103, -37.15956304183931991 ) ) ;
#231622=FACE_OUTER_BOUND ( 'NONE', #110397, .T. ) ;
#231642=AXIS2_PLACEMENT_3D ( 'NONE', #161731, #83417, #245092 ) ;
#231645=VECTOR ( 'NONE', #206957, 1000.000000000000000 ) ;
#231650=LINE ( 'NONE', #47835, #31923 ) ;
#231670=AXIS2_PLACEMENT_3D ( 'NONE', #138473, #99350, #41990 ) ;
#231676=CARTESIAN_POINT ( 'NONE',  ( -22.32929514600008503, 0.09907567811392146984, 7.578647565376503081 ) ) ;
#231680=LINE ( 'NONE', #114279, #105823 ) ;
#231681=DIRECTION ( 'NONE',  ( 0.000000000000000000, 1.000000000000000000, 1.734723475976807292E-15 ) ) ;
#231683=VERTEX_POINT ( 'NONE', #195195 ) ;
#231691=DIRECTION ( 'NONE',  ( -4.408576920032448588E-17, 0.1350103645451876944, 0.9908441862701601321 ) ) ;
#231704=DIRECTION ( 'NONE',  ( 1.000000000000000000, -0.000000000000000000, 0.000000000000000000 ) ) ;
#231731=EDGE_LOOP ( 'NONE', ( #77846, #219202, #242184 ) ) ;
#231742=ORIENTED_EDGE ( 'NONE', *, *, #84414, .F. ) ;
#231762=CARTESIAN_POINT ( 'NONE',  ( -21.64999999999999858, 7.349999999999998757, -21.15000000000000213 ) ) ;
#231770=ORIENTED_EDGE ( 'NONE', *, *, #201299, .T. ) ;
#231816=DIRECTION ( 'NONE',  ( -1.000000000000000000, 0.000000000000000000, 0.000000000000000000 ) ) ;
#231848=AXIS2_PLACEMENT_3D ( 'NONE', #170470, #231691, #53027 ) ;
#231858=ORIENTED_EDGE ( 'NONE', *, *, #119979, .T. ) ;
#231892=CARTESIAN_POINT ( 'NONE',  ( -18.41809261886924887, -9.682403314756559354, -40.15684355009123152 ) ) ;
#231935=CARTESIAN_POINT ( 'NONE',  ( 18.43473516226073627, -9.494942282758197294, -7.045898683349446578 ) ) ;
#231952=CARTESIAN_POINT ( 'NONE',  ( 18.50000000000000355, -9.400000000000000355, -40.38204184817267617 ) ) ;
#231959=CARTESIAN_POINT ( 'NONE',  ( -21.05000000000000071, -1.162701749938009677, -7.900000000000000355 ) ) ;
#231969=CARTESIAN_POINT ( 'NONE',  ( 21.30000000000002558, 4.959819536546778628E-16, -4.049999999999998934 ) ) ;
#231978=DIRECTION ( 'NONE',  ( 1.000000000000000000, 0.000000000000000000, 0.000000000000000000 ) ) ;
#231985=EDGE_CURVE ( 'NONE', #233652, #89621, #203277, .T. ) ;
#231987=ORIENTED_EDGE ( 'NONE', *, *, #115905, .T. ) ;
#232034=LINE ( 'NONE', #71677, #245306 ) ;
#232048=ORIENTED_EDGE ( 'NONE', *, *, #167737, .T. ) ;
#232054=CARTESIAN_POINT ( 'NONE',  ( 18.49999999999999289, 10.20857864376268509, -24.76715728752538226 ) ) ;
#232100=DIRECTION ( 'NONE',  ( 0.000000000000000000, 0.4999999999999956701, -0.8660254037844411501 ) ) ;
#232119=CARTESIAN_POINT ( 'NONE',  ( 18.39999999999999858, -9.499999999999998224, -40.41465834296967330 ) ) ;
#232149=AXIS2_PLACEMENT_3D ( 'NONE', #107550, #248359, #67151 ) ;
#232172=DIRECTION ( 'NONE',  ( 0.000000000000000000, 0.000000000000000000, -1.000000000000000000 ) ) ;
#232183=DIRECTION ( 'NONE',  ( 0.000000000000000000, 0.000000000000000000, -1.000000000000000000 ) ) ;
#232204=VERTEX_POINT ( 'NONE', #206101 ) ;
#232219=DIRECTION ( 'NONE',  ( -1.000000000000000000, -3.265361837132813093E-16, 0.000000000000000000 ) ) ;
#232229=CARTESIAN_POINT ( 'NONE',  ( -18.50000000000000000, 11.64999999999999680, 11.75000000000000000 ) ) ;
#232234=ADVANCED_FACE ( 'NONE', ( #204796 ), #141117, .F. ) ;
#232248=EDGE_CURVE ( 'NONE', #24982, #112457, #28720, .T. ) ;
#232270=LINE ( 'NONE', #31512, #41201 ) ;
#232282=DIRECTION ( 'NONE',  ( -0.000000000000000000, 0.1350103645451876666, 0.9908441862701600211 ) ) ;
#232312=LINE ( 'NONE', #13253, #91614 ) ;
#232313=CIRCLE ( 'NONE', #82224, 0.9750000000000036415 ) ;
#232342=ORIENTED_EDGE ( 'NONE', *, *, #24957, .T. ) ;
#232349=AXIS2_PLACEMENT_3D ( 'NONE', #32185, #55530, #16469 ) ;
#232357=VECTOR ( 'NONE', #168933, 1000.000000000000114 ) ;
#232399=AXIS2_PLACEMENT_3D ( 'NONE', #69661, #246984, #113905 ) ;
#232401=CIRCLE ( 'NONE', #74204, 0.09999999999999843736 ) ;
#232421=ORIENTED_EDGE ( 'NONE', *, *, #211986, .T. ) ;
#232433=DIRECTION ( 'NONE',  ( 1.000000000000000000, 0.000000000000000000, 0.000000000000000000 ) ) ;
#232435=ADVANCED_FACE ( 'NONE', ( #119863 ), #94271, .T. ) ;
#232441=CIRCLE ( 'NONE', #15971, 6.329289321881367059 ) ;
#232443=CARTESIAN_POINT ( 'NONE',  ( 23.24999999999999645, 0.000000000000000000, -33.50000000000000000 ) ) ;
#232447=ORIENTED_EDGE ( 'NONE', *, *, #241587, .F. ) ;
#232453=ORIENTED_EDGE ( 'NONE', *, *, #85094, .T. ) ;
#232462=DIRECTION ( 'NONE',  ( 0.000000000000000000, 0.000000000000000000, -1.000000000000000000 ) ) ;
#232506=ORIENTED_EDGE ( 'NONE', *, *, #115804, .F. ) ;
#232544=DIRECTION ( 'NONE',  ( 0.000000000000000000, 0.8700118002898322711, -0.4930308989875231696 ) ) ;
#232567=DIRECTION ( 'NONE',  ( -1.000000000000000000, 0.000000000000000000, -3.469446951953635015E-14 ) ) ;
#232581=PLANE ( 'NONE',  #188176 ) ;
#232632=EDGE_LOOP ( 'NONE', ( #88555, #2693, #152577, #43079, #229518 ) ) ;
#232653=ORIENTED_EDGE ( 'NONE', *, *, #116759, .F. ) ;
#232675=CIRCLE ( 'NONE', #3697, 11.80000000000000249 ) ;
#232682=ORIENTED_EDGE ( 'NONE', *, *, #237852, .T. ) ;
#232688=DIRECTION ( 'NONE',  ( -0.000000000000000000, -0.000000000000000000, 1.000000000000000000 ) ) ;
#232691=LINE ( 'NONE', #69766, #174344 ) ;
#232700=EDGE_CURVE ( 'NONE', #168131, #255533, #74688, .T. ) ;
#232733=CARTESIAN_POINT ( 'NONE',  ( -23.25000000000000000, 10.33248238082518711, -39.09484654391314962 ) ) ;
#232743=ORIENTED_EDGE ( 'NONE', *, *, #8325, .F. ) ;
#232747=VECTOR ( 'NONE', #209046, 1000.000000000000000 ) ;
#232762=DIRECTION ( 'NONE',  ( -7.304098846218201720E-16, 1.000000000000000000, 0.000000000000000000 ) ) ;
#232766=DIRECTION ( 'NONE',  ( 1.000000000000000000, 0.000000000000000000, 0.000000000000000000 ) ) ;
#232846=FACE_OUTER_BOUND ( 'NONE', #225259, .T. ) ;
#232849=ORIENTED_EDGE ( 'NONE', *, *, #15958, .T. ) ;
#232871=FACE_OUTER_BOUND ( 'NONE', #104651, .T. ) ;
#232917=ADVANCED_FACE ( 'NONE', ( #187222 ), #149384, .F. ) ;
#232952=CARTESIAN_POINT ( 'NONE',  ( 22.00356870068479154, -2.593051619917821170E-12, 7.254242361760407043 ) ) ;
#232971=ORIENTED_EDGE ( 'NONE', *, *, #202739, .F. ) ;
#232983=TOROIDAL_SURFACE ( 'NONE', #49797, 11.70000000000000462, 0.1000000000000000056 ) ;
#233000=CIRCLE ( 'NONE', #195411, 0.09999999999999939493 ) ;
#233002=CARTESIAN_POINT ( 'NONE',  ( -23.25000000000000000, 0.000000000000000000, -35.60000000000000853 ) ) ;
#233005=CARTESIAN_POINT ( 'NONE',  ( -22.59999999999999787, 11.74987124437650721, 0.06542959101367804009 ) ) ;
#233027=CARTESIAN_POINT ( 'NONE',  ( 20.85000000000000142, 11.75000000000000355, -26.71613433702190932 ) ) ;
#233029=CARTESIAN_POINT ( 'NONE',  ( -18.52139480978223318, -9.481358845066894858, -7.024556567119067729 ) ) ;
#233113=AXIS2_PLACEMENT_3D ( 'NONE', #256576, #174590, #139222 ) ;
#233139=CARTESIAN_POINT ( 'NONE',  ( 20.94999999999999929, 6.649999999999999467, -12.15000000000000036 ) ) ;
#233145=ORIENTED_EDGE ( 'NONE', *, *, #189274, .F. ) ;
#233159=EDGE_LOOP ( 'NONE', ( #28127, #46910, #22608, #16606, #59361 ) ) ;
#233175=CARTESIAN_POINT ( 'NONE',  ( 21.13461538461538325, 10.61458296202553697, -12.35000000000000320 ) ) ;
#233207=LINE ( 'NONE', #156241, #138909 ) ;
#233219=ORIENTED_EDGE ( 'NONE', *, *, #214526, .F. ) ;
#233232=EDGE_LOOP ( 'NONE', ( #83451, #123242, #83887, #126682 ) ) ;
#233305=ORIENTED_EDGE ( 'NONE', *, *, #216542, .F. ) ;
#233325=VERTEX_POINT ( 'NONE', #229877 ) ;
#233391=CARTESIAN_POINT ( 'NONE',  ( 22.50000000000000000, 0.09999999999999939493, 11.64957080754479968 ) ) ;
#233445=VECTOR ( 'NONE', #81966, 1000.000000000000000 ) ;
#233459=TOROIDAL_SURFACE ( 'NONE', #125114, 11.65000000000000036, 0.1000000000000000056 ) ;
#233476=DIRECTION ( 'NONE',  ( 1.000000000000000000, 7.304098846218134667E-16, -0.000000000000000000 ) ) ;
#233509=FACE_OUTER_BOUND ( 'NONE', #87367, .T. ) ;
#233525=CARTESIAN_POINT ( 'NONE',  ( -23.15000000000000213, -8.596261682242989366, -24.04987248284972523 ) ) ;
#233533=CARTESIAN_POINT ( 'NONE',  ( 21.08198257630413508, 6.336596734015063959, 0.07264332378460747197 ) ) ;
#233539=AXIS2_PLACEMENT_3D ( 'NONE', #246898, #82662, #27900 ) ;
#233552=ORIENTED_EDGE ( 'NONE', *, *, #238878, .T. ) ;
#233568=CARTESIAN_POINT ( 'NONE',  ( 20.95378194480896639, 10.53491199154278668, -7.565054148147858371 ) ) ;
#233584=VECTOR ( 'NONE', #76316, 1000.000000000000000 ) ;
#233586=AXIS2_PLACEMENT_3D ( 'NONE', #121924, #22839, #3226 ) ;
#233592=AXIS2_PLACEMENT_3D ( 'NONE', #176049, #216424, #76911 ) ;
#233597=AXIS2_PLACEMENT_3D ( 'NONE', #2356, #83153, #44075 ) ;
#233645=VERTEX_POINT ( 'NONE', #46745 ) ;
#233646=B_SPLINE_CURVE_WITH_KNOTS ( 'NONE', 3,
 ( #177926, #193628, #116651, #256094, #172823, #15004 ),
 .UNSPECIFIED., .F., .F.,
 ( 4, 2, 4 ),
 ( 0.000000000000000000, 0.0001568709654583420778, 0.0003137419309166841557 ),
 .UNSPECIFIED. ) ;
#233652=VERTEX_POINT ( 'NONE', #224101 ) ;
#233665=DIRECTION ( 'NONE',  ( -1.000000000000000000, 0.000000000000000000, 0.000000000000000000 ) ) ;
#233676=ORIENTED_EDGE ( 'NONE', *, *, #154338, .T. ) ;
#233680=DIRECTION ( 'NONE',  ( 1.000000000000000000, -7.304098846218133681E-16, 4.607487905232622991E-31 ) ) ;
#233686=DIRECTION ( 'NONE',  ( -0.000000000000000000, 1.000000000000000000, -1.224646799147352961E-16 ) ) ;
#233754=PLANE ( 'NONE',  #160618 ) ;
#233796=DIRECTION ( 'NONE',  ( 0.000000000000000000, 0.1350103645451904977, -0.9908441862701596881 ) ) ;
#233811=FACE_OUTER_BOUND ( 'NONE', #184671, .T. ) ;
#233879=DIRECTION ( 'NONE',  ( -0.000000000000000000, -0.000000000000000000, -1.000000000000000000 ) ) ;
#233889=DIRECTION ( 'NONE',  ( 1.000000000000000000, 0.000000000000000000, 0.000000000000000000 ) ) ;
#233895=CARTESIAN_POINT ( 'NONE',  ( 21.05000000000000071, -11.64999999999999147, 0.000000000000000000 ) ) ;
#233901=EDGE_CURVE ( 'NONE', #96622, #34317, #133457, .T. ) ;
#233908=VERTEX_POINT ( 'NONE', #199105 ) ;
#233931=ORIENTED_EDGE ( 'NONE', *, *, #222843, .T. ) ;
#233946=CARTESIAN_POINT ( 'NONE',  ( 20.94999999999999929, 1.835341550224413698, -11.55515129256298401 ) ) ;
#233976=ORIENTED_EDGE ( 'NONE', *, *, #121766, .F. ) ;
#233983=LINE ( 'NONE', #89328, #232357 ) ;
#233988=EDGE_CURVE ( 'NONE', #106299, #214079, #100296, .T. ) ;
#233995=EDGE_CURVE ( 'NONE', #11322, #26533, #17140, .T. ) ;
#234017=DIRECTION ( 'NONE',  ( 1.000000000000000000, 0.000000000000000000, -0.000000000000000000 ) ) ;
#234035=EDGE_CURVE ( 'NONE', #130496, #216736, #33734, .T. ) ;
#234089=TOROIDAL_SURFACE ( 'NONE', #155025, 0.2000000000000000111, 0.1000000000000000056 ) ;
#234090=B_SPLINE_CURVE_WITH_KNOTS ( 'NONE', 3,
 ( #152033, #148151, #133720, #247239, #227681, #169042, #89452 ),
 .UNSPECIFIED., .F., .F.,
 ( 4, 3, 4 ),
 ( 0.000000000000000000, 1.860045280645836611E-05, 5.251155757304663829E-05 ),
 .UNSPECIFIED. ) ;
#234101=EDGE_LOOP ( 'NONE', ( #227202, #240760, #41058, #24681 ) ) ;
#234140=CARTESIAN_POINT ( 'NONE',  ( 18.59999999999999787, -9.399999999999998579, -40.38204184817267617 ) ) ;
#234145=CYLINDRICAL_SURFACE ( 'NONE', #51317, 0.09999999999999939493 ) ;
#234190=ORIENTED_EDGE ( 'NONE', *, *, #131816, .F. ) ;
#234193=ORIENTED_EDGE ( 'NONE', *, *, #67911, .F. ) ;
#234210=ORIENTED_EDGE ( 'NONE', *, *, #106735, .T. ) ;
#234226=CARTESIAN_POINT ( 'NONE',  ( 20.04142135623730070, 11.65000000000000391, 11.75000000000000000 ) ) ;
#234230=EDGE_CURVE ( 'NONE', #172615, #145230, #8742, .T. ) ;
#234235=DIRECTION ( 'NONE',  ( -0.000000000000000000, -0.1350103645451928291, -0.9908441862701594660 ) ) ;
#234238=EDGE_CURVE ( 'NONE', #4508, #91559, #354, .T. ) ;
#234239=DIRECTION ( 'NONE',  ( -2.561896900575096011E-15, -0.5907332058517279494, 0.8068669527897025517 ) ) ;
#234268=ORIENTED_EDGE ( 'NONE', *, *, #84155, .T. ) ;
#234284=DIRECTION ( 'NONE',  ( 1.000000000000000000, 0.000000000000000000, -0.000000000000000000 ) ) ;
#234293=VECTOR ( 'NONE', #121129, 1000.000000000000000 ) ;
#234296=EDGE_CURVE ( 'NONE', #11112, #56184, #119401, .T. ) ;
#234298=CARTESIAN_POINT ( 'NONE',  ( -20.94999999999999929, -1.162701749938009677, -7.900000000000000355 ) ) ;
#234302=VERTEX_POINT ( 'NONE', #75030 ) ;
#234348=DIRECTION ( 'NONE',  ( 0.000000000000000000, 0.000000000000000000, 1.000000000000000000 ) ) ;
#234360=DIRECTION ( 'NONE',  ( 1.000000000000000000, 0.000000000000000000, 0.000000000000000000 ) ) ;
#234365=CARTESIAN_POINT ( 'NONE',  ( 22.59999999999999787, 11.64957080754479968, 0.09999999999999592548 ) ) ;
#234368=EDGE_CURVE ( 'NONE', #192659, #106265, #50599, .T. ) ;
#234387=CARTESIAN_POINT ( 'NONE',  ( 18.52351027002948314, -9.642162904695185333, -40.21504695050978029 ) ) ;
#234398=FACE_BOUND ( 'NONE', #81679, .T. ) ;
#234401=AXIS2_PLACEMENT_3D ( 'NONE', #183647, #4965, #84481 ) ;
#234439=LINE ( 'NONE', #248897, #51949 ) ;
#234459=CARTESIAN_POINT ( 'NONE',  ( -21.05000000000000071, 6.307425219565403474, -0.01681986838567561815 ) ) ;
#234463=CARTESIAN_POINT ( 'NONE',  ( 18.49999999999999289, 10.29270135740183179, -38.95736188715193293 ) ) ;
#234468=CARTESIAN_POINT ( 'NONE',  ( 18.59999994388910238, -9.363566187071151958, -7.181117236800915293 ) ) ;
#234483=CARTESIAN_POINT ( 'NONE',  ( 18.40916198585732388, -9.500000000000000000, -40.10018963182346852 ) ) ;
#234498=CARTESIAN_POINT ( 'NONE',  ( -20.64999999999999858, 7.249999999999999112, -12.34999999999999964 ) ) ;
#234510=DIRECTION ( 'NONE',  ( 0.000000000000000000, -0.9908441862701620195, -0.1350103645451731504 ) ) ;
#234532=EDGE_CURVE ( 'NONE', #122037, #80105, #75593, .T. ) ;
#234559=CARTESIAN_POINT ( 'NONE',  ( -21.10320863425827298, 0.02502225122710637073, 6.400277386459231721 ) ) ;
#234571=EDGE_LOOP ( 'NONE', ( #95403, #223398, #58944, #137299 ) ) ;
#234576=ORIENTED_EDGE ( 'NONE', *, *, #231207, .T. ) ;
#234578=EDGE_CURVE ( 'NONE', #241989, #56194, #63071, .T. ) ;
#234586=PLANE ( 'NONE',  #97901 ) ;
#234607=CIRCLE ( 'NONE', #34924, 0.09999999999999939493 ) ;
#234619=ORIENTED_EDGE ( 'NONE', *, *, #45917, .T. ) ;
#234636=AXIS2_PLACEMENT_3D ( 'NONE', #226958, #206113, #48317 ) ;
#234641=ORIENTED_EDGE ( 'NONE', *, *, #21925, .T. ) ;
#234675=DIRECTION ( 'NONE',  ( 1.000000000000000000, -0.000000000000000000, -0.000000000000000000 ) ) ;
#234678=CARTESIAN_POINT ( 'NONE',  ( -22.49072729836729678, 0.05648193273361867134, 11.65000824915494171 ) ) ;
#234682=LINE ( 'NONE', #177311, #237523 ) ;
#234696=CARTESIAN_POINT ( 'NONE',  ( 18.59999999999999076, 6.450000000000001066, -10.01702717044001822 ) ) ;
#234715=CARTESIAN_POINT ( 'NONE',  ( 20.94999999999999929, 0.000000000000000000, -33.50000000000000000 ) ) ;
#234734=DIRECTION ( 'NONE',  ( 0.000000000000000000, 0.000000000000000000, -1.000000000000000000 ) ) ;
#234739=AXIS2_PLACEMENT_3D ( 'NONE', #216863, #39559, #235160 ) ;
#234752=EDGE_CURVE ( 'NONE', #16790, #191917, #187995, .T. ) ;
#234761=DIRECTION ( 'NONE',  ( 1.000000000000000000, 0.000000000000000000, 0.000000000000000000 ) ) ;
#234770=LINE ( 'NONE', #47450, #7346 ) ;
#234773=DIRECTION ( 'NONE',  ( -0.000000000000000000, -0.000000000000000000, 1.000000000000000000 ) ) ;
#234802=ADVANCED_FACE ( 'NONE', ( #232871 ), #216821, .T. ) ;
#234803=CARTESIAN_POINT ( 'NONE',  ( 21.07933241753356768, 6.328645948379748809, 0.09337959041930479764 ) ) ;
#234837=LINE ( 'NONE', #113602, #117801 ) ;
#234840=EDGE_CURVE ( 'NONE', #56815, #197037, #42356, .T. ) ;
#234866=CARTESIAN_POINT ( 'NONE',  ( -18.59999999999999787, 0.000000000000000000, 0.000000000000000000 ) ) ;
#234869=AXIS2_PLACEMENT_3D ( 'NONE', #34488, #54017, #210533 ) ;
#234892=CARTESIAN_POINT ( 'NONE',  ( -23.25000000000000000, 2.600000000000000089, -13.22462192276210224 ) ) ;
#234900=VERTEX_POINT ( 'NONE', #81447 ) ;
#234935=EDGE_LOOP ( 'NONE', ( #218050, #183917, #229268, #222484 ) ) ;
#234940=EDGE_LOOP ( 'NONE', ( #144080, #119472 ) ) ;
#234945=DIRECTION ( 'NONE',  ( 0.000000000000000000, 0.000000000000000000, -1.000000000000000000 ) ) ;
#235016=AXIS2_PLACEMENT_3D ( 'NONE', #67228, #144180, #244575 ) ;
#235035=FACE_OUTER_BOUND ( 'NONE', #178760, .T. ) ;
#235074=VERTEX_POINT ( 'NONE', #27965 ) ;
#235089=EDGE_CURVE ( 'NONE', #34172, #40483, #30520, .T. ) ;
#235103=DIRECTION ( 'NONE',  ( 2.978066053179067751E-16, -1.000000000000000000, 0.000000000000000000 ) ) ;
#235110=EDGE_CURVE ( 'NONE', #61026, #183417, #4979, .T. ) ;
#235114=DIRECTION ( 'NONE',  ( 0.000000000000000000, 8.673617379884087537E-15, -1.000000000000000000 ) ) ;
#235152=ADVANCED_FACE ( 'NONE', ( #94310 ), #232581, .F. ) ;
#235160=DIRECTION ( 'NONE',  ( 0.000000000000000000, 0.1495327102803663544, -0.9887567792719339499 ) ) ;
#235187=ORIENTED_EDGE ( 'NONE', *, *, #79979, .T. ) ;
#235207=AXIS2_PLACEMENT_3D ( 'NONE', #190539, #129259, #250476 ) ;
#235210=AXIS2_PLACEMENT_3D ( 'NONE', #121359, #200855, #146005 ) ;
#235215=ORIENTED_EDGE ( 'NONE', *, *, #14375, .F. ) ;
#235225=ORIENTED_EDGE ( 'NONE', *, *, #73537, .F. ) ;
#235233=CARTESIAN_POINT ( 'NONE',  ( -20.94999999999999929, 11.75000000000000000, -7.014805770654001016 ) ) ;
#235251=CYLINDRICAL_SURFACE ( 'NONE', #3883, 0.09999999999999939493 ) ;
#235262=CARTESIAN_POINT ( 'NONE',  ( 21.05563370358598263, 10.72423035584650997, -12.18309081596307308 ) ) ;
#235279=( BOUNDED_SURFACE ( )  B_SPLINE_SURFACE ( 3, 2, ( 
 ( #68911, #148436, #208425 ),
 ( #29801, #109279, #51867 ),
 ( #17883, #251368, #16630 ),
 ( #171877, #216082, #154870 ),
 ( #72774, #195278, #170612 ),
 ( #213517, #116998, #113146 ) ),
 .UNSPECIFIED., .F., .F., .T. ) 
 B_SPLINE_SURFACE_WITH_KNOTS ( ( 4, 2, 4 ),
 ( 3, 3 ),
 ( 0.0001342700090130047525, 0.0002909192928057360351, 0.0004475685765984672906 ),
 ( 0.000000000000000000, 1.000000000000000000 ),
 .UNSPECIFIED. ) 
 GEOMETRIC_REPRESENTATION_ITEM ( )  RATIONAL_B_SPLINE_SURFACE ( (
 ( 1.000000000000000000, 0.7250110520819876836, 1.000000000000000000),
 ( 1.000000000000000000, 0.7257599279134024917, 1.000000000000000000),
 ( 1.000000000000000000, 0.7137594617284269694, 1.000000000000000000),
 ( 1.000000000000000000, 0.6959270178809834340, 1.000000000000000000),
 ( 1.000000000000000000, 0.6919879549339010838, 1.000000000000000000),
 ( 1.000000000000000000, 0.7071067811865414665, 1.000000000000000000) ) ) 
 REPRESENTATION_ITEM ( '' )  SURFACE ( )  );
#235284=ORIENTED_EDGE ( 'NONE', *, *, #123370, .F. ) ;
#235296=CARTESIAN_POINT ( 'NONE',  ( -22.39999999999999503, -5.963111948670274387E-16, 7.790779598373403836 ) ) ;
#235312=DIRECTION ( 'NONE',  ( 1.000000000000000000, 0.000000000000000000, 0.000000000000000000 ) ) ;
#235336=DIRECTION ( 'NONE',  ( -1.000000000000000000, 0.000000000000000000, 0.000000000000000000 ) ) ;
#235398=CARTESIAN_POINT ( 'NONE',  ( -23.24999999999999645, -9.600000000000003197, -40.10018939122204529 ) ) ;
#235455=ADVANCED_FACE ( 'NONE', ( #244090 ), #79440, .F. ) ;
#235477=EDGE_CURVE ( 'NONE', #253517, #183242, #35366, .T. ) ;
#235478=FACE_OUTER_BOUND ( 'NONE', #38058, .T. ) ;
#235485=DIRECTION ( 'NONE',  ( -0.000000000000000000, -0.000000000000000000, 1.000000000000000000 ) ) ;
#235490=ORIENTED_EDGE ( 'NONE', *, *, #50718, .T. ) ;
#235546=CARTESIAN_POINT ( 'NONE',  ( 20.95289811251229750, 8.893168004458594567, -8.501809493918521810 ) ) ;
#235552=VERTEX_POINT ( 'NONE', #11933 ) ;
#235565=FACE_OUTER_BOUND ( 'NONE', #203076, .T. ) ;
#235584=ORIENTED_EDGE ( 'NONE', *, *, #221273, .T. ) ;
#235664=AXIS2_PLACEMENT_3D ( 'NONE', #46545, #107819, #126083 ) ;
#235665=EDGE_LOOP ( 'NONE', ( #240060, #96828, #198309, #246513, #234190, #82113, #177248, #214105, #21852, #66121, #213985, #3936, #83832, #178741, #241340, #40097 ) ) ;
#235674=ORIENTED_EDGE ( 'NONE', *, *, #193075, .F. ) ;
#235692=DIRECTION ( 'NONE',  ( -1.000000000000000000, -2.952720810173289112E-16, 0.000000000000000000 ) ) ;
#235766=VECTOR ( 'NONE', #122399, 1000.000000000000000 ) ;
#235836=EDGE_LOOP ( 'NONE', ( #215057, #222421, #108457, #118520 ) ) ;
#235845=FACE_OUTER_BOUND ( 'NONE', #241040, .T. ) ;
#235886=ORIENTED_EDGE ( 'NONE', *, *, #18183, .T. ) ;
#235888=DIRECTION ( 'NONE',  ( 1.000000000000000000, 0.000000000000000000, 0.000000000000000000 ) ) ;
#235905=CIRCLE ( 'NONE', #15358, 0.1000000000000002831 ) ;
#235906=DIRECTION ( 'NONE',  ( 1.000000000000000000, 2.952720810173289112E-16, -0.000000000000000000 ) ) ;
#235929=ORIENTED_EDGE ( 'NONE', *, *, #27637, .F. ) ;
#235934=CARTESIAN_POINT ( 'NONE',  ( 23.15000000000000213, -9.000000000000000000, -23.60603087734755690 ) ) ;
#235937=ADVANCED_FACE ( 'NONE', ( #213647 ), #181110, .T. ) ;
#235948=CARTESIAN_POINT ( 'NONE',  ( -22.48479450179659977, 0.04699158118688477603, 11.64999844625161352 ) ) ;
#235949=CARTESIAN_POINT ( 'NONE',  ( -18.59999999999999787, -1.736705739467587772, -45.01742258762372728 ) ) ;
#236005=CARTESIAN_POINT ( 'NONE',  ( 20.94999999999999929, -9.000000000000000000, -23.60603087734755690 ) ) ;
#236051=DIRECTION ( 'NONE',  ( 0.000000000000000000, -0.9915357197604853789, 0.1298341882520022694 ) ) ;
#236056=CARTESIAN_POINT ( 'NONE',  ( 20.94999999999999929, 5.499999999999998224, -21.09473398108690390 ) ) ;
#236123=ADVANCED_FACE ( 'NONE', ( #143073 ), #64066, .F. ) ;
#236126=AXIS2_PLACEMENT_3D ( 'NONE', #8969, #132790, #110635 ) ;
#236139=EDGE_CURVE ( 'NONE', #242875, #107696, #203061, .T. ) ;
#236144=AXIS2_PLACEMENT_3D ( 'NONE', #165057, #67236, #105033 ) ;
#236154=DIRECTION ( 'NONE',  ( -1.000000000000000000, 0.000000000000000000, 0.000000000000000000 ) ) ;
#236158=AXIS2_PLACEMENT_3D ( 'NONE', #32343, #216067, #37462 ) ;
#236211=DIRECTION ( 'NONE',  ( 0.000000000000000000, -0.4999999999999799605, 0.8660254037844502539 ) ) ;
#236233=AXIS2_PLACEMENT_3D ( 'NONE', #64859, #158861, #218793 ) ;
#236247=EDGE_LOOP ( 'NONE', ( #194511, #30020, #119731, #43254 ) ) ;
#236252=CARTESIAN_POINT ( 'NONE',  ( 20.94999999999999929, 10.72371710470752149, -7.664913569087605794 ) ) ;
#236260=AXIS2_PLACEMENT_3D ( 'NONE', #229522, #224368, #207400 ) ;
#236276=AXIS2_PLACEMENT_3D ( 'NONE', #99511, #179117, #94395 ) ;
#236290=DIRECTION ( 'NONE',  ( 0.000000000000000000, 0.1495327102803663544, -0.9887567792719339499 ) ) ;
#236327=EDGE_LOOP ( 'NONE', ( #181117, #134096, #183079 ) ) ;
#236331=CARTESIAN_POINT ( 'NONE',  ( 22.49533356619861024, 11.65000000630418597, 0.06512258032273263164 ) ) ;
#236335=EDGE_CURVE ( 'NONE', #251409, #77132, #226741, .T. ) ;
#236376=CARTESIAN_POINT ( 'NONE',  ( 22.60000000000000142, 11.74956712348939192, 0.1008583690987087389 ) ) ;
#236386=AXIS2_PLACEMENT_3D ( 'NONE', #236056, #256849, #118702 ) ;
#236404=TOROIDAL_SURFACE ( 'NONE', #111506, 0.2000000000000000111, 0.1000000000000000056 ) ;
#236415=DIRECTION ( 'NONE',  ( 0.000000000000000000, 0.000000000000000000, 1.000000000000000000 ) ) ;
#236452=DIRECTION ( 'NONE',  ( 0.000000000000000000, 0.000000000000000000, -1.000000000000000000 ) ) ;
#236467=ORIENTED_EDGE ( 'NONE', *, *, #75131, .T. ) ;
#236469=EDGE_CURVE ( 'NONE', #82580, #79894, #139238, .T. ) ;
#236490=FACE_OUTER_BOUND ( 'NONE', #196311, .T. ) ;
#236509=CARTESIAN_POINT ( 'NONE',  ( 20.46382478191414833, 8.901379558702615213, -8.545728094883093817 ) ) ;
#236524=ADVANCED_FACE ( 'NONE', ( #109749 ), #228446, .T. ) ;
#236569=AXIS2_PLACEMENT_3D ( 'NONE', #65557, #145083, #45991 ) ;
#236573=DIRECTION ( 'NONE',  ( 4.377807931758638789E-15, 0.2605042016806672911, 0.9654727137038716656 ) ) ;
#236575=AXIS2_PLACEMENT_3D ( 'NONE', #228494, #112392, #150245 ) ;
#236585=CIRCLE ( 'NONE', #157532, 0.1000000000000002831 ) ;
#236620=CARTESIAN_POINT ( 'NONE',  ( 21.05000000000000071, -11.48912529307605546, -30.50000000000000000 ) ) ;
#236660=EDGE_LOOP ( 'NONE', ( #142756, #48813, #172953, #143424 ) ) ;
#236676=TOROIDAL_SURFACE ( 'NONE', #41087, 11.89999999999999858, 0.1000000000000000056 ) ;
#236681=FACE_OUTER_BOUND ( 'NONE', #24041, .T. ) ;
#236698=( BOUNDED_SURFACE ( )  B_SPLINE_SURFACE ( 3, 2, ( 
 ( #98753, #216163, #77937 ),
 ( #37557, #79211, #36281 ),
 ( #100047, #179636, #939 ),
 ( #80474, #160078, #156233 ),
 ( #239599, #220029, #120955 ),
 ( #83042, #67374, #186036 ) ),
 .UNSPECIFIED., .F., .F., .F. ) 
 B_SPLINE_SURFACE_WITH_KNOTS ( ( 4, 2, 4 ),
 ( 3, 3 ),
 ( 0.0001300404313046605199, 0.0003183318589266616056, 0.0005066232865486627185 ),
 ( 0.000000000000000000, 1.000000000000000000 ),
 .UNSPECIFIED. ) 
 GEOMETRIC_REPRESENTATION_ITEM ( )  RATIONAL_B_SPLINE_SURFACE ( (
 ( 1.000000000000000000, 0.7071067811865475727, 1.000000000000000000),
 ( 1.000000000000000000, 0.7625113560539543700, 1.000000000000000000),
 ( 1.000000000000000000, 0.8126073484689319004, 1.000000000000000000),
 ( 1.000000000000000000, 0.8923049332731584071, 1.000000000000000000),
 ( 1.000000000000000000, 0.9231914937770194785, 1.000000000000000000),
 ( 1.000000000000000000, 0.9238795325112901802, 1.000000000000000000) ) ) 
 REPRESENTATION_ITEM ( '' )  SURFACE ( )  );
#236728=DIRECTION ( 'NONE',  ( 0.000000000000000000, 1.000000000000000000, 0.000000000000000000 ) ) ;
#236729=ADVANCED_FACE ( 'NONE', ( #80889 ), #181314, .T. ) ;
#236772=DIRECTION ( 'NONE',  ( -1.000000000000000000, -1.836970198721029934E-16, 0.000000000000000000 ) ) ;
#236776=AXIS2_PLACEMENT_3D ( 'NONE', #3287, #42433, #236772 ) ;
#236782=DIRECTION ( 'NONE',  ( -1.000000000000000000, 0.000000000000000000, 0.000000000000000000 ) ) ;
#236830=CARTESIAN_POINT ( 'NONE',  ( 20.95483826173900255, 8.876166204769987189, -8.546275552899514238 ) ) ;
#236838=ORIENTED_EDGE ( 'NONE', *, *, #30569, .F. ) ;
#236844=CARTESIAN_POINT ( 'NONE',  ( -18.39999999999999858, -9.519327731092436906, -6.972976376559334888 ) ) ;
#236935=AXIS2_PLACEMENT_3D ( 'NONE', #198928, #20319, #180662 ) ;
#236963=AXIS2_PLACEMENT_3D ( 'NONE', #242646, #64022, #185254 ) ;
#236972=CARTESIAN_POINT ( 'NONE',  ( -20.94999999999999929, 0.000000000000000000, -21.80000000000000071 ) ) ;
#236992=CARTESIAN_POINT ( 'NONE',  ( 23.24999999999999645, 0.000000000000000000, -33.50000000000000000 ) ) ;
#236994=DIRECTION ( 'NONE',  ( -1.000000000000000000, 0.000000000000000000, 0.000000000000000000 ) ) ;
#237029=DIRECTION ( 'NONE',  ( -0.000000000000000000, -0.1298341882520022694, -0.9915357197604853789 ) ) ;
#237048=CARTESIAN_POINT ( 'NONE',  ( 18.51565452909384391, -9.352859338836742253, -7.194909321233445176 ) ) ;
#237066=CARTESIAN_POINT ( 'NONE',  ( 20.84999999999998721, 10.33248238082518711, -39.09484654391314962 ) ) ;
#237088=CIRCLE ( 'NONE', #124659, 0.8750000000000007772 ) ;
#237096=EDGE_CURVE ( 'NONE', #6556, #176194, #210381, .T. ) ;
#237108=CARTESIAN_POINT ( 'NONE',  ( -23.25000000000000000, 4.250000000000000000, -21.14999999999999858 ) ) ;
#237122=CARTESIAN_POINT ( 'NONE',  ( -21.64999999999999858, 7.349999999999998757, -12.25000000000000000 ) ) ;
#237123=DIRECTION ( 'NONE',  ( 0.000000000000000000, 0.000000000000000000, 1.000000000000000000 ) ) ;
#237133=CARTESIAN_POINT ( 'NONE',  ( -21.11101077989000174, 0.01528526891428022040, 6.423684734726124113 ) ) ;
#237140=FACE_OUTER_BOUND ( 'NONE', #45378, .T. ) ;
#237146=CARTESIAN_POINT ( 'NONE',  ( -18.59999999999999787, 7.021664781900089913, -37.33356540189728889 ) ) ;
#237158=AXIS2_PLACEMENT_3D ( 'NONE', #75863, #155443, #234945 ) ;
#237164=EDGE_CURVE ( 'NONE', #207105, #71370, #243687, .T. ) ;
#237182=CARTESIAN_POINT ( 'NONE',  ( 20.94999999999999929, -1.835341550224413698, -11.55515129256298046 ) ) ;
#237215=VECTOR ( 'NONE', #119820, 1000.000000000000000 ) ;
#237223=CARTESIAN_POINT ( 'NONE',  ( 20.12481660106788084, 9.526343992273943684, -8.226141669093042452 ) ) ;
#237265=PLANE ( 'NONE',  #191228 ) ;
#237283=ORIENTED_EDGE ( 'NONE', *, *, #175243, .F. ) ;
#237294=DIRECTION ( 'NONE',  ( 1.000000000000000000, -0.000000000000000000, -0.000000000000000000 ) ) ;
#237300=CIRCLE ( 'NONE', #258087, 0.1000000000000007133 ) ;
#237316=EDGE_LOOP ( 'NONE', ( #106212, #199836, #246761, #41096, #84418, #187866 ) ) ;
#237365=DIRECTION ( 'NONE',  ( 0.000000000000000000, -0.9915357197604860451, 0.1298341882519964408 ) ) ;
#237372=CARTESIAN_POINT ( 'NONE',  ( 21.09813707148777340, 6.385062105736502680, 0.03135149952951371555 ) ) ;
#237376=AXIS2_PLACEMENT_3D ( 'NONE', #228272, #130438, #49620 ) ;
#237410=CARTESIAN_POINT ( 'NONE',  ( 20.95203847575071521, 10.50106053927400751, -7.567071348623560567 ) ) ;
#237441=VERTEX_POINT ( 'NONE', #154718 ) ;
#237491=DIRECTION ( 'NONE',  ( 1.000000000000000000, -0.000000000000000000, -0.000000000000000000 ) ) ;
#237523=VECTOR ( 'NONE', #133025, 1000.000000000000000 ) ;
#237527=ORIENTED_EDGE ( 'NONE', *, *, #240695, .F. ) ;
#237559=DIRECTION ( 'NONE',  ( 0.000000000000000000, -1.000000000000000000, 0.000000000000000000 ) ) ;
#237579=EDGE_CURVE ( 'NONE', #162975, #157226, #160703, .T. ) ;
#237604=CYLINDRICAL_SURFACE ( 'NONE', #115817, 0.09999999999999939493 ) ;
#237608=EDGE_CURVE ( 'NONE', #206232, #171717, #255002, .T. ) ;
#237610=CARTESIAN_POINT ( 'NONE',  ( 20.94999999999999929, -1.164121893241208960, -41.41484808557160591 ) ) ;
#237621=VERTEX_POINT ( 'NONE', #239363 ) ;
#237647=CARTESIAN_POINT ( 'NONE',  ( 21.05000000000000071, -11.39257802170566691, -30.42605042016806394 ) ) ;
#237650=TOROIDAL_SURFACE ( 'NONE', #12815, 12.77499999999999858, 0.1000000000000000056 ) ;
#237662=CARTESIAN_POINT ( 'NONE',  ( 23.14999999999998437, 2.048861642965144398E-30, -4.049999999999998934 ) ) ;
#237665=CARTESIAN_POINT ( 'NONE',  ( 18.39999999999999858, -9.519327731092436906, -6.972976376559336664 ) ) ;
#237673=ORIENTED_EDGE ( 'NONE', *, *, #7862, .T. ) ;
#237697=AXIS2_PLACEMENT_3D ( 'NONE', #253089, #37932, #137003 ) ;
#237710=CARTESIAN_POINT ( 'NONE',  ( 21.14999999999999503, 0.000000000000000000, 0.000000000000000000 ) ) ;
#237737=CARTESIAN_POINT ( 'NONE',  ( 22.50000000000000000, 0.09999999999999939493, 11.75000000000000000 ) ) ;
#237805=EDGE_CURVE ( 'NONE', #206018, #29639, #98258, .T. ) ;
#237852=EDGE_CURVE ( 'NONE', #82492, #123641, #187944, .T. ) ;
#237863=DIRECTION ( 'NONE',  ( 0.000000000000000000, -0.4930308989875248349, -0.8700118002898312719 ) ) ;
#237887=B_SPLINE_CURVE_WITH_KNOTS ( 'NONE', 3,
 ( #136820, #33935, #192962, #132996, #75600, #195546, #92555, #134244, #11776, #16896, #194266, #71739, #131695, #74329, #55980, #233391 ),
 .UNSPECIFIED., .F., .F.,
 ( 4, 3, 3, 3, 3, 4 ),
 ( 0.000000000000000000, 2.209833635978076120E-05, 5.595056164119271882E-05, 8.979992002655370561E-05, 0.0001236482757198912198, 0.0001574984039362985287 ),
 .UNSPECIFIED. ) ;
#237923=DIRECTION ( 'NONE',  ( 0.000000000000000000, -1.000000000000000000, 0.000000000000000000 ) ) ;
#237950=ORIENTED_EDGE ( 'NONE', *, *, #250545, .F. ) ;
#238015=AXIS2_PLACEMENT_3D ( 'NONE', #121758, #164721, #219537 ) ;
#238037=CARTESIAN_POINT ( 'NONE',  ( -18.59999999999999787, -1.835341550224411922, -11.55515129256297868 ) ) ;
#238042=ORIENTED_EDGE ( 'NONE', *, *, #104138, .T. ) ;
#238060=DIRECTION ( 'NONE',  ( 1.000000000000000000, -0.000000000000000000, -0.000000000000000000 ) ) ;
#238062=CIRCLE ( 'NONE', #113182, 0.1000000000000028644 ) ;
#238095=DIRECTION ( 'NONE',  ( -0.000000000000000000, -1.897661533703519897E-16, 1.000000000000000000 ) ) ;
#238098=DIRECTION ( 'NONE',  ( 1.000000000000000000, -0.000000000000000000, 0.000000000000000000 ) ) ;
#238156=DIRECTION ( 'NONE',  ( 2.952720810173289112E-16, -1.000000000000000000, 0.000000000000000000 ) ) ;
#238159=ORIENTED_EDGE ( 'NONE', *, *, #202651, .F. ) ;
#238202=LINE ( 'NONE', #139076, #69862 ) ;
#238242=CARTESIAN_POINT ( 'NONE',  ( 18.54286124688533377, -9.623917578797810179, -40.24120233186267370 ) ) ;
#238252=CIRCLE ( 'NONE', #117645, 0.09999999999999939493 ) ;
#238261=LINE ( 'NONE', #80436, #15569 ) ;
#238285=EDGE_CURVE ( 'NONE', #196401, #159975, #252593, .T. ) ;
#238296=CARTESIAN_POINT ( 'NONE',  ( -18.59999999999999787, -1.249999999999999334, -41.30048075441507649 ) ) ;
#238306=AXIS2_PLACEMENT_3D ( 'NONE', #72933, #208579, #9071 ) ;
#238311=CARTESIAN_POINT ( 'NONE',  ( 22.59999954896768770, -0.008828232244170662948, 11.75050867406799604 ) ) ;
#238346=CARTESIAN_POINT ( 'NONE',  ( -21.14999999999999858, 11.74999999999999645, -6.783865662978151967 ) ) ;
#238363=AXIS2_PLACEMENT_3D ( 'NONE', #248376, #51422, #50158 ) ;
#238365=DIRECTION ( 'NONE',  ( 1.000000000000000000, 0.000000000000000000, -0.000000000000000000 ) ) ;
#238374=AXIS2_PLACEMENT_3D ( 'NONE', #178824, #242597, #220493 ) ;
#238397=CARTESIAN_POINT ( 'NONE',  ( 20.97239005616515328, 8.874843841350120499, -12.25015280215317048 ) ) ;
#238409=ORIENTED_EDGE ( 'NONE', *, *, #8531, .T. ) ;
#238412=CARTESIAN_POINT ( 'NONE',  ( -21.08078803292166725, 0.07918598715770600038, 6.333012964437140901 ) ) ;
#238423=AXIS2_PLACEMENT_3D ( 'NONE', #139840, #104229, #238967 ) ;
#238441=DIRECTION ( 'NONE',  ( 1.734723475976817507E-14, 0.000000000000000000, -1.000000000000000000 ) ) ;
#238444=ORIENTED_EDGE ( 'NONE', *, *, #45890, .T. ) ;
#238460=VERTEX_POINT ( 'NONE', #77228 ) ;
#238471=CARTESIAN_POINT ( 'NONE',  ( 20.95000000000000284, 11.60000000000000675, -26.57179676972450011 ) ) ;
#238473=DIRECTION ( 'NONE',  ( 0.000000000000000000, 0.000000000000000000, 1.000000000000000000 ) ) ;
#238475=DIRECTION ( 'NONE',  ( 0.000000000000000000, 1.040834085586079681E-14, -1.000000000000000000 ) ) ;
#238496=CARTESIAN_POINT ( 'NONE',  ( 20.12518398540832365, 9.975088720668688680, -7.996668252469905980 ) ) ;
#238509=DIRECTION ( 'NONE',  ( 1.000000000000000000, 0.000000000000000000, 0.000000000000000000 ) ) ;
#238531=DIRECTION ( 'NONE',  ( 0.000000000000000000, 0.000000000000000000, -1.000000000000000000 ) ) ;
#238538=EDGE_CURVE ( 'NONE', #220463, #107823, #254565, .T. ) ;
#238584=FACE_OUTER_BOUND ( 'NONE', #221035, .T. ) ;
#238595=CARTESIAN_POINT ( 'NONE',  ( -22.16821283564876666, 7.558973340780778649, 1.462253661542743006E-16 ) ) ;
#238621=DIRECTION ( 'NONE',  ( -2.952720810173289112E-16, 1.000000000000000000, -0.000000000000000000 ) ) ;
#238629=CARTESIAN_POINT ( 'NONE',  ( 20.94999999999999574, 10.62357026048281128, -7.491945203230555350 ) ) ;
#238637=CARTESIAN_POINT ( 'NONE',  ( 20.85000000000000142, 11.65000000000000391, -33.50000000000000000 ) ) ;
#238736=AXIS2_PLACEMENT_3D ( 'NONE', #171425, #130975, #210516 ) ;
#238764=ORIENTED_EDGE ( 'NONE', *, *, #157772, .T. ) ;
#238776=CYLINDRICAL_SURFACE ( 'NONE', #27955, 11.80000000000000249 ) ;
#238789=DIRECTION ( 'NONE',  ( 0.000000000000000000, 0.1495327102803689356, 0.9887567792719336168 ) ) ;
#238840=PLANE ( 'NONE',  #184678 ) ;
#238856=VECTOR ( 'NONE', #21552, 1000.000000000000000 ) ;
#238878=EDGE_CURVE ( 'NONE', #141594, #143109, #97755, .T. ) ;
#238880=DIRECTION ( 'NONE',  ( -1.000000000000000000, 0.000000000000000000, 0.000000000000000000 ) ) ;
#238887=CARTESIAN_POINT ( 'NONE',  ( 21.14999999999999858, 8.786607556600111835, -12.25000000000000000 ) ) ;
#238908=CARTESIAN_POINT ( 'NONE',  ( 22.59999985501178799, 11.74986979300298806, 0.06559866979947076571 ) ) ;
#238912=ORIENTED_EDGE ( 'NONE', *, *, #67476, .F. ) ;
#238919=ORIENTED_EDGE ( 'NONE', *, *, #113697, .T. ) ;
#238935=ADVANCED_FACE ( 'NONE', ( #156516 ), #152658, .F. ) ;
#238948=ADVANCED_FACE ( 'NONE', ( #173528 ), #194349, .F. ) ;
#238957=CARTESIAN_POINT ( 'NONE',  ( 18.52130828395271678, -9.481395502625792560, -7.024506723883644277 ) ) ;
#238967=DIRECTION ( 'NONE',  ( 0.000000000000000000, 0.000000000000000000, 1.000000000000000000 ) ) ;
#239006=ORIENTED_EDGE ( 'NONE', *, *, #137930, .T. ) ;
#239029=EDGE_LOOP ( 'NONE', ( #88924, #11554, #250297, #171359 ) ) ;
#239042=AXIS2_PLACEMENT_3D ( 'NONE', #44052, #21931, #183568 ) ;
#239053=AXIS2_PLACEMENT_3D ( 'NONE', #120807, #4660, #67220 ) ;
#239073=ORIENTED_EDGE ( 'NONE', *, *, #78700, .T. ) ;
#239076=DIRECTION ( 'NONE',  ( 0.000000000000000000, 0.000000000000000000, 1.000000000000000000 ) ) ;
#239077=CIRCLE ( 'NONE', #168387, 0.1000000000000002554 ) ;
#239139=CARTESIAN_POINT ( 'NONE',  ( 20.84999999999999432, 7.021664781900089913, -37.33356540189728889 ) ) ;
#239153=EDGE_CURVE ( 'NONE', #26218, #185478, #90637, .T. ) ;
#239230=VERTEX_POINT ( 'NONE', #134025 ) ;
#239243=EDGE_CURVE ( 'NONE', #11085, #256624, #186352, .T. ) ;
#239267=ADVANCED_FACE ( 'NONE', ( #191478 ), #236404, .T. ) ;
#239295=CARTESIAN_POINT ( 'NONE',  ( -21.05000000000000071, -11.64999999999999858, -30.59999999999999432 ) ) ;
#239317=VERTEX_POINT ( 'NONE', #15391 ) ;
#239332=EDGE_LOOP ( 'NONE', ( #29265, #163119, #68465, #31245 ) ) ;
#239335=DIRECTION ( 'NONE',  ( -0.000000000000000000, 0.000000000000000000, 1.000000000000000000 ) ) ;
#239356=ADVANCED_FACE ( 'NONE', ( #102576 ), #200429, .F. ) ;
#239363=CARTESIAN_POINT ( 'NONE',  ( 23.24999999999999289, 6.450000000000001066, -12.35000000000000320 ) ) ;
#239423=VECTOR ( 'NONE', #257063, 1000.000000000000000 ) ;
#239435=DIRECTION ( 'NONE',  ( 0.000000000000000000, 0.000000000000000000, -1.000000000000000000 ) ) ;
#239454=ORIENTED_EDGE ( 'NONE', *, *, #121864, .T. ) ;
#239464=CIRCLE ( 'NONE', #68767, 0.1000000000000002554 ) ;
#239479=CARTESIAN_POINT ( 'NONE',  ( -23.25000000000000000, 11.65000000000000036, -12.15000000000000036 ) ) ;
#239484=CARTESIAN_POINT ( 'NONE',  ( 23.14999999999999503, 11.65000000000000746, -26.48519422934606027 ) ) ;
#239500=ORIENTED_EDGE ( 'NONE', *, *, #126743, .T. ) ;
#239503=ORIENTED_EDGE ( 'NONE', *, *, #113180, .F. ) ;
#239519=DIRECTION ( 'NONE',  ( -1.000000000000000000, 0.000000000000000000, 0.000000000000000000 ) ) ;
#239545=EDGE_CURVE ( 'NONE', #191355, #239696, #107410, .T. ) ;
#239554=DIRECTION ( 'NONE',  ( -1.000000000000000000, -3.265361837132813093E-16, 0.000000000000000000 ) ) ;
#239593=VECTOR ( 'NONE', #95075, 1000.000000000000000 ) ;
#239599=CARTESIAN_POINT ( 'NONE',  ( 21.07954640115340439, 0.06600770713963947933, 6.329287696024268328 ) ) ;
#239604=DIRECTION ( 'NONE',  ( 0.000000000000000000, 1.000000000000000000, 0.000000000000000000 ) ) ;
#239613=CARTESIAN_POINT ( 'NONE',  ( 22.45463910399148233, -8.887310749685707770E-13, 11.64957081018417639 ) ) ;
#239614=DIRECTION ( 'NONE',  ( 0.000000000000000000, 0.000000000000000000, 1.000000000000000000 ) ) ;
#239652=VERTEX_POINT ( 'NONE', #58977 ) ;
#239656=DIRECTION ( 'NONE',  ( 0.000000000000000000, -0.000000000000000000, 1.000000000000000000 ) ) ;
#239670=CIRCLE ( 'NONE', #127245, 0.09999999999999939493 ) ;
#239672=FACE_OUTER_BOUND ( 'NONE', #190332, .T. ) ;
#239676=DIRECTION ( 'NONE',  ( -1.000000000000000000, 0.000000000000000000, 0.000000000000000000 ) ) ;
#239685=CARTESIAN_POINT ( 'NONE',  ( -20.94999999999999929, 0.000000000000000000, -33.50000000000000000 ) ) ;
#239696=VERTEX_POINT ( 'NONE', #198518 ) ;
#239712=DIRECTION ( 'NONE',  ( 0.000000000000000000, 2.891205793294679805E-16, -1.000000000000000000 ) ) ;
#239713=AXIS2_PLACEMENT_3D ( 'NONE', #31668, #189435, #90307 ) ;
#239752=DIRECTION ( 'NONE',  ( -1.000000000000000000, -0.000000000000000000, -0.000000000000000000 ) ) ;
#239768=LINE ( 'NONE', #139353, #184937 ) ;
#239791=FACE_OUTER_BOUND ( 'NONE', #65547, .T. ) ;
#239792=ADVANCED_FACE ( 'NONE', ( #65423 ), #101955, .F. ) ;
#239829=DIRECTION ( 'NONE',  ( 0.000000000000000000, 0.000000000000000000, 1.000000000000000000 ) ) ;
#239845=DIRECTION ( 'NONE',  ( -0.000000000000000000, -0.000000000000000000, 1.000000000000000000 ) ) ;
#239854=FACE_OUTER_BOUND ( 'NONE', #195961, .T. ) ;
#239855=EDGE_CURVE ( 'NONE', #62691, #150108, #209260, .T. ) ;
#239880=CARTESIAN_POINT ( 'NONE',  ( 21.93340585971863632, 7.324147022855297173, -1.277737337956073836E-15 ) ) ;
#239888=EDGE_CURVE ( 'NONE', #217291, #84692, #91419, .T. ) ;
#239901=DIRECTION ( 'NONE',  ( -3.265361837132813093E-16, 1.000000000000000000, 0.000000000000000000 ) ) ;
#239910=B_SPLINE_CURVE_WITH_KNOTS ( 'NONE', 3,
 ( #145256, #142685, #87841, #188252, #46165, #167432 ),
 .UNSPECIFIED., .F., .F.,
 ( 4, 2, 4 ),
 ( 1.138412281109779656E-18, 0.0001569047307838639788, 0.0003138094615677267650 ),
 .UNSPECIFIED. ) ;
#239960=DIRECTION ( 'NONE',  ( 0.000000000000000000, 0.000000000000000000, 1.000000000000000000 ) ) ;
#239961=VERTEX_POINT ( 'NONE', #256843 ) ;
#240042=VERTEX_POINT ( 'NONE', #19587 ) ;
#240060=ORIENTED_EDGE ( 'NONE', *, *, #10518, .F. ) ;
#240071=ORIENTED_EDGE ( 'NONE', *, *, #31781, .F. ) ;
#240073=ORIENTED_EDGE ( 'NONE', *, *, #51529, .F. ) ;
#240088=EDGE_CURVE ( 'NONE', #32767, #70529, #178685, .T. ) ;
#240114=CARTESIAN_POINT ( 'NONE',  ( -20.54999999999999716, -9.400000000000002132, -23.60603087734756045 ) ) ;
#240122=DIRECTION ( 'NONE',  ( 0.000000000000000000, 1.776356839400250465E-15, -1.000000000000000000 ) ) ;
#240131=CARTESIAN_POINT ( 'NONE',  ( 23.14999999999999503, 6.649999999999999467, -12.25000000000000000 ) ) ;
#240132=CARTESIAN_POINT ( 'NONE',  ( 18.49999999999998934, 6.550000000000000711, -21.25000000000000000 ) ) ;
#240138=EDGE_LOOP ( 'NONE', ( #83683, #24036, #243129, #83165 ) ) ;
#240152=AXIS2_PLACEMENT_3D ( 'NONE', #228862, #249708, #211881 ) ;
#240172=VERTEX_POINT ( 'NONE', #140808 ) ;
#240190=CARTESIAN_POINT ( 'NONE',  ( 20.95512820512820440, 10.62384868371188062, -12.15000000000000036 ) ) ;
#240197=EDGE_LOOP ( 'NONE', ( #244582, #132262, #44994, #146745 ) ) ;
#240204=ORIENTED_EDGE ( 'NONE', *, *, #65192, .T. ) ;
#240218=DIRECTION ( 'NONE',  ( 0.000000000000000000, 0.000000000000000000, 1.000000000000000000 ) ) ;
#240260=AXIS2_PLACEMENT_3D ( 'NONE', #23973, #44802, #124342 ) ;
#240272=VECTOR ( 'NONE', #94840, 1000.000000000000000 ) ;
#240282=CARTESIAN_POINT ( 'NONE',  ( -23.15000000000000213, 1.999999999999998224, -20.27537807723789953 ) ) ;
#240291=DIRECTION ( 'NONE',  ( 0.000000000000000000, 0.000000000000000000, 1.000000000000000000 ) ) ;
#240298=DIRECTION ( 'NONE',  ( 0.7071067811865474617, 0.7071067811865474617, 0.000000000000000000 ) ) ;
#240300=ORIENTED_EDGE ( 'NONE', *, *, #5406, .T. ) ;
#240318=CIRCLE ( 'NONE', #244398, 0.1000000000000007133 ) ;
#240325=CARTESIAN_POINT ( 'NONE',  ( -20.64999999999999858, 0.000000000000000000, -35.40000000000000568 ) ) ;
#240342=DIRECTION ( 'NONE',  ( -2.940209281316621016E-16, 1.000000000000000000, -8.881784197001251337E-16 ) ) ;
#240366=CARTESIAN_POINT ( 'NONE',  ( 23.24999999999999289, 11.75000000000000711, -0.1000000000000028644 ) ) ;
#240373=EDGE_CURVE ( 'NONE', #183417, #247150, #174475, .T. ) ;
#240412=ORIENTED_EDGE ( 'NONE', *, *, #156333, .F. ) ;
#240422=CARTESIAN_POINT ( 'NONE',  ( -18.50000972452446035, 10.29326151434210779, -38.95928225104149334 ) ) ;
#240433=CARTESIAN_POINT ( 'NONE',  ( -21.05315837394252654, 11.74999999999999289, -26.65835600069834399 ) ) ;
#240458=DIRECTION ( 'NONE',  ( 1.000000000000000000, 0.000000000000000000, 0.000000000000000000 ) ) ;
#240468=DIRECTION ( 'NONE',  ( 0.000000000000000000, 0.1298341882520022694, 0.9915357197604852679 ) ) ;
#240496=DIRECTION ( 'NONE',  ( 0.000000000000000000, -1.000000000000000000, 0.000000000000000000 ) ) ;
#240501=DIRECTION ( 'NONE',  ( -4.408576920032448588E-17, 0.1350103645451876666, 0.9908441862701600211 ) ) ;
#240523=EDGE_CURVE ( 'NONE', #190309, #53632, #140714, .T. ) ;
#240552=VECTOR ( 'NONE', #155737, 1000.000000000000000 ) ;
#240573=CARTESIAN_POINT ( 'NONE',  ( 21.05000000000000071, -9.500000000000001776, -9.893969122652443104 ) ) ;
#240585=ORIENTED_EDGE ( 'NONE', *, *, #7527, .F. ) ;
#240586=CARTESIAN_POINT ( 'NONE',  ( 18.49999999999999645, 1.736257131597397585, -11.56865232901749962 ) ) ;
#240598=AXIS2_PLACEMENT_3D ( 'NONE', #94873, #251386, #12806 ) ;
#240613=LINE ( 'NONE', #119390, #114935 ) ;
#240614=DIRECTION ( 'NONE',  ( -0.000000000000000000, -0.000000000000000000, -1.000000000000000000 ) ) ;
#240638=EDGE_LOOP ( 'NONE', ( #108425, #85511, #135641, #88499 ) ) ;
#240659=LINE ( 'NONE', #221083, #44399 ) ;
#240665=EDGE_LOOP ( 'NONE', ( #140508, #177153, #205963, #218588 ) ) ;
#240669=ORIENTED_EDGE ( 'NONE', *, *, #141896, .F. ) ;
#240672=CARTESIAN_POINT ( 'NONE',  ( 23.15000000000000213, -8.596261682242991142, -9.450127517150276546 ) ) ;
#240675=FACE_OUTER_BOUND ( 'NONE', #192582, .T. ) ;
#240695=EDGE_CURVE ( 'NONE', #239961, #153115, #68665, .T. ) ;
#240707=FACE_OUTER_BOUND ( 'NONE', #123067, .T. ) ;
#240725=CIRCLE ( 'NONE', #111546, 0.1000000000000000472 ) ;
#240760=ORIENTED_EDGE ( 'NONE', *, *, #245725, .F. ) ;
#240786=LINE ( 'NONE', #142936, #165611 ) ;
#240814=CARTESIAN_POINT ( 'NONE',  ( -22.39999999999999858, -1.124330358361676913E-15, 11.75043289245860834 ) ) ;
#240838=EDGE_LOOP ( 'NONE', ( #132763, #201505, #92470, #124200, #46595, #31205, #100422 ) ) ;
#240858=AXIS2_PLACEMENT_3D ( 'NONE', #76056, #173929, #53930 ) ;
#240865=EDGE_CURVE ( 'NONE', #191917, #108350, #161044, .T. ) ;
#240919=EDGE_CURVE ( 'NONE', #47980, #239317, #111503, .T. ) ;
#240969=VERTEX_POINT ( 'NONE', #22835 ) ;
#240984=DIRECTION ( 'NONE',  ( 1.000000000000000000, -0.000000000000000000, -0.000000000000000000 ) ) ;
#240995=DIRECTION ( 'NONE',  ( -0.000000000000000000, -2.891205793294679805E-16, 1.000000000000000000 ) ) ;
#241010=CARTESIAN_POINT ( 'NONE',  ( -21.46681500593124170, 6.857511159386057820, -9.855405879761855605E-16 ) ) ;
#241011=VERTEX_POINT ( 'NONE', #129620 ) ;
#241022=ORIENTED_EDGE ( 'NONE', *, *, #151680, .T. ) ;
#241040=EDGE_LOOP ( 'NONE', ( #243563, #202368, #58194, #5012 ) ) ;
#241042=CARTESIAN_POINT ( 'NONE',  ( -20.94999999999999929, 0.000000000000000000, -21.70000000000000284 ) ) ;
#241044=EDGE_CURVE ( 'NONE', #11322, #26951, #170075, .T. ) ;
#241056=EDGE_LOOP ( 'NONE', ( #215572, #98311, #147619, #155824 ) ) ;
#241078=ORIENTED_EDGE ( 'NONE', *, *, #154731, .T. ) ;
#241099=DIRECTION ( 'NONE',  ( -1.000000000000000000, -2.952720810173289112E-16, 0.000000000000000000 ) ) ;
#241105=AXIS2_PLACEMENT_3D ( 'NONE', #244988, #3815, #123769 ) ;
#241108=ORIENTED_EDGE ( 'NONE', *, *, #225795, .T. ) ;
#241123=FACE_OUTER_BOUND ( 'NONE', #115584, .T. ) ;
#241124=DIRECTION ( 'NONE',  ( 0.000000000000000000, -1.000000000000000000, 0.000000000000000000 ) ) ;
#241130=EDGE_CURVE ( 'NONE', #11112, #138031, #28523, .T. ) ;
#241151=ORIENTED_EDGE ( 'NONE', *, *, #239888, .F. ) ;
#241174=AXIS2_PLACEMENT_3D ( 'NONE', #214840, #16665, #15383 ) ;
#241183=EDGE_CURVE ( 'NONE', #147515, #80105, #215878, .T. ) ;
#241196=EDGE_CURVE ( 'NONE', #153115, #199045, #134729, .T. ) ;
#241197=ORIENTED_EDGE ( 'NONE', *, *, #14804, .T. ) ;
#241216=CARTESIAN_POINT ( 'NONE',  ( -18.59999999999999787, -9.399999999999943512, -7.297259759663287326 ) ) ;
#241219=EDGE_LOOP ( 'NONE', ( #111606, #170200, #43064, #15979 ) ) ;
#241298=EDGE_CURVE ( 'NONE', #95630, #4734, #199358, .T. ) ;
#241340=ORIENTED_EDGE ( 'NONE', *, *, #35575, .T. ) ;
#241358=TOROIDAL_SURFACE ( 'NONE', #62276, 11.65000000000000036, 0.1000000000000000056 ) ;
#241361=ORIENTED_EDGE ( 'NONE', *, *, #211364, .F. ) ;
#241380=EDGE_LOOP ( 'NONE', ( #31644, #119693, #195008, #167187 ) ) ;
#241428=LINE ( 'NONE', #164458, #113033 ) ;
#241450=CARTESIAN_POINT ( 'NONE',  ( 21.05000000000000071, 4.999999999999997335, -12.40526601891309788 ) ) ;
#241458=ORIENTED_EDGE ( 'NONE', *, *, #8801, .T. ) ;
#241513=VERTEX_POINT ( 'NONE', #51995 ) ;
#241551=DIRECTION ( 'NONE',  ( -1.000000000000000000, -0.000000000000000000, 0.000000000000000000 ) ) ;
#241587=EDGE_CURVE ( 'NONE', #113100, #16494, #146799, .T. ) ;
#241607=AXIS2_PLACEMENT_3D ( 'NONE', #132018, #12100, #138106 ) ;
#241620=FACE_OUTER_BOUND ( 'NONE', #1562, .T. ) ;
#241622=EDGE_CURVE ( 'NONE', #243446, #11085, #174454, .T. ) ;
#241623=ORIENTED_EDGE ( 'NONE', *, *, #120739, .F. ) ;
#241629=ORIENTED_EDGE ( 'NONE', *, *, #80195, .T. ) ;
#241661=CYLINDRICAL_SURFACE ( 'NONE', #184324, 4.000000000000000000 ) ;
#241669=ORIENTED_EDGE ( 'NONE', *, *, #75383, .F. ) ;
#241690=DIRECTION ( 'NONE',  ( -0.000000000000000000, 1.000000000000000000, 1.734723475976807292E-15 ) ) ;
#241705=CARTESIAN_POINT ( 'NONE',  ( -18.50016250449483479, 10.29766095124169922, -38.97436639332758546 ) ) ;
#241708=ORIENTED_EDGE ( 'NONE', *, *, #230905, .F. ) ;
#241714=CARTESIAN_POINT ( 'NONE',  ( -20.94999999999999929, 11.63687328910415886, -26.67824078667520382 ) ) ;
#241718=AXIS2_PLACEMENT_3D ( 'NONE', #88765, #126630, #11849 ) ;
#241753=CARTESIAN_POINT ( 'NONE',  ( -23.25000000000000000, 10.33248238082518711, -39.09484654391314962 ) ) ;
#241760=EDGE_LOOP ( 'NONE', ( #123104, #31066, #222675, #249474 ) ) ;
#241846=CARTESIAN_POINT ( 'NONE',  ( -22.50000000000000000, 0.000000000000000000, 0.1000000000000028644 ) ) ;
#241868=CYLINDRICAL_SURFACE ( 'NONE', #63796, 12.87500000000000000 ) ;
#241872=AXIS2_PLACEMENT_3D ( 'NONE', #30838, #253695, #212034 ) ;
#241902=FACE_OUTER_BOUND ( 'NONE', #172417, .T. ) ;
#241912=CIRCLE ( 'NONE', #146057, 0.5000000000000004441 ) ;
#241934=DIRECTION ( 'NONE',  ( 1.000000000000000000, 0.000000000000000000, 0.000000000000000000 ) ) ;
#241940=ORIENTED_EDGE ( 'NONE', *, *, #53180, .F. ) ;
#241989=VERTEX_POINT ( 'NONE', #40747 ) ;
#241991=ORIENTED_EDGE ( 'NONE', *, *, #92792, .F. ) ;
#241992=CARTESIAN_POINT ( 'NONE',  ( -18.59999999999999787, 6.933893972126341509, -37.28564583437357527 ) ) ;
#242069=DIRECTION ( 'NONE',  ( 0.000000000000000000, 0.000000000000000000, -1.000000000000000000 ) ) ;
#242071=CARTESIAN_POINT ( 'NONE',  ( -20.85000000000000142, 11.64999999999999680, -33.50000000000000000 ) ) ;
#242092=AXIS2_PLACEMENT_3D ( 'NONE', #250147, #10260, #29843 ) ;
#242109=CARTESIAN_POINT ( 'NONE',  ( 21.05000000000000071, 0.06570161032208717000, 6.258316057332036664 ) ) ;
#242171=ADVANCED_FACE ( 'NONE', ( #82367 ), #204900, .T. ) ;
#242179=ORIENTED_EDGE ( 'NONE', *, *, #241130, .T. ) ;
#242184=ORIENTED_EDGE ( 'NONE', *, *, #200877, .F. ) ;
#242196=CARTESIAN_POINT ( 'NONE',  ( -20.64999999999999858, 0.000000000000000000, -33.50000000000000000 ) ) ;
#242214=CARTESIAN_POINT ( 'NONE',  ( 21.05000000000000071, -9.000000000000000000, -23.60603087734755690 ) ) ;
#242230=DIRECTION ( 'NONE',  ( 0.000000000000000000, 0.000000000000000000, -1.000000000000000000 ) ) ;
#242243=ORIENTED_EDGE ( 'NONE', *, *, #229146, .T. ) ;
#242279=PLANE ( 'NONE',  #136294 ) ;
#242293=LINE ( 'NONE', #66240, #15866 ) ;
#242300=DIRECTION ( 'NONE',  ( -0.000000000000000000, -1.000000000000000000, -5.421010862427649374E-16 ) ) ;
#242354=CARTESIAN_POINT ( 'NONE',  ( 23.14999999999999858, 11.65000000000000746, -26.48519422934606027 ) ) ;
#242364=DIRECTION ( 'NONE',  ( -0.000000000000000000, -0.000000000000000000, -1.000000000000000000 ) ) ;
#242369=DIRECTION ( 'NONE',  ( 0.000000000000000000, 0.000000000000000000, 1.000000000000000000 ) ) ;
#242388=CARTESIAN_POINT ( 'NONE',  ( 23.15000000000000213, -9.000000000000001776, -9.893969122652443104 ) ) ;
#242389=DIRECTION ( 'NONE',  ( 1.000000000000000000, 0.000000000000000000, 0.000000000000000000 ) ) ;
#242406=CARTESIAN_POINT ( 'NONE',  ( 20.94999999999999929, 7.120270961697594103, -37.15956304183931991 ) ) ;
#242449=EDGE_CURVE ( 'NONE', #129511, #33930, #18271, .T. ) ;
#242511=ORIENTED_EDGE ( 'NONE', *, *, #178167, .T. ) ;
#242536=VERTEX_POINT ( 'NONE', #25983 ) ;
#242551=ADVANCED_FACE ( 'NONE', ( #145905 ), #144618, .F. ) ;
#242565=CARTESIAN_POINT ( 'NONE',  ( -23.25000000000000000, -9.000000000000003553, -9.893969122652444881 ) ) ;
#242597=DIRECTION ( 'NONE',  ( 4.026293107431335996E-15, -0.8700118002898359348, 0.4930308989875165082 ) ) ;
#242623=CARTESIAN_POINT ( 'NONE',  ( 20.94999999999999929, -1.362429037193307435, -41.38888124792119783 ) ) ;
#242636=AXIS2_PLACEMENT_3D ( 'NONE', #16101, #173913, #249564 ) ;
#242644=CIRCLE ( 'NONE', #130203, 0.09999999999999996392 ) ;
#242646=CARTESIAN_POINT ( 'NONE',  ( -20.00857864376270001, 9.150000000000002132, -21.15000000000000213 ) ) ;
#242660=CARTESIAN_POINT ( 'NONE',  ( 18.41356215285960829, -9.500000000000023093, -7.032069396699602848 ) ) ;
#242661=AXIS2_PLACEMENT_3D ( 'NONE', #69028, #208537, #205947 ) ;
#242705=CARTESIAN_POINT ( 'NONE',  ( 21.09610168723073187, 0.03358950689149224622, 6.378955715224786438 ) ) ;
#242711=CARTESIAN_POINT ( 'NONE',  ( -21.05000000000000071, 1.162701749938009677, -8.000000000000000000 ) ) ;
#242725=DIRECTION ( 'NONE',  ( -1.000000000000000000, 0.000000000000000000, 0.000000000000000000 ) ) ;
#242799=AXIS2_PLACEMENT_3D ( 'NONE', #81376, #572, #159679 ) ;
#242833=EDGE_CURVE ( 'NONE', #1674, #237441, #212569, .T. ) ;
#242845=AXIS2_PLACEMENT_3D ( 'NONE', #87050, #84457, #208329 ) ;
#242875=VERTEX_POINT ( 'NONE', #80453 ) ;
#242879=VERTEX_POINT ( 'NONE', #216146 ) ;
#242896=CARTESIAN_POINT ( 'NONE',  ( 23.14999999999999858, 0.000000000000000000, -33.50000000000000000 ) ) ;
#242926=EDGE_CURVE ( 'NONE', #96700, #156221, #137686, .T. ) ;
#242933=FACE_OUTER_BOUND ( 'NONE', #38243, .T. ) ;
#242951=VECTOR ( 'NONE', #159535, 1000.000000000000000 ) ;
#242960=DIRECTION ( 'NONE',  ( 0.000000000000000000, 0.000000000000000000, -1.000000000000000000 ) ) ;
#242961=CARTESIAN_POINT ( 'NONE',  ( -20.64999999999999858, 4.349999999999999645, -12.35000000000000142 ) ) ;
#242979=CARTESIAN_POINT ( 'NONE',  ( -23.25000000000000000, 4.150000000000001243, -21.25000000000000000 ) ) ;
#242986=FACE_OUTER_BOUND ( 'NONE', #16631, .T. ) ;
#242994=TOROIDAL_SURFACE ( 'NONE', #51436, 11.65000000000000036, 0.1000000000000000056 ) ;
#243007=ORIENTED_EDGE ( 'NONE', *, *, #135744, .F. ) ;
#243042=CIRCLE ( 'NONE', #251431, 0.09999999999999939493 ) ;
#243076=DIRECTION ( 'NONE',  ( 0.000000000000000000, 2.664535259100375697E-15, -1.000000000000000000 ) ) ;
#243079=CARTESIAN_POINT ( 'NONE',  ( 21.05000000000000071, 0.000000000000000000, -30.59999999999999432 ) ) ;
#243093=ORIENTED_EDGE ( 'NONE', *, *, #156202, .T. ) ;
#243099=CARTESIAN_POINT ( 'NONE',  ( -20.85000000000000142, 11.64999999999999680, -26.71613433702190576 ) ) ;
#243103=VERTEX_POINT ( 'NONE', #231572 ) ;
#243129=ORIENTED_EDGE ( 'NONE', *, *, #123212, .T. ) ;
#243151=TOROIDAL_SURFACE ( 'NONE', #147482, 6.258578643762700899, 0.1000000000000000056 ) ;
#243200=CIRCLE ( 'NONE', #189052, 0.09999999999999939493 ) ;
#243217=AXIS2_PLACEMENT_3D ( 'NONE', #149953, #226895, #110797 ) ;
#243284=EDGE_CURVE ( 'NONE', #161574, #249634, #108672, .T. ) ;
#243289=DIRECTION ( 'NONE',  ( 0.000000000000000000, 0.000000000000000000, -1.000000000000000000 ) ) ;
#243301=AXIS2_PLACEMENT_3D ( 'NONE', #253783, #73917, #214667 ) ;
#243317=DIRECTION ( 'NONE',  ( 1.000000000000000000, 0.000000000000000000, 0.000000000000000000 ) ) ;
#243323=EDGE_CURVE ( 'NONE', #129511, #204776, #118030, .T. ) ;
#243332=ORIENTED_EDGE ( 'NONE', *, *, #203063, .T. ) ;
#243333=ADVANCED_FACE ( 'NONE', ( #236681 ), #116746, .T. ) ;
#243377=CARTESIAN_POINT ( 'NONE',  ( 22.48970261584622321, 11.65000000000000036, 0.05536948821740608068 ) ) ;
#243378=TOROIDAL_SURFACE ( 'NONE', #72726, 7.791421356237335338, 0.1000000000000000056 ) ;
#243408=AXIS2_PLACEMENT_3D ( 'NONE', #156383, #132949, #138049 ) ;
#243416=DIRECTION ( 'NONE',  ( 1.000000000000000000, -0.000000000000000000, -0.000000000000000000 ) ) ;
#243446=VERTEX_POINT ( 'NONE', #128323 ) ;
#243457=LINE ( 'NONE', #3557, #4954 ) ;
#243468=AXIS2_PLACEMENT_3D ( 'NONE', #113569, #50995, #30201 ) ;
#243499=ORIENTED_EDGE ( 'NONE', *, *, #20235, .T. ) ;
#243508=ORIENTED_EDGE ( 'NONE', *, *, #252643, .F. ) ;
#243511=AXIS2_PLACEMENT_3D ( 'NONE', #111905, #53193, #132755 ) ;
#243519=CARTESIAN_POINT ( 'NONE',  ( 23.14999999999999858, 5.499999999999998224, -21.09473398108690390 ) ) ;
#243525=CIRCLE ( 'NONE', #255949, 0.09999999999999999167 ) ;
#243527=ADVANCED_FACE ( 'NONE', ( #70937, #185723 ), #150460, .T. ) ;
#243556=VECTOR ( 'NONE', #7111, 1000.000000000000000 ) ;
#243563=ORIENTED_EDGE ( 'NONE', *, *, #108228, .T. ) ;
#243583=CARTESIAN_POINT ( 'NONE',  ( -21.55000000000000071, 7.349999999999998757, -21.15000000000000213 ) ) ;
#243615=ORIENTED_EDGE ( 'NONE', *, *, #19359, .F. ) ;
#243625=AXIS2_PLACEMENT_3D ( 'NONE', #24707, #3830, #82043 ) ;
#243649=ORIENTED_EDGE ( 'NONE', *, *, #257768, .T. ) ;
#243657=DIRECTION ( 'NONE',  ( 0.000000000000000000, 0.000000000000000000, -1.000000000000000000 ) ) ;
#243658=ORIENTED_EDGE ( 'NONE', *, *, #85522, .T. ) ;
#243687=CIRCLE ( 'NONE', #193800, 0.09999999999999939493 ) ;
#243708=AXIS2_PLACEMENT_3D ( 'NONE', #49829, #125519, #205027 ) ;
#243717=LINE ( 'NONE', #126332, #19471 ) ;
#243719=DIRECTION ( 'NONE',  ( 0.000000000000000000, -0.4999999999999799605, 0.8660254037844502539 ) ) ;
#243729=ORIENTED_EDGE ( 'NONE', *, *, #14375, .T. ) ;
#243763=CYLINDRICAL_SURFACE ( 'NONE', #244734, 11.80000000000000426 ) ;
#243771=VERTEX_POINT ( 'NONE', #105510 ) ;
#243777=CARTESIAN_POINT ( 'NONE',  ( -22.57320508075687115, 11.75000000000000000, 0.000000000000000000 ) ) ;
#243784=EDGE_CURVE ( 'NONE', #88943, #211780, #250501, .T. ) ;
#243786=VERTEX_POINT ( 'NONE', #221619 ) ;
#243825=DIRECTION ( 'NONE',  ( 1.000000000000000000, 0.000000000000000000, 0.000000000000000000 ) ) ;
#243847=CARTESIAN_POINT ( 'NONE',  ( -21.40925344232282512, 6.658518859390450295, 0.09895018861964700874 ) ) ;
#243848=ORIENTED_EDGE ( 'NONE', *, *, #65909, .T. ) ;
#243852=VERTEX_POINT ( 'NONE', #113248 ) ;
#243864=ADVANCED_FACE ( 'NONE', ( #229360 ), #183873, .T. ) ;
#243870=DIRECTION ( 'NONE',  ( 0.000000000000000000, 0.000000000000000000, -1.000000000000000000 ) ) ;
#243891=CIRCLE ( 'NONE', #89950, 7.791421356237335338 ) ;
#243911=CARTESIAN_POINT ( 'NONE',  ( -20.94999999999999929, 6.846123162352588665, -37.23772626684986164 ) ) ;
#243912=DIRECTION ( 'NONE',  ( -0.000000000000000000, -1.000000000000000000, -0.000000000000000000 ) ) ;
#243913=CARTESIAN_POINT ( 'NONE',  ( -23.15000000000000213, 1.999999999999998224, -12.72462192276209869 ) ) ;
#243918=CYLINDRICAL_SURFACE ( 'NONE', #28546, 0.09999999999999939493 ) ;
#243926=ADVANCED_FACE ( 'NONE', ( #254029 ), #138063, .T. ) ;
#243963=CARTESIAN_POINT ( 'NONE',  ( -18.59999999999999787, 0.000000000000000000, 0.000000000000000000 ) ) ;
#243969=ADVANCED_FACE ( 'NONE', ( #55803 ), #121547, .T. ) ;
#243973=TOROIDAL_SURFACE ( 'NONE', #144001, 11.70000000000000107, 0.1000000000000000056 ) ;
#244016=AXIS2_PLACEMENT_3D ( 'NONE', #214604, #236728, #213317 ) ;
#244020=CYLINDRICAL_SURFACE ( 'NONE', #81536, 0.09999999999999939493 ) ;
#244022=FACE_OUTER_BOUND ( 'NONE', #181481, .T. ) ;
#244038=DIRECTION ( 'NONE',  ( 0.000000000000000000, 1.000000000000000000, 2.891205793294679805E-16 ) ) ;
#244052=CIRCLE ( 'NONE', #31719, 0.09999999999999939493 ) ;
#244065=DIRECTION ( 'NONE',  ( 1.000000000000000000, 0.000000000000000000, -0.000000000000000000 ) ) ;
#244077=LINE ( 'NONE', #159432, #60515 ) ;
#244082=CARTESIAN_POINT ( 'NONE',  ( -20.93975676684922504, 10.31104185822947450, -39.02045169831057336 ) ) ;
#244090=FACE_OUTER_BOUND ( 'NONE', #113266, .T. ) ;
#244091=B_SPLINE_CURVE_WITH_KNOTS ( 'NONE', 3,
 ( #57900, #98289, #192305, #235262, #137437, #55315, #216975, #78749, #56598, #38365, #214416, #35814, #117885, #197422, #18784, #158342 ),
 .UNSPECIFIED., .F., .F.,
 ( 4, 3, 3, 3, 3, 4 ),
 ( 0.000000000000000000, 3.357088238233517998E-05, 6.714213034887110308E-05, 0.0001007408646120942151, 0.0001343627955914231033, 0.0001573956632896011476 ),
 .UNSPECIFIED. ) ;
#244099=CIRCLE ( 'NONE', #131687, 0.1000000000000017958 ) ;
#244117=LINE ( 'NONE', #65483, #192816 ) ;
#244142=EDGE_CURVE ( 'NONE', #4508, #19453, #243457, .T. ) ;
#244195=ORIENTED_EDGE ( 'NONE', *, *, #86783, .T. ) ;
#244280=CYLINDRICAL_SURFACE ( 'NONE', #170221, 0.1000000000000000472 ) ;
#244283=CARTESIAN_POINT ( 'NONE',  ( 23.24999999999999645, 0.000000000000000000, 0.000000000000000000 ) ) ;
#244352=CARTESIAN_POINT ( 'NONE',  ( -23.25000000000000000, 4.349999999999999645, -21.34999999999999787 ) ) ;
#244361=VECTOR ( 'NONE', #172761, 1000.000000000000000 ) ;
#244370=DIRECTION ( 'NONE',  ( 1.000000000000000000, 0.000000000000000000, 0.000000000000000000 ) ) ;
#244376=CIRCLE ( 'NONE', #131955, 0.09999999999999939493 ) ;
#244383=CARTESIAN_POINT ( 'NONE',  ( -23.15000000000000213, 4.349999999999999645, -21.14999999999999858 ) ) ;
#244398=AXIS2_PLACEMENT_3D ( 'NONE', #230519, #253908, #152282 ) ;
#244406=ORIENTED_EDGE ( 'NONE', *, *, #246762, .F. ) ;
#244416=B_SPLINE_CURVE_WITH_KNOTS ( 'NONE', 3,
 ( #218046, #155568, #39470, #96803, #197218, #177697, #115124, #257143, #35620, #215498 ),
 .UNSPECIFIED., .F., .F.,
 ( 4, 2, 2, 2, 4 ),
 ( 0.000000000000000000, 4.221631689686865393E-05, 8.443263379373730786E-05, 0.0001688652675874746157, 0.0003377305351749315589 ),
 .UNSPECIFIED. ) ;
#244433=AXIS2_PLACEMENT_3D ( 'NONE', #48639, #53784, #107333 ) ;
#244441=CIRCLE ( 'NONE', #56985, 0.1000000000000001721 ) ;
#244452=ORIENTED_EDGE ( 'NONE', *, *, #110945, .T. ) ;
#244460=CIRCLE ( 'NONE', #206875, 0.09999999999999997780 ) ;
#244468=VERTEX_POINT ( 'NONE', #59343 ) ;
#244476=DIRECTION ( 'NONE',  ( -2.812466655313719426E-14, 0.1350103645451904977, 0.9908441862701596881 ) ) ;
#244481=DIRECTION ( 'NONE',  ( 0.000000000000000000, -0.8777080977375132376, 0.4791956752371582251 ) ) ;
#244502=DIRECTION ( 'NONE',  ( -1.000000000000000000, 0.000000000000000000, 0.000000000000000000 ) ) ;
#244508=CIRCLE ( 'NONE', #219560, 3.999999999999999112 ) ;
#244526=VERTEX_POINT ( 'NONE', #163627 ) ;
#244561=DIRECTION ( 'NONE',  ( 1.000000000000000000, 0.000000000000000000, -0.000000000000000000 ) ) ;
#244570=ORIENTED_EDGE ( 'NONE', *, *, #125653, .T. ) ;
#244575=DIRECTION ( 'NONE',  ( 0.000000000000000000, 0.000000000000000000, -1.000000000000000000 ) ) ;
#244582=ORIENTED_EDGE ( 'NONE', *, *, #251257, .T. ) ;
#244603=EDGE_CURVE ( 'NONE', #12754, #14945, #145329, .T. ) ;
#244646=DIRECTION ( 'NONE',  ( 0.000000000000000000, -0.000000000000000000, -1.000000000000000000 ) ) ;
#244687=CARTESIAN_POINT ( 'NONE',  ( 21.14999999999999503, -11.74999999999999112, -2.900000000000003464 ) ) ;
#244713=FACE_OUTER_BOUND ( 'NONE', #30994, .T. ) ;
#244734=AXIS2_PLACEMENT_3D ( 'NONE', #245047, #108109, #65118 ) ;
#244742=VERTEX_POINT ( 'NONE', #246996 ) ;
#244746=AXIS2_PLACEMENT_3D ( 'NONE', #49883, #87711, #146393 ) ;
#244755=ORIENTED_EDGE ( 'NONE', *, *, #236469, .T. ) ;
#244756=DIRECTION ( 'NONE',  ( 1.000000000000000000, -0.000000000000000000, -0.000000000000000000 ) ) ;
#244786=CIRCLE ( 'NONE', #165134, 0.09999999999999939493 ) ;
#244818=VERTEX_POINT ( 'NONE', #155648 ) ;
#244834=ORIENTED_EDGE ( 'NONE', *, *, #195307, .T. ) ;
#244855=ADVANCED_FACE ( 'NONE', ( #59041 ), #243151, .T. ) ;
#244862=DIRECTION ( 'NONE',  ( 0.000000000000000000, -0.9908441862701596881, -0.1350103645451904977 ) ) ;
#244866=EDGE_LOOP ( 'NONE', ( #159000, #24753, #255065, #187079 ) ) ;
#244871=DIRECTION ( 'NONE',  ( 0.000000000000000000, 0.8700118002898321601, -0.4930308989875230030 ) ) ;
#244885=CARTESIAN_POINT ( 'NONE',  ( -18.59999999999999787, -1.835859311443637010, -45.00443916879852679 ) ) ;
#244920=ORIENTED_EDGE ( 'NONE', *, *, #101229, .F. ) ;
#244942=DIRECTION ( 'NONE',  ( 1.000000000000000000, -0.000000000000000000, -0.000000000000000000 ) ) ;
#244947=CARTESIAN_POINT ( 'NONE',  ( -18.59999999999999787, 1.835341550224411922, -11.55515129256298046 ) ) ;
#244978=EDGE_LOOP ( 'NONE', ( #200208, #118083, #137119, #226999 ) ) ;
#244988=CARTESIAN_POINT ( 'NONE',  ( -20.94999999999999929, -1.164121893241208960, -41.41484808557160591 ) ) ;
#245013=DIRECTION ( 'NONE',  ( 1.000000000000000000, 0.000000000000000000, 0.000000000000000000 ) ) ;
#245040=AXIS2_PLACEMENT_3D ( 'NONE', #152388, #170691, #74138 ) ;
#245047=CARTESIAN_POINT ( 'NONE',  ( -21.05000000000000071, 0.000000000000000000, 0.000000000000000000 ) ) ;
#245092=DIRECTION ( 'NONE',  ( 0.000000000000000000, 1.000000000000000000, 0.000000000000000000 ) ) ;
#245097=EDGE_CURVE ( 'NONE', #208385, #172995, #43612, .T. ) ;
#245136=VECTOR ( 'NONE', #105085, 1000.000000000000000 ) ;
#245165=EDGE_LOOP ( 'NONE', ( #228389, #249600, #249943, #219947 ) ) ;
#245166=CARTESIAN_POINT ( 'NONE',  ( -18.50000000000000000, 1.340746217933695750, 10.27286250542118040 ) ) ;
#245259=CARTESIAN_POINT ( 'NONE',  ( -21.05000000000000071, 6.257814610481521989, 0.09779029130922732571 ) ) ;
#245277=EDGE_CURVE ( 'NONE', #38380, #16525, #97744, .T. ) ;
#245285=CIRCLE ( 'NONE', #132868, 0.5000000000000022204 ) ;
#245306=VECTOR ( 'NONE', #70412, 1000.000000000000000 ) ;
#245328=DIRECTION ( 'NONE',  ( 1.000000000000000000, 0.000000000000000000, 0.000000000000000000 ) ) ;
#245358=VECTOR ( 'NONE', #225295, 1000.000000000000000 ) ;
#245373=CARTESIAN_POINT ( 'NONE',  ( -21.05000000000000071, 1.162701749938009677, -8.099999999999999645 ) ) ;
#245384=AXIS2_PLACEMENT_3D ( 'NONE', #143283, #41645, #42910 ) ;
#245390=CARTESIAN_POINT ( 'NONE',  ( 21.05000000000000071, -11.64999999999999147, -30.39999999999999503 ) ) ;
#245411=EDGE_CURVE ( 'NONE', #201638, #226285, #143577, .T. ) ;
#245419=LINE ( 'NONE', #87595, #132991 ) ;
#245427=VERTEX_POINT ( 'NONE', #34954 ) ;
#245429=CIRCLE ( 'NONE', #203727, 0.09999999999999939493 ) ;
#245463=DIRECTION ( 'NONE',  ( 0.000000000000000000, 0.000000000000000000, 1.000000000000000000 ) ) ;
#245471=CIRCLE ( 'NONE', #87217, 0.09999999999999939493 ) ;
#245472=CYLINDRICAL_SURFACE ( 'NONE', #57177, 0.09999999999999939493 ) ;
#245479=FACE_OUTER_BOUND ( 'NONE', #211692, .T. ) ;
#245501=EDGE_LOOP ( 'NONE', ( #321, #126060, #105600, #164573, #126398, #155953, #10889 ) ) ;
#245518=DIRECTION ( 'NONE',  ( -3.265361837132813093E-16, 1.000000000000000000, 0.000000000000000000 ) ) ;
#245531=ADVANCED_FACE ( 'NONE', ( #55039 ), #94176, .F. ) ;
#245540=ORIENTED_EDGE ( 'NONE', *, *, #185994, .F. ) ;
#245567=CARTESIAN_POINT ( 'NONE',  ( -18.51024323315077424, 10.31104185822947095, -39.02045169831058047 ) ) ;
#245574=EDGE_LOOP ( 'NONE', ( #246007, #217273, #153512, #131942 ) ) ;
#245581=EDGE_CURVE ( 'NONE', #127799, #214167, #139453, .T. ) ;
#245587=CARTESIAN_POINT ( 'NONE',  ( -20.54999999999999716, 1.925233644859816629, -12.73024353312613144 ) ) ;
#245588=CARTESIAN_POINT ( 'NONE',  ( 20.94999999999999574, 1.849084418627015891, -11.65601052144712391 ) ) ;
#245595=CARTESIAN_POINT ( 'NONE',  ( 21.04386569057580658, 11.74999999999974598, -26.64283735177988177 ) ) ;
#245600=CARTESIAN_POINT ( 'NONE',  ( 20.94999999999999929, -8.730841121495327428, -9.598074718984332065 ) ) ;
#245627=VERTEX_POINT ( 'NONE', #154215 ) ;
#245643=EDGE_CURVE ( 'NONE', #73708, #83068, #220562, .T. ) ;
#245648=DIRECTION ( 'NONE',  ( 1.000000000000000000, 2.952720810173289112E-16, -0.000000000000000000 ) ) ;
#245688=ORIENTED_EDGE ( 'NONE', *, *, #45890, .F. ) ;
#245705=ADVANCED_FACE ( 'NONE', ( #216 ), #238840, .F. ) ;
#245725=EDGE_CURVE ( 'NONE', #17057, #241011, #181451, .T. ) ;
#245750=ORIENTED_EDGE ( 'NONE', *, *, #151323, .F. ) ;
#245776=ORIENTED_EDGE ( 'NONE', *, *, #29714, .F. ) ;
#245783=EDGE_LOOP ( 'NONE', ( #225922, #198761 ) ) ;
#245826=ORIENTED_EDGE ( 'NONE', *, *, #169395, .T. ) ;
#245834=LINE ( 'NONE', #219841, #53319 ) ;
#245851=CYLINDRICAL_SURFACE ( 'NONE', #74955, 0.09999999999999939493 ) ;
#245857=ADVANCED_FACE ( 'NONE', ( #168338 ), #10512, .F. ) ;
#245895=CYLINDRICAL_SURFACE ( 'NONE', #209163, 12.87499999999999822 ) ;
#245925=ORIENTED_EDGE ( 'NONE', *, *, #177693, .T. ) ;
#245939=ORIENTED_EDGE ( 'NONE', *, *, #182763, .F. ) ;
#245961=CIRCLE ( 'NONE', #4323, 6.329289321881357289 ) ;
#245976=EDGE_CURVE ( 'NONE', #194720, #47350, #187036, .T. ) ;
#245980=DIRECTION ( 'NONE',  ( -0.000000000000000000, 0.000000000000000000, 1.000000000000000000 ) ) ;
#245989=CARTESIAN_POINT ( 'NONE',  ( 18.39999999999999858, -9.499999999999998224, -40.10018939122204529 ) ) ;
#246007=ORIENTED_EDGE ( 'NONE', *, *, #210130, .T. ) ;
#246012=VECTOR ( 'NONE', #240501, 1000.000000000000114 ) ;
#246027=VERTEX_POINT ( 'NONE', #152611 ) ;
#246037=EDGE_CURVE ( 'NONE', #192810, #27728, #158018, .T. ) ;
#246044=ADVANCED_FACE ( 'NONE', ( #241123 ), #149610, .T. ) ;
#246057=ADVANCED_FACE ( 'NONE', ( #196829 ), #139408, .T. ) ;
#246061=CIRCLE ( 'NONE', #250339, 12.77499999999999503 ) ;
#246062=CARTESIAN_POINT ( 'NONE',  ( -20.94999999999999929, 11.74999999999999645, -7.014805770654001016 ) ) ;
#246065=EDGE_CURVE ( 'NONE', #125216, #253366, #159028, .T. ) ;
#246075=FACE_OUTER_BOUND ( 'NONE', #215234, .T. ) ;
#246105=ORIENTED_EDGE ( 'NONE', *, *, #213973, .T. ) ;
#246106=TOROIDAL_SURFACE ( 'NONE', #71333, 7.791421356237316687, 0.1000000000000000056 ) ;
#246119=DIRECTION ( 'NONE',  ( -7.304098846218134667E-16, -1.000000000000000000, 0.000000000000000000 ) ) ;
#246201=CARTESIAN_POINT ( 'NONE',  ( -18.50000000000000000, 9.250000000000001776, -21.15000000000000213 ) ) ;
#246220=AXIS2_PLACEMENT_3D ( 'NONE', #58094, #196342, #38563 ) ;
#246260=AXIS2_PLACEMENT_3D ( 'NONE', #64430, #184357, #124407 ) ;
#246319=DIRECTION ( 'NONE',  ( 1.000000000000000000, 0.000000000000000000, 0.000000000000000000 ) ) ;
#246330=CIRCLE ( 'NONE', #42321, 0.09999999999999939493 ) ;
#246332=FACE_OUTER_BOUND ( 'NONE', #24242, .T. ) ;
#246344=ADVANCED_FACE ( 'NONE', ( #152294 ), #173166, .T. ) ;
#246358=ORIENTED_EDGE ( 'NONE', *, *, #201903, .T. ) ;
#246393=DIRECTION ( 'NONE',  ( 1.000000000000000000, 0.000000000000000000, 0.000000000000000000 ) ) ;
#246418=DIRECTION ( 'NONE',  ( 1.000000000000000000, -0.000000000000000000, -0.000000000000000000 ) ) ;
#246436=DIRECTION ( 'NONE',  ( -1.000000000000000000, -1.836970198721029934E-16, -3.186635328391151676E-31 ) ) ;
#246451=CARTESIAN_POINT ( 'NONE',  ( 20.94999999999999574, -1.162701749938009677, -8.099999999999999645 ) ) ;
#246475=DIRECTION ( 'NONE',  ( -4.239556034732056743E-17, 0.1298341882520022694, 0.9915357197604853789 ) ) ;
#246497=CIRCLE ( 'NONE', #154386, 0.09999999999999939493 ) ;
#246509=EDGE_CURVE ( 'NONE', #109031, #204739, #49813, .T. ) ;
#246513=ORIENTED_EDGE ( 'NONE', *, *, #216786, .T. ) ;
#246525=CARTESIAN_POINT ( 'NONE',  ( -20.64999999999999858, 7.150000000000000355, -12.34999999999999964 ) ) ;
#246603=DIRECTION ( 'NONE',  ( 0.000000000000000000, 0.000000000000000000, -1.000000000000000000 ) ) ;
#246674=CARTESIAN_POINT ( 'NONE',  ( -21.05000000000000071, 1.851028230140860487, -11.65391326942249606 ) ) ;
#246754=ORIENTED_EDGE ( 'NONE', *, *, #130993, .F. ) ;
#246761=ORIENTED_EDGE ( 'NONE', *, *, #20511, .F. ) ;
#246762=EDGE_CURVE ( 'NONE', #47980, #27728, #153276, .T. ) ;
#246763=ORIENTED_EDGE ( 'NONE', *, *, #160963, .T. ) ;
#246772=DIRECTION ( 'NONE',  ( 0.000000000000000000, 0.4999999999999956701, -0.8660254037844411501 ) ) ;
#246775=ORIENTED_EDGE ( 'NONE', *, *, #128981, .T. ) ;
#246776=CARTESIAN_POINT ( 'NONE',  ( -20.64999999999999858, -8.730841121495327428, -9.598074718984330289 ) ) ;
#246802=ORIENTED_EDGE ( 'NONE', *, *, #256521, .T. ) ;
#246815=DIRECTION ( 'NONE',  ( -1.000000000000000000, 0.000000000000000000, 0.000000000000000000 ) ) ;
#246817=ADVANCED_FACE ( 'NONE', ( #168993 ), #199869, .F. ) ;
#246819=FACE_OUTER_BOUND ( 'NONE', #35473, .T. ) ;
#246829=DIRECTION ( 'NONE',  ( -2.978066053179067751E-16, 1.000000000000000000, 0.000000000000000000 ) ) ;
#246838=ADVANCED_FACE ( 'NONE', ( #201032 ), #79771, .T. ) ;
#246841=EDGE_LOOP ( 'NONE', ( #167199, #144013, #36744, #200521 ) ) ;
#246849=CYLINDRICAL_SURFACE ( 'NONE', #42458, 0.09999999999999939493 ) ;
#246851=CYLINDRICAL_SURFACE ( 'NONE', #170064, 12.87499999999999822 ) ;
#246858=CARTESIAN_POINT ( 'NONE',  ( 20.99780126800938262, 11.60538868787666011, -26.58735257170533473 ) ) ;
#246865=CARTESIAN_POINT ( 'NONE',  ( -20.85000000000000142, 11.74999999999999645, -26.65839931010294350 ) ) ;
#246879=AXIS2_PLACEMENT_3D ( 'NONE', #244885, #227897, #109220 ) ;
#246898=CARTESIAN_POINT ( 'NONE',  ( -20.85000000000000142, 11.64999999999999680, -33.50000000000000000 ) ) ;
#246971=VECTOR ( 'NONE', #161361, 1000.000000000000000 ) ;
#246984=DIRECTION ( 'NONE',  ( 1.000000000000000000, -0.000000000000000000, -0.000000000000000000 ) ) ;
#246988=DIRECTION ( 'NONE',  ( 0.000000000000000000, 0.000000000000000000, 1.000000000000000000 ) ) ;
#246996=CARTESIAN_POINT ( 'NONE',  ( 23.14999999999999858, -2.000000000000002665, -33.50000000000000000 ) ) ;
#247016=ORIENTED_EDGE ( 'NONE', *, *, #146797, .F. ) ;
#247031=PLANE ( 'NONE',  #61874 ) ;
#247033=CARTESIAN_POINT ( 'NONE',  ( 20.95512820512820440, 10.62384868371188062, -7.664913569087605794 ) ) ;
#247054=DIRECTION ( 'NONE',  ( 1.000000000000000000, -0.000000000000000000, -0.000000000000000000 ) ) ;
#247089=EDGE_CURVE ( 'NONE', #105911, #230477, #41836, .T. ) ;
#247114=DIRECTION ( 'NONE',  ( 0.7070776581709139474, -0.7071359030027652981, -2.453168425935592377E-14 ) ) ;
#247147=ORIENTED_EDGE ( 'NONE', *, *, #107678, .F. ) ;
#247150=VERTEX_POINT ( 'NONE', #187903 ) ;
#247153=CARTESIAN_POINT ( 'NONE',  ( 21.05000000000000071, 6.649999999999999467, -12.15000000000000036 ) ) ;
#247162=ORIENTED_EDGE ( 'NONE', *, *, #101044, .F. ) ;
#247171=CARTESIAN_POINT ( 'NONE',  ( 20.94999999999999929, 5.021051876504146399E-16, -29.40000000000000213 ) ) ;
#247179=EDGE_CURVE ( 'NONE', #99784, #8515, #21351, .T. ) ;
#247194=ADVANCED_FACE ( 'NONE', ( #33996 ), #83650, .T. ) ;
#247215=DIRECTION ( 'NONE',  ( 1.000000000000000000, 0.000000000000000000, -0.000000000000000000 ) ) ;
#247222=ORIENTED_EDGE ( 'NONE', *, *, #119733, .F. ) ;
#247228=AXIS2_PLACEMENT_3D ( 'NONE', #234298, #214739, #136466 ) ;
#247239=CARTESIAN_POINT ( 'NONE',  ( -22.49436431346200038, 11.64995094765345840, 0.06690352972225574457 ) ) ;
#247244=CARTESIAN_POINT ( 'NONE',  ( -20.94999999999999929, -1.249999999999999334, -8.000000000000000000 ) ) ;
#247290=ORIENTED_EDGE ( 'NONE', *, *, #86783, .F. ) ;
#247295=DIRECTION ( 'NONE',  ( 1.000000000000000000, 0.000000000000000000, 0.000000000000000000 ) ) ;
#247341=VECTOR ( 'NONE', #154657, 1000.000000000000000 ) ;
#247358=CARTESIAN_POINT ( 'NONE',  ( 18.59999999999999076, 10.20857864376269575, -21.35000000000000142 ) ) ;
#247366=EDGE_LOOP ( 'NONE', ( #95279, #82874, #39838, #34910 ) ) ;
#247371=FACE_OUTER_BOUND ( 'NONE', #72868, .T. ) ;
#247414=DIRECTION ( 'NONE',  ( 0.000000000000000000, 1.000000000000000000, 0.000000000000000000 ) ) ;
#247429=EDGE_CURVE ( 'NONE', #209763, #217421, #254351, .T. ) ;
#247445=ADVANCED_FACE ( 'NONE', ( #83311 ), #78199, .F. ) ;
#247474=EDGE_CURVE ( 'NONE', #240042, #216736, #175296, .T. ) ;
#247490=ADVANCED_FACE ( 'NONE', ( #128901 ), #187603, .T. ) ;
#247492=ORIENTED_EDGE ( 'NONE', *, *, #146696, .T. ) ;
#247512=ADVANCED_FACE ( 'NONE', ( #148467 ), #104506, .T. ) ;
#247520=EDGE_CURVE ( 'NONE', #201638, #89621, #46251, .T. ) ;
#247524=VECTOR ( 'NONE', #125238, 1000.000000000000000 ) ;
#247538=CARTESIAN_POINT ( 'NONE',  ( -23.25000000000000000, -11.75000000000000000, 3.469446951953614189E-15 ) ) ;
#247543=CARTESIAN_POINT ( 'NONE',  ( -18.59999999999999787, 11.64999999999999680, -7.014805770654001016 ) ) ;
#247581=CARTESIAN_POINT ( 'NONE',  ( -18.50000000000000000, -9.400000000000005684, -40.38204184817266906 ) ) ;
#247602=ORIENTED_EDGE ( 'NONE', *, *, #203286, .T. ) ;
#247644=FACE_OUTER_BOUND ( 'NONE', #64063, .T. ) ;
#247674=FACE_OUTER_BOUND ( 'NONE', #209752, .T. ) ;
#247677=ORIENTED_EDGE ( 'NONE', *, *, #130343, .T. ) ;
#247696=TOROIDAL_SURFACE ( 'NONE', #55955, 2.100000000000002309, 0.1000000000000000056 ) ;
#247734=VECTOR ( 'NONE', #55560, 1000.000000000000000 ) ;
#247743=DIRECTION ( 'NONE',  ( 0.000000000000000000, 0.000000000000000000, -1.000000000000000000 ) ) ;
#247747=FACE_OUTER_BOUND ( 'NONE', #220544, .T. ) ;
#247786=AXIS2_PLACEMENT_3D ( 'NONE', #6079, #243416, #64776 ) ;
#247796=CIRCLE ( 'NONE', #6365, 0.09999999999999939493 ) ;
#247818=TOROIDAL_SURFACE ( 'NONE', #56255, 0.2000000000000000111, 0.1000000000000000056 ) ;
#247821=DIRECTION ( 'NONE',  ( -0.000000000000000000, -0.8660254037844411501, -0.4999999999999956701 ) ) ;
#247873=CARTESIAN_POINT ( 'NONE',  ( 21.05000000000000071, -12.41227409414968541, -30.50000000000000000 ) ) ;
#247892=FACE_OUTER_BOUND ( 'NONE', #256740, .T. ) ;
#247932=DIRECTION ( 'NONE',  ( -2.952720810173289112E-16, 1.000000000000000000, 0.000000000000000000 ) ) ;
#247961=FACE_OUTER_BOUND ( 'NONE', #31380, .T. ) ;
#247976=ORIENTED_EDGE ( 'NONE', *, *, #64538, .F. ) ;
#247985=CYLINDRICAL_SURFACE ( 'NONE', #255716, 0.09999999999999939493 ) ;
#248005=ORIENTED_EDGE ( 'NONE', *, *, #182302, .F. ) ;
#248073=FACE_OUTER_BOUND ( 'NONE', #174589, .T. ) ;
#248074=DIRECTION ( 'NONE',  ( 1.000000000000000000, 0.000000000000000000, 0.000000000000000000 ) ) ;
#248081=EDGE_LOOP ( 'NONE', ( #76211, #129125, #89926, #20344 ) ) ;
#248100=CARTESIAN_POINT ( 'NONE',  ( 20.85000000000000142, -1.835859311443637010, -45.00443916879852679 ) ) ;
#248114=CYLINDRICAL_SURFACE ( 'NONE', #140903, 0.09999999999999939493 ) ;
#248123=AXIS2_PLACEMENT_3D ( 'NONE', #98469, #179361, #3249 ) ;
#248130=EDGE_CURVE ( 'NONE', #8661, #246027, #30790, .T. ) ;
#248147=VECTOR ( 'NONE', #208224, 1000.000000000000000 ) ;
#248163=AXIS2_PLACEMENT_3D ( 'NONE', #74476, #194410, #154027 ) ;
#248177=DIRECTION ( 'NONE',  ( 0.000000000000000000, -1.776356839400250465E-15, 1.000000000000000000 ) ) ;
#248186=CARTESIAN_POINT ( 'NONE',  ( 21.05000000000000071, 10.72371710470752149, -7.664913569087605794 ) ) ;
#248199=CYLINDRICAL_SURFACE ( 'NONE', #199036, 0.09999999999999939493 ) ;
#248216=TOROIDAL_SURFACE ( 'NONE', #98313, 11.65000000000000036, 0.1000000000000000056 ) ;
#248243=AXIS2_PLACEMENT_3D ( 'NONE', #107887, #49198, #27105 ) ;
#248248=VERTEX_POINT ( 'NONE', #119295 ) ;
#248264=ADVANCED_FACE ( 'NONE', ( #29222 ), #226056, .F. ) ;
#248267=ORIENTED_EDGE ( 'NONE', *, *, #41955, .T. ) ;
#248338=CARTESIAN_POINT ( 'NONE',  ( -21.44999999999999929, 7.349999999999998757, -21.25000000000000000 ) ) ;
#248355=DIRECTION ( 'NONE',  ( -1.000000000000000000, 0.000000000000000000, -0.000000000000000000 ) ) ;
#248359=DIRECTION ( 'NONE',  ( -0.000000000000000000, 1.000000000000000000, -0.000000000000000000 ) ) ;
#248365=SURFACE_STYLE_FILL_AREA ( #9745 ) ;
#248376=CARTESIAN_POINT ( 'NONE',  ( -20.00857864376270001, 9.150000000000002132, -21.15000000000000213 ) ) ;
#248377=PLANE ( 'NONE',  #14148 ) ;
#248401=AXIS2_PLACEMENT_3D ( 'NONE', #146194, #242725, #184043 ) ;
#248418=DIRECTION ( 'NONE',  ( 0.000000000000000000, 1.224646799147316229E-16, 1.000000000000000000 ) ) ;
#248496=CARTESIAN_POINT ( 'NONE',  ( 20.94403535211772294, 10.30632246270531738, -39.00418367788957852 ) ) ;
#248503=CARTESIAN_POINT ( 'NONE',  ( 21.05000000000000071, 2.326828918379974323E-16, -31.59999999999999787 ) ) ;
#248513=ORIENTED_EDGE ( 'NONE', *, *, #150686, .T. ) ;
#248517=CARTESIAN_POINT ( 'NONE',  ( 23.15000000000000213, -11.48912529307605546, -30.50000000000000000 ) ) ;
#248519=AXIS2_PLACEMENT_3D ( 'NONE', #177094, #217453, #216177 ) ;
#248548=VERTEX_POINT ( 'NONE', #141127 ) ;
#248610=CIRCLE ( 'NONE', #2900, 4.099999999999999645 ) ;
#248617=ORIENTED_EDGE ( 'NONE', *, *, #15609, .F. ) ;
#248651=CARTESIAN_POINT ( 'NONE',  ( -22.47071067811865319, 0.09909245470260570621, 7.720074744498060859 ) ) ;
#248669=LINE ( 'NONE', #129985, #231471 ) ;
#248680=AXIS2_PLACEMENT_3D ( 'NONE', #200605, #138044, #100187 ) ;
#248688=FACE_OUTER_BOUND ( 'NONE', #246841, .T. ) ;
#248727=ORIENTED_EDGE ( 'NONE', *, *, #184534, .F. ) ;
#248752=FACE_OUTER_BOUND ( 'NONE', #231731, .T. ) ;
#248757=EDGE_LOOP ( 'NONE', ( #67700, #169013, #28724, #238919 ) ) ;
#248759=DIRECTION ( 'NONE',  ( -1.000000000000000000, 0.000000000000000000, 0.000000000000000000 ) ) ;
#248780=CARTESIAN_POINT ( 'NONE',  ( 21.13920837816993270, 8.783247050119912913, -12.25000000000000000 ) ) ;
#248788=DIRECTION ( 'NONE',  ( 1.000000000000000000, -0.000000000000000000, -0.000000000000000000 ) ) ;
#248803=EDGE_LOOP ( 'NONE', ( #1410, #109027, #185459, #208617 ) ) ;
#248816=AXIS2_PLACEMENT_3D ( 'NONE', #247543, #225388, #46757 ) ;
#248846=DIRECTION ( 'NONE',  ( 0.000000000000000000, 0.000000000000000000, -1.000000000000000000 ) ) ;
#248853=DIRECTION ( 'NONE',  ( 0.000000000000000000, 0.000000000000000000, 1.000000000000000000 ) ) ;
#248897=CARTESIAN_POINT ( 'NONE',  ( -21.05000000000000071, 0.000000000000000000, -4.299999999999956302 ) ) ;
#248906=CYLINDRICAL_SURFACE ( 'NONE', #143224, 0.8750000000000007772 ) ;
#248909=DIRECTION ( 'NONE',  ( 0.000000000000000000, 0.000000000000000000, -1.000000000000000000 ) ) ;
#248978=ORIENTED_EDGE ( 'NONE', *, *, #85466, .T. ) ;
#249018=AXIS2_PLACEMENT_3D ( 'NONE', #143681, #161995, #100675 ) ;
#249020=CARTESIAN_POINT ( 'NONE',  ( 21.14999999999999858, 0.000000000000000000, 0.000000000000000000 ) ) ;
#249051=ORIENTED_EDGE ( 'NONE', *, *, #105872, .T. ) ;
#249057=DIRECTION ( 'NONE',  ( -0.000000000000000000, -0.000000000000000000, 1.000000000000000000 ) ) ;
#249069=ORIENTED_EDGE ( 'NONE', *, *, #44445, .T. ) ;
#249082=LINE ( 'NONE', #11761, #223084 ) ;
#249102=CYLINDRICAL_SURFACE ( 'NONE', #134194, 0.09999999999999939493 ) ;
#249104=CARTESIAN_POINT ( 'NONE',  ( -21.07954763557447109, 0.06587591861840921825, 6.329290990037786280 ) ) ;
#249109=VECTOR ( 'NONE', #209595, 1000.000000000000000 ) ;
#249130=CARTESIAN_POINT ( 'NONE',  ( -18.50000000000000711, -9.419203418026649288, -7.247785810428664099 ) ) ;
#249131=CARTESIAN_POINT ( 'NONE',  ( 21.05000000000000071, 5.399999999999998579, -23.60603087734755690 ) ) ;
#249139=ADVANCED_FACE ( 'NONE', ( #128186 ), #25769, .F. ) ;
#249151=ORIENTED_EDGE ( 'NONE', *, *, #123370, .T. ) ;
#249175=AXIS2_PLACEMENT_3D ( 'NONE', #257, #152965, #55077 ) ;
#249201=ORIENTED_EDGE ( 'NONE', *, *, #81221, .T. ) ;
#249204=CARTESIAN_POINT ( 'NONE',  ( -21.44999999999999929, 7.349999999999998757, -21.15000000000000213 ) ) ;
#249210=CARTESIAN_POINT ( 'NONE',  ( -20.85000000000000142, -11.75000000000000000, -33.50000000000000000 ) ) ;
#249222=ORIENTED_EDGE ( 'NONE', *, *, #86973, .F. ) ;
#249231=ADVANCED_FACE ( 'NONE', ( #70805 ), #210299, .F. ) ;
#249241=ORIENTED_EDGE ( 'NONE', *, *, #142886, .F. ) ;
#249248=DIRECTION ( 'NONE',  ( -1.000000000000000000, 0.000000000000000000, 0.000000000000000000 ) ) ;
#249260=LINE ( 'NONE', #11948, #62904 ) ;
#249270=CYLINDRICAL_SURFACE ( 'NONE', #150128, 0.09999999999999939493 ) ;
#249326=CARTESIAN_POINT ( 'NONE',  ( 18.60000000000000497, 0.000000000000000000, 0.000000000000000000 ) ) ;
#249368=VERTEX_POINT ( 'NONE', #45173 ) ;
#249385=ORIENTED_EDGE ( 'NONE', *, *, #159943, .F. ) ;
#249394=CARTESIAN_POINT ( 'NONE',  ( -18.59999999999999787, -1.263275465217258198, -41.40186466674640542 ) ) ;
#249449=CARTESIAN_POINT ( 'NONE',  ( -20.54999999999999716, 0.000000000000000000, -33.50000000000000000 ) ) ;
#249454=CARTESIAN_POINT ( 'NONE',  ( 21.05000000000000071, 10.72371710470752149, 0.000000000000000000 ) ) ;
#249468=EDGE_LOOP ( 'NONE', ( #165456, #162067, #153576, #165766 ) ) ;
#249469=DIRECTION ( 'NONE',  ( -0.000000000000000000, 0.000000000000000000, -1.000000000000000000 ) ) ;
#249471=CARTESIAN_POINT ( 'NONE',  ( 21.07928932188134397, 0.000000000000000000, 0.000000000000000000 ) ) ;
#249474=ORIENTED_EDGE ( 'NONE', *, *, #134759, .F. ) ;
#249488=AXIS2_PLACEMENT_3D ( 'NONE', #157044, #116618, #256064 ) ;
#249518=DIRECTION ( 'NONE',  ( -0.000000000000000000, -0.000000000000000000, 1.000000000000000000 ) ) ;
#249534=CARTESIAN_POINT ( 'NONE',  ( -23.15000000000000213, 1.925233644859816629, -12.73024353312613144 ) ) ;
#249554=ORIENTED_EDGE ( 'NONE', *, *, #86375, .T. ) ;
#249564=DIRECTION ( 'NONE',  ( -1.000000000000000000, 0.000000000000000000, 0.000000000000000000 ) ) ;
#249566=AXIS2_PLACEMENT_3D ( 'NONE', #249131, #70511, #229559 ) ;
#249573=CARTESIAN_POINT ( 'NONE',  ( -23.25000000000000000, 7.021664781900089913, -37.33356540189728889 ) ) ;
#249574=CARTESIAN_POINT ( 'NONE',  ( 18.59999999999999787, -1.835341550224411922, -11.55515129256297868 ) ) ;
#249598=DIRECTION ( 'NONE',  ( 0.000000000000000000, 0.000000000000000000, -1.000000000000000000 ) ) ;
#249600=ORIENTED_EDGE ( 'NONE', *, *, #222853, .F. ) ;
#249613=AXIS2_PLACEMENT_3D ( 'NONE', #172189, #251670, #242369 ) ;
#249634=VERTEX_POINT ( 'NONE', #224776 ) ;
#249706=CARTESIAN_POINT ( 'NONE',  ( -21.44999999999999929, 7.349999999999998757, -12.25000000000000000 ) ) ;
#249708=DIRECTION ( 'NONE',  ( 0.000000000000000000, 0.000000000000000000, -1.000000000000000000 ) ) ;
#249726=ADVANCED_FACE ( 'NONE', ( #44876 ), #61875, .T. ) ;
#249744=DIRECTION ( 'NONE',  ( 1.000000000000000000, 3.265361837132813093E-16, -0.000000000000000000 ) ) ;
#249747=EDGE_LOOP ( 'NONE', ( #156152, #41540, #100133, #215773 ) ) ;
#249771=DIRECTION ( 'NONE',  ( 1.000000000000000000, -0.000000000000000000, -0.000000000000000000 ) ) ;
#249778=CARTESIAN_POINT ( 'NONE',  ( 20.88420186297724257, 10.33025634371521662, -39.08709292826387838 ) ) ;
#249788=CARTESIAN_POINT ( 'NONE',  ( 21.11345278033283179, 8.882122073370972259, -12.24602217075528010 ) ) ;
#249815=CARTESIAN_POINT ( 'NONE',  ( 21.76363531954645936, 7.012936547871724713, 0.09900187429945014883 ) ) ;
#249838=CARTESIAN_POINT ( 'NONE',  ( -21.64999999999999858, 7.249999999999992895, -12.25000000000000000 ) ) ;
#249863=DIRECTION ( 'NONE',  ( 0.000000000000000000, 0.000000000000000000, -1.000000000000000000 ) ) ;
#249865=CYLINDRICAL_SURFACE ( 'NONE', #255800, 0.09999999999999939493 ) ;
#249876=DIRECTION ( 'NONE',  ( 0.000000000000000000, 1.776356839400250070E-15, 1.000000000000000000 ) ) ;
#249885=CARTESIAN_POINT ( 'NONE',  ( 20.94999999999999574, -11.64999999999999147, -2.900000000000003464 ) ) ;
#249888=AXIS2_PLACEMENT_3D ( 'NONE', #111305, #68326, #227385 ) ;
#249892=EDGE_CURVE ( 'NONE', #72309, #94186, #244416, .T. ) ;
#249915=DIRECTION ( 'NONE',  ( 0.000000000000000000, 1.000000000000000000, 0.000000000000000000 ) ) ;
#249936=EDGE_CURVE ( 'NONE', #17057, #133463, #151047, .T. ) ;
#249940=CARTESIAN_POINT ( 'NONE',  ( -22.14074124539699895, 0.09905289584407227232, 7.390077851043765911 ) ) ;
#249943=ORIENTED_EDGE ( 'NONE', *, *, #35266, .F. ) ;
#249955=ADVANCED_FACE ( 'NONE', ( #44577 ), #83652, .T. ) ;
#249971=FACE_OUTER_BOUND ( 'NONE', #130377, .T. ) ;
#249999=ORIENTED_EDGE ( 'NONE', *, *, #25189, .T. ) ;
#250026=ORIENTED_EDGE ( 'NONE', *, *, #199764, .F. ) ;
#250027=CARTESIAN_POINT ( 'NONE',  ( 21.04999999999999716, 8.872080675377937098, -8.521047418830562492 ) ) ;
#250029=ORIENTED_EDGE ( 'NONE', *, *, #179744, .T. ) ;
#250033=CARTESIAN_POINT ( 'NONE',  ( -18.50000000000000000, 9.350000000000001421, -12.14999999999999858 ) ) ;
#250037=AXIS2_PLACEMENT_3D ( 'NONE', #90902, #50467, #130010 ) ;
#250059=EDGE_CURVE ( 'NONE', #77408, #106998, #42021, .T. ) ;
#250063=DIRECTION ( 'NONE',  ( 1.000000000000000000, 0.000000000000000000, 0.000000000000000000 ) ) ;
#250086=DIRECTION ( 'NONE',  ( 0.000000000000000000, 1.224646799147363807E-16, 1.000000000000000000 ) ) ;
#250093=CARTESIAN_POINT ( 'NONE',  ( -23.15000000000000213, -9.500000000000003553, -9.893969122652446657 ) ) ;
#250128=EDGE_CURVE ( 'NONE', #204776, #119315, #205181, .T. ) ;
#250136=SPHERICAL_SURFACE ( 'NONE', #213953, 0.1000000000000000056 ) ;
#250147=CARTESIAN_POINT ( 'NONE',  ( 18.49999999999999645, 0.000000000000000000, -33.50000000000000000 ) ) ;
#250157=AXIS2_PLACEMENT_3D ( 'NONE', #43239, #164475, #24981 ) ;
#250182=CARTESIAN_POINT ( 'NONE',  ( 22.39999999999999503, 0.000000000000000000, 7.790779598373379855 ) ) ;
#250189=CARTESIAN_POINT ( 'NONE',  ( -21.05000000000000071, 6.258316057332023341, 0.06570161032208736429 ) ) ;
#250234=EDGE_CURVE ( 'NONE', #197777, #233325, #180274, .T. ) ;
#250241=FACE_OUTER_BOUND ( 'NONE', #83993, .T. ) ;
#250243=VERTEX_POINT ( 'NONE', #157834 ) ;
#250275=VERTEX_POINT ( 'NONE', #133096 ) ;
#250276=AXIS2_PLACEMENT_3D ( 'NONE', #204571, #226696, #248846 ) ;
#250296=CIRCLE ( 'NONE', #150354, 3.999999999999999112 ) ;
#250297=ORIENTED_EDGE ( 'NONE', *, *, #38135, .F. ) ;
#250311=DIRECTION ( 'NONE',  ( 1.000000000000000000, 0.000000000000000000, -0.000000000000000000 ) ) ;
#250319=LINE ( 'NONE', #129095, #206888 ) ;
#250339=AXIS2_PLACEMENT_3D ( 'NONE', #132602, #114309, #36073 ) ;
#250340=CARTESIAN_POINT ( 'NONE',  ( -20.85000000000000142, -1.164121893241208960, -41.41484808557160591 ) ) ;
#250343=DIRECTION ( 'NONE',  ( 0.000000000000000000, 0.000000000000000000, 1.000000000000000000 ) ) ;
#250347=DIRECTION ( 'NONE',  ( 1.000000000000000000, -0.000000000000000000, -0.000000000000000000 ) ) ;
#250352=VERTEX_POINT ( 'NONE', #56092 ) ;
#250358=ORIENTED_EDGE ( 'NONE', *, *, #45262, .F. ) ;
#250364=CARTESIAN_POINT ( 'NONE',  ( 22.16821283564876666, 7.558973340780761774, 1.462253661542695674E-16 ) ) ;
#250394=EDGE_LOOP ( 'NONE', ( #226493, #252565, #27178 ) ) ;
#250395=CIRCLE ( 'NONE', #171343, 3.999999999999996447 ) ;
#250437=AXIS2_PLACEMENT_3D ( 'NONE', #89702, #226648, #8902 ) ;
#250476=DIRECTION ( 'NONE',  ( -1.000000000000000000, 0.000000000000000000, 0.000000000000000000 ) ) ;
#250497=CIRCLE ( 'NONE', #204697, 0.1000000000000000472 ) ;
#250501=CIRCLE ( 'NONE', #669, 0.09999999999999996392 ) ;
#250511=EDGE_CURVE ( 'NONE', #47980, #62691, #217836, .T. ) ;
#250517=DIRECTION ( 'NONE',  ( -0.000000000000000000, -0.1350103645451876666, 0.9908441862701600211 ) ) ;
#250545=EDGE_CURVE ( 'NONE', #196401, #17135, #130195, .T. ) ;
#250551=ORIENTED_EDGE ( 'NONE', *, *, #193771, .T. ) ;
#250557=AXIS2_PLACEMENT_3D ( 'NONE', #185812, #42446, #226186 ) ;
#250598=CIRCLE ( 'NONE', #38241, 0.09999999999999939493 ) ;
#250609=CARTESIAN_POINT ( 'NONE',  ( 20.94999999999999929, -9.000000000000000000, -24.00603087734755547 ) ) ;
#250610=ORIENTED_EDGE ( 'NONE', *, *, #252388, .T. ) ;
#250678=CARTESIAN_POINT ( 'NONE',  ( 21.05000000000000071, 4.999999999999997335, -21.49473398108690603 ) ) ;
#250695=ORIENTED_EDGE ( 'NONE', *, *, #166871, .T. ) ;
#250738=CARTESIAN_POINT ( 'NONE',  ( 20.94999999999999929, 10.72371710470752149, -21.25000000000000000 ) ) ;
#250744=CARTESIAN_POINT ( 'NONE',  ( -18.50000000000000711, 11.74999999999999645, -7.014805770653998351 ) ) ;
#250748=ADVANCED_FACE ( 'NONE', ( #203009 ), #38995, .F. ) ;
#250767=VERTEX_POINT ( 'NONE', #179623 ) ;
#250774=ORIENTED_EDGE ( 'NONE', *, *, #143162, .F. ) ;
#250777=CIRCLE ( 'NONE', #204789, 0.5000000000000004441 ) ;
#250803=CARTESIAN_POINT ( 'NONE',  ( -20.94999999999999929, 11.75000000000000000, -7.014805770654001016 ) ) ;
#250822=VECTOR ( 'NONE', #155121, 1000.000000000000000 ) ;
#250854=VECTOR ( 'NONE', #120667, 1000.000000000000000 ) ;
#250917=EDGE_CURVE ( 'NONE', #117101, #158841, #234607, .T. ) ;
#250937=TOROIDAL_SURFACE ( 'NONE', #130148, 12.97499999999999787, 0.1000000000000000056 ) ;
#250946=FILL_AREA_STYLE ('',( #91886 ) ) ;
#250947=VECTOR ( 'NONE', #239676, 1000.000000000000000 ) ;
#250948=DIRECTION ( 'NONE',  ( -0.000000000000000000, 0.000000000000000000, 1.000000000000000000 ) ) ;
#250999=CARTESIAN_POINT ( 'NONE',  ( -20.64999999999999858, 7.150000000000000355, -21.15000000000000213 ) ) ;
#251010=CARTESIAN_POINT ( 'NONE',  ( -20.64999999999999858, -9.000000000000001776, -24.00603087734755903 ) ) ;
#251055=CARTESIAN_POINT ( 'NONE',  ( 20.97462148592286013, 8.874737576450577592, -12.25464433173102563 ) ) ;
#251071=EDGE_CURVE ( 'NONE', #24291, #90989, #147490, .T. ) ;
#251073=DIRECTION ( 'NONE',  ( -0.000000000000000000, -1.000000000000000000, 6.308085367188393199E-16 ) ) ;
#251086=CARTESIAN_POINT ( 'NONE',  ( 20.95595012432476167, 10.60417921307614542, -7.595769330218145932 ) ) ;
#251096=CARTESIAN_POINT ( 'NONE',  ( 20.94999999999999929, 0.000000000000000000, -30.59999999999999432 ) ) ;
#251098=VECTOR ( 'NONE', #84940, 1000.000000000000000 ) ;
#251111=EDGE_CURVE ( 'NONE', #13199, #224018, #184902, .T. ) ;
#251157=LINE ( 'NONE', #89522, #221742 ) ;
#251176=DIRECTION ( 'NONE',  ( 0.000000000000000000, -0.8660254037844411501, -0.4999999999999956146 ) ) ;
#251180=VERTEX_POINT ( 'NONE', #84984 ) ;
#251201=DIRECTION ( 'NONE',  ( -0.7071067811865475727, -0.7071067811865475727, 0.000000000000000000 ) ) ;
#251239=ADVANCED_FACE ( 'NONE', ( #204946 ), #144973, .T. ) ;
#251243=AXIS2_PLACEMENT_3D ( 'NONE', #63204, #64511, #99754 ) ;
#251257=EDGE_CURVE ( 'NONE', #94704, #174236, #76571, .T. ) ;
#251285=VERTEX_POINT ( 'NONE', #207548 ) ;
#251304=CARTESIAN_POINT ( 'NONE',  ( 20.84999999999998721, 11.75000000000000000, -33.50000000000000000 ) ) ;
#251327=VERTEX_POINT ( 'NONE', #28949 ) ;
#251347=CARTESIAN_POINT ( 'NONE',  ( 20.94999999999999929, 0.000000000000000000, -12.97499999999999787 ) ) ;
#251362=EDGE_CURVE ( 'NONE', #210246, #47156, #190559, .T. ) ;
#251368=CARTESIAN_POINT ( 'NONE',  ( 21.06280952165543496, 10.62713230060095171, -12.20405388677887260 ) ) ;
#251385=EDGE_CURVE ( 'NONE', #126780, #230477, #147409, .T. ) ;
#251386=DIRECTION ( 'NONE',  ( -1.000000000000000000, -0.000000000000000000, -0.000000000000000000 ) ) ;
#251409=VERTEX_POINT ( 'NONE', #15785 ) ;
#251431=AXIS2_PLACEMENT_3D ( 'NONE', #47584, #206677, #144111 ) ;
#251469=CARTESIAN_POINT ( 'NONE',  ( 18.42595409746870772, -9.499999812565054214, -6.999362351746812649 ) ) ;
#251541=ORIENTED_EDGE ( 'NONE', *, *, #148886, .F. ) ;
#251561=EDGE_CURVE ( 'NONE', #41617, #14945, #176729, .T. ) ;
#251570=DIRECTION ( 'NONE',  ( -1.000000000000000000, 0.000000000000000000, 0.000000000000000000 ) ) ;
#251597=CARTESIAN_POINT ( 'NONE',  ( 18.49999999999999289, 10.32573593128807232, -24.85000000000000142 ) ) ;
#251603=CARTESIAN_POINT ( 'NONE',  ( 18.59999999999999076, -1.149570369575693807, -41.31591248450196474 ) ) ;
#251604=CARTESIAN_POINT ( 'NONE',  ( 20.94999999999999929, 6.649999999999999467, -21.25000000000000000 ) ) ;
#251610=CARTESIAN_POINT ( 'NONE',  ( 22.50000000000000000, 0.09999999999999939493, 11.64957080754479968 ) ) ;
#251641=ORIENTED_EDGE ( 'NONE', *, *, #231159, .F. ) ;
#251669=DIRECTION ( 'NONE',  ( 0.000000000000000000, 0.000000000000000000, 1.000000000000000000 ) ) ;
#251670=DIRECTION ( 'NONE',  ( -1.000000000000000000, 0.000000000000000000, 0.000000000000000000 ) ) ;
#251684=DIRECTION ( 'NONE',  ( 1.000000000000000000, 0.000000000000000000, 0.000000000000000000 ) ) ;
#251706=CARTESIAN_POINT ( 'NONE',  ( -20.94999999999999929, 11.59999999999999609, -6.928203230275558511 ) ) ;
#251763=CARTESIAN_POINT ( 'NONE',  ( -21.14999999999999858, -0.1008583690987122083, 11.74956712348939192 ) ) ;
#251765=CIRCLE ( 'NONE', #1764, 0.09999999999999939493 ) ;
#251806=LINE ( 'NONE', #213975, #212741 ) ;
#251816=ORIENTED_EDGE ( 'NONE', *, *, #134385, .F. ) ;
#251834=AXIS2_PLACEMENT_3D ( 'NONE', #177325, #195591, #258061 ) ;
#251836=VERTEX_POINT ( 'NONE', #36305 ) ;
#251856=ORIENTED_EDGE ( 'NONE', *, *, #251561, .F. ) ;
#251893=ORIENTED_EDGE ( 'NONE', *, *, #214664, .T. ) ;
#251901=AXIS2_PLACEMENT_3D ( 'NONE', #138921, #181947, #200225 ) ;
#251902=AXIS2_PLACEMENT_3D ( 'NONE', #123525, #218754, #165215 ) ;
#251905=EDGE_CURVE ( 'NONE', #59419, #62255, #243525, .T. ) ;
#251912=EDGE_CURVE ( 'NONE', #7751, #158135, #202026, .T. ) ;
#251914=ORIENTED_EDGE ( 'NONE', *, *, #206602, .T. ) ;
#251926=DIRECTION ( 'NONE',  ( -1.000000000000000000, 0.000000000000000000, 0.000000000000000000 ) ) ;
#251931=VECTOR ( 'NONE', #121019, 999.9999999999998863 ) ;
#251943=CYLINDRICAL_SURFACE ( 'NONE', #90285, 0.09999999999999939493 ) ;
#251946=ORIENTED_EDGE ( 'NONE', *, *, #240865, .F. ) ;
#251976=CYLINDRICAL_SURFACE ( 'NONE', #39353, 0.09999999999999939493 ) ;
#251981=ADVANCED_FACE ( 'NONE', ( #40166 ), #247818, .T. ) ;
#251989=EDGE_LOOP ( 'NONE', ( #12727, #55811, #29160, #55768 ) ) ;
#252053=DIRECTION ( 'NONE',  ( 1.000000000000000000, 0.000000000000000000, 0.000000000000000000 ) ) ;
#252085=TOROIDAL_SURFACE ( 'NONE', #10673, 11.65000000000000036, 0.1000000000000000056 ) ;
#252094=CARTESIAN_POINT ( 'NONE',  ( -20.94999999999999929, 1.835341550224411922, -11.65515129256298010 ) ) ;
#252127=CARTESIAN_POINT ( 'NONE',  ( -20.54999999999999716, 2.449293598294709373E-16, -35.50000000000000711 ) ) ;
#252141=FACE_OUTER_BOUND ( 'NONE', #183908, .T. ) ;
#252155=ORIENTED_EDGE ( 'NONE', *, *, #77184, .F. ) ;
#252161=DIRECTION ( 'NONE',  ( 0.000000000000000000, 0.000000000000000000, 1.000000000000000000 ) ) ;
#252180=LINE ( 'NONE', #133530, #75264 ) ;
#252211=DIRECTION ( 'NONE',  ( 0.000000000000000000, 1.776356839400250465E-15, -1.000000000000000000 ) ) ;
#252229=CIRCLE ( 'NONE', #110592, 11.74999999999999645 ) ;
#252231=TOROIDAL_SURFACE ( 'NONE', #156433, 0.6000000000000015321, 0.1000000000000000056 ) ;
#252232=EDGE_CURVE ( 'NONE', #58239, #253517, #206308, .T. ) ;
#252249=EDGE_LOOP ( 'NONE', ( #139459, #255671 ) ) ;
#252260=CARTESIAN_POINT ( 'NONE',  ( 18.59999999999999076, 6.649999999999999467, -21.25000000000000000 ) ) ;
#252270=VERTEX_POINT ( 'NONE', #13852 ) ;
#252272=CARTESIAN_POINT ( 'NONE',  ( 18.60000000000000142, -9.399999999999938183, -7.297259759663296208 ) ) ;
#252288=DIRECTION ( 'NONE',  ( 1.000000000000000000, 0.000000000000000000, 0.000000000000000000 ) ) ;
#252331=FACE_OUTER_BOUND ( 'NONE', #191880, .T. ) ;
#252360=DIRECTION ( 'NONE',  ( 0.000000000000000000, 0.000000000000000000, -1.000000000000000000 ) ) ;
#252369=B_SPLINE_CURVE_WITH_KNOTS ( 'NONE', 3,
 ( #156464, #16926, #57298, #74358, #191733, #234678, #235948, #76874, #73078, #135560, #172188, #173480, #153911, #176013, #195571, #117302 ),
 .UNSPECIFIED., .F., .F.,
 ( 4, 3, 3, 3, 3, 4 ),
 ( 0.000000000000000000, 2.209075297430740031E-05, 5.594258369009624354E-05, 8.979524372342012487E-05, 0.0001236472815274586301, 0.0001574990747609554737 ),
 .UNSPECIFIED. ) ;
#252386=DIRECTION ( 'NONE',  ( 0.000000000000000000, 0.000000000000000000, -1.000000000000000000 ) ) ;
#252388=EDGE_CURVE ( 'NONE', #243103, #4098, #124508, .T. ) ;
#252404=DIRECTION ( 'NONE',  ( 0.000000000000000000, -1.000000000000000000, -1.734723475976807292E-15 ) ) ;
#252449=DIRECTION ( 'NONE',  ( 0.000000000000000000, 0.000000000000000000, 1.000000000000000000 ) ) ;
#252471=CARTESIAN_POINT ( 'NONE',  ( -23.15000000000000213, 0.000000000000000000, -20.62500000000000355 ) ) ;
#252473=DIRECTION ( 'NONE',  ( 2.259780016855445309E-14, 0.9875055080513753802, -0.1575844902526748192 ) ) ;
#252495=CIRCLE ( 'NONE', #160951, 0.09999999999999939493 ) ;
#252502=DIRECTION ( 'NONE',  ( -1.000000000000000000, 0.000000000000000000, 0.000000000000000000 ) ) ;
#252532=VERTEX_POINT ( 'NONE', #180197 ) ;
#252543=ORIENTED_EDGE ( 'NONE', *, *, #209944, .T. ) ;
#252558=CARTESIAN_POINT ( 'NONE',  ( -22.39999999999999858, 0.000000000000000000, 7.790779598373403836 ) ) ;
#252563=CIRCLE ( 'NONE', #131773, 0.09999999999999939493 ) ;
#252565=ORIENTED_EDGE ( 'NONE', *, *, #234230, .F. ) ;
#252593=CIRCLE ( 'NONE', #110962, 0.09999999999999982514 ) ;
#252621=CIRCLE ( 'NONE', #202741, 0.09999999999999761857 ) ;
#252643=EDGE_CURVE ( 'NONE', #71370, #240172, #163199, .T. ) ;
#252658=CIRCLE ( 'NONE', #61132, 0.09999999999999939493 ) ;
#252662=CARTESIAN_POINT ( 'NONE',  ( 21.05000000000000071, 5.499999999999998224, -12.40526601891309788 ) ) ;
#252683=CARTESIAN_POINT ( 'NONE',  ( 18.59999999999999787, -1.835341550224411922, -11.55515129256297868 ) ) ;
#252685=DIRECTION ( 'NONE',  ( 1.000000000000000000, 0.000000000000000000, 0.000000000000000000 ) ) ;
#252697=CARTESIAN_POINT ( 'NONE',  ( -18.43634282235122512, -9.679787199927979202, -40.16065188545389475 ) ) ;
#252709=EDGE_LOOP ( 'NONE', ( #161021, #134197, #86698 ) ) ;
#252721=( BOUNDED_SURFACE ( )  B_SPLINE_SURFACE ( 3, 2, ( 
 ( #28654, #145966, #188959 ),
 ( #29909, #186404, #106837 ),
 ( #108139, #187694, #109402 ),
 ( #144678, #10335, #27361 ),
 ( #5150, #7760, #224219 ),
 ( #104261, #89840, #9034 ) ),
 .UNSPECIFIED., .F., .F., .F. ) 
 B_SPLINE_SURFACE_WITH_KNOTS ( ( 4, 2, 4 ),
 ( 3, 3 ),
 ( 4.712388980384689674, 5.497787143782137953, 6.283185307179586232 ),
 ( 0.000000000000000000, 1.000000000000000000 ),
 .UNSPECIFIED. ) 
 GEOMETRIC_REPRESENTATION_ITEM ( )  RATIONAL_B_SPLINE_SURFACE ( (
 ( 1.000000000000000000, 0.7071067811865536790, 1.000000000000000000),
 ( 1.000000000000000000, 0.7727932973490582169, 1.000000000000000000),
 ( 1.000000000000000000, 0.8282379607650555142, 1.000000000000000000),
 ( 1.000000000000000000, 0.9038128468038272301, 1.000000000000000000),
 ( 1.000000000000000000, 0.9240297172244550383, 1.000000000000000000),
 ( 1.000000000000000000, 0.9238795325112914014, 1.000000000000000000) ) ) 
 REPRESENTATION_ITEM ( '' )  SURFACE ( )  );
#252730=CARTESIAN_POINT ( 'NONE',  ( 18.59999999999999076, 6.649999999999999467, -21.35000000000000142 ) ) ;
#252743=EDGE_CURVE ( 'NONE', #197300, #245627, #2464, .T. ) ;
#252759=CARTESIAN_POINT ( 'NONE',  ( 18.39999999999999858, -9.682403433476395094, -40.15684337741279109 ) ) ;
#252784=AXIS2_PLACEMENT_3D ( 'NONE', #81017, #160608, #61410 ) ;
#252827=ORIENTED_EDGE ( 'NONE', *, *, #159943, .T. ) ;
#252847=EDGE_CURVE ( 'NONE', #9216, #71227, #243891, .T. ) ;
#252866=ORIENTED_EDGE ( 'NONE', *, *, #28610, .F. ) ;
#252867=CARTESIAN_POINT ( 'NONE',  ( 21.05000000000000071, 8.776282895292474961, -8.558628995140949769 ) ) ;
#252916=CARTESIAN_POINT ( 'NONE',  ( -18.50000000000000000, 11.74999999999999645, 11.75000000000000000 ) ) ;
#252930=CARTESIAN_POINT ( 'NONE',  ( -20.54999999999999716, 0.000000000000000000, -35.40000000000000568 ) ) ;
#252936=DIRECTION ( 'NONE',  ( 1.000000000000000000, 0.000000000000000000, 0.000000000000000000 ) ) ;
#252938=DIRECTION ( 'NONE',  ( 1.836970198721029934E-16, -1.000000000000000000, -0.000000000000000000 ) ) ;
#252958=CIRCLE ( 'NONE', #136398, 0.09999999999999939493 ) ;
#252981=CIRCLE ( 'NONE', #148955, 0.09999999999999939493 ) ;
#252984=ORIENTED_EDGE ( 'NONE', *, *, #194278, .T. ) ;
#252992=CIRCLE ( 'NONE', #48982, 11.90000000000000391 ) ;
#253000=CARTESIAN_POINT ( 'NONE',  ( -22.50000000000000000, 11.75000000000000000, -3.469446951953614189E-15 ) ) ;
#253064=DIRECTION ( 'NONE',  ( 0.000000000000000000, 0.000000000000000000, -1.000000000000000000 ) ) ;
#253086=CARTESIAN_POINT ( 'NONE',  ( 23.15000000000000213, -11.64999999999999147, -30.39999999999999503 ) ) ;
#253089=CARTESIAN_POINT ( 'NONE',  ( 21.00000000000000000, 9.749999999999998224, -21.25000000000000000 ) ) ;
#253101=CARTESIAN_POINT ( 'NONE',  ( 20.95017935633852346, 10.47548927962532339, -7.577439797390487008 ) ) ;
#253137=ORIENTED_EDGE ( 'NONE', *, *, #90525, .F. ) ;
#253169=CIRCLE ( 'NONE', #240152, 0.09999999999999939493 ) ;
#253199=DIRECTION ( 'NONE',  ( 2.694716079187272946E-16, -1.000000000000000000, 0.000000000000000000 ) ) ;
#253201=AXIS2_PLACEMENT_3D ( 'NONE', #220131, #121057, #166597 ) ;
#253205=CARTESIAN_POINT ( 'NONE',  ( -23.25000000000000000, -9.682403433476396870, -40.15684337741279109 ) ) ;
#253206=DIRECTION ( 'NONE',  ( 0.000000000000000000, 1.000000000000000000, 0.000000000000000000 ) ) ;
#253210=DIRECTION ( 'NONE',  ( 1.000000000000000000, 2.952720810173289112E-16, -0.000000000000000000 ) ) ;
#253220=DIRECTION ( 'NONE',  ( 0.000000000000000000, 1.000000000000000000, 0.000000000000000000 ) ) ;
#253243=CARTESIAN_POINT ( 'NONE',  ( -18.39999999999999858, -9.400000000000005684, 11.75000000000000000 ) ) ;
#253276=LINE ( 'NONE', #249454, #50928 ) ;
#253286=DIRECTION ( 'NONE',  ( 0.000000000000000000, -1.265107689135680095E-16, 1.000000000000000000 ) ) ;
#253319=CARTESIAN_POINT ( 'NONE',  ( 22.48660254037843842, 11.74999999999999822, 0.04999999999999833744 ) ) ;
#253348=CARTESIAN_POINT ( 'NONE',  ( 23.25000000000000000, -11.65000000000000036, 3.469446951953614189E-15 ) ) ;
#253360=CARTESIAN_POINT ( 'NONE',  ( -20.85000000000000142, 7.021664781900089913, -37.33356540189728889 ) ) ;
#253366=VERTEX_POINT ( 'NONE', #29357 ) ;
#253376=ORIENTED_EDGE ( 'NONE', *, *, #7693, .F. ) ;
#253378=ADVANCED_FACE ( 'NONE', ( #106257 ), #104955, .F. ) ;
#253391=ORIENTED_EDGE ( 'NONE', *, *, #95806, .F. ) ;
#253392=CARTESIAN_POINT ( 'NONE',  ( -20.54999999999999716, -9.000000000000001776, -23.60603087734756045 ) ) ;
#253399=AXIS2_PLACEMENT_3D ( 'NONE', #150524, #26740, #188360 ) ;
#253415=DIRECTION ( 'NONE',  ( 0.7071067811865474617, 0.7071067811865474617, -0.000000000000000000 ) ) ;
#253426=AXIS2_PLACEMENT_3D ( 'NONE', #145414, #31924, #8494 ) ;
#253447=LINE ( 'NONE', #233895, #173611 ) ;
#253474=VERTEX_POINT ( 'NONE', #111423 ) ;
#253491=CIRCLE ( 'NONE', #7815, 3.999999999999996447 ) ;
#253500=CYLINDRICAL_SURFACE ( 'NONE', #195210, 0.09999999999999939493 ) ;
#253514=CIRCLE ( 'NONE', #161982, 0.09999999999999939493 ) ;
#253517=VERTEX_POINT ( 'NONE', #136087 ) ;
#253522=SURFACE_STYLE_FILL_AREA ( #250946 ) ;
#253551=LINE ( 'NONE', #240114, #13771 ) ;
#253573=DIRECTION ( 'NONE',  ( 1.000000000000000000, -0.000000000000000000, -0.000000000000000000 ) ) ;
#253582=CARTESIAN_POINT ( 'NONE',  ( -22.59999999999999787, 0.000000000000000000, 0.000000000000000000 ) ) ;
#253599=VERTEX_POINT ( 'NONE', #16196 ) ;
#253602=EDGE_CURVE ( 'NONE', #57106, #163009, #247796, .T. ) ;
#253620=CARTESIAN_POINT ( 'NONE',  ( 18.49999999999998934, 6.550000000000000711, -10.01702717044001822 ) ) ;
#253639=EDGE_CURVE ( 'NONE', #108803, #232204, #158290, .T. ) ;
#253695=DIRECTION ( 'NONE',  ( -1.000000000000000000, -2.952720810173289112E-16, 0.000000000000000000 ) ) ;
#253732=DIRECTION ( 'NONE',  ( 1.000000000000000000, 0.000000000000000000, 0.000000000000000000 ) ) ;
#253774=DIRECTION ( 'NONE',  ( 1.000000000000000000, -0.000000000000000000, -0.000000000000000000 ) ) ;
#253783=CARTESIAN_POINT ( 'NONE',  ( 21.05000000000000071, 4.999999999999997335, -21.09473398108690390 ) ) ;
#253822=EDGE_LOOP ( 'NONE', ( #4290, #226663, #149686, #247147 ) ) ;
#253885=DIRECTION ( 'NONE',  ( 0.000000000000000000, -1.000000000000000000, 0.000000000000000000 ) ) ;
#253898=DIRECTION ( 'NONE',  ( 1.000000000000000000, 3.265361837132813093E-16, -0.000000000000000000 ) ) ;
#253908=DIRECTION ( 'NONE',  ( 6.484947573744954877E-15, 0.9274965247785529332, -0.3738317757009255171 ) ) ;
#253944=CARTESIAN_POINT ( 'NONE',  ( 18.43709777086139567, -9.682403433476389765, -40.15684337741277687 ) ) ;
#253952=DIRECTION ( 'NONE',  ( -1.000000000000000000, -0.000000000000000000, -0.000000000000000000 ) ) ;
#254029=FACE_OUTER_BOUND ( 'NONE', #58616, .T. ) ;
#254031=CIRCLE ( 'NONE', #154135, 0.5000000000000004441 ) ;
#254057=DIRECTION ( 'NONE',  ( -1.000000000000000000, -0.000000000000000000, 0.000000000000000000 ) ) ;
#254059=DIRECTION ( 'NONE',  ( -1.000000000000000000, 0.000000000000000000, 0.000000000000000000 ) ) ;
#254078=CARTESIAN_POINT ( 'NONE',  ( 20.94999999999999574, 1.835341550224411922, -11.55515129256298046 ) ) ;
#254081=DIRECTION ( 'NONE',  ( 1.000000000000000000, 0.000000000000000000, 0.000000000000000000 ) ) ;
#254082=DIRECTION ( 'NONE',  ( -1.000000000000000000, -0.000000000000000000, -0.000000000000000000 ) ) ;
#254102=EDGE_CURVE ( 'NONE', #41617, #8661, #244052, .T. ) ;
#254123=ORIENTED_EDGE ( 'NONE', *, *, #182302, .T. ) ;
#254138=LINE ( 'NONE', #98895, #102801 ) ;
#254143=EDGE_LOOP ( 'NONE', ( #144353, #20958, #30826, #103713 ) ) ;
#254164=CARTESIAN_POINT ( 'NONE',  ( -20.64999999999999858, 0.000000000000000000, -33.50000000000000000 ) ) ;
#254197=ADVANCED_FACE ( 'NONE', ( #247747 ), #147365, .T. ) ;
#254211=CARTESIAN_POINT ( 'NONE',  ( -20.54999999999999716, 7.150000000000000355, -21.15000000000000213 ) ) ;
#254235=ORIENTED_EDGE ( 'NONE', *, *, #27157, .T. ) ;
#254254=CARTESIAN_POINT ( 'NONE',  ( -21.05000000000000071, 11.64999999999999680, -6.783865662978151967 ) ) ;
#254257=CIRCLE ( 'NONE', #87665, 0.09999999999999939493 ) ;
#254268=ORIENTED_EDGE ( 'NONE', *, *, #199870, .F. ) ;
#254269=CARTESIAN_POINT ( 'NONE',  ( 20.94999999999999574, 1.851028230140860487, -11.65391326942249250 ) ) ;
#254299=DIRECTION ( 'NONE',  ( 0.000000000000000000, 0.5000000000000209832, 0.8660254037844264952 ) ) ;
#254303=CIRCLE ( 'NONE', #66879, 3.999999999999999112 ) ;
#254325=VERTEX_POINT ( 'NONE', #135482 ) ;
#254328=DIRECTION ( 'NONE',  ( -0.000000000000000000, 1.000000000000000000, 0.000000000000000000 ) ) ;
#254351=CIRCLE ( 'NONE', #229435, 0.1000000000000028644 ) ;
#254354=DIRECTION ( 'NONE',  ( 1.000000000000000000, 0.000000000000000000, 0.000000000000000000 ) ) ;
#254372=DIRECTION ( 'NONE',  ( -1.000000000000000000, -0.000000000000000000, -0.000000000000000000 ) ) ;
#254373=CARTESIAN_POINT ( 'NONE',  ( 20.95496329884391784, 10.56743320609303716, -7.574309932284823965 ) ) ;
#254385=CARTESIAN_POINT ( 'NONE',  ( 20.94999999999999929, -9.500000000000000000, -23.60603087734755690 ) ) ;
#254387=CARTESIAN_POINT ( 'NONE',  ( -23.25000000000000000, -1.736705739467587772, -45.01742258762372728 ) ) ;
#254417=AXIS2_PLACEMENT_3D ( 'NONE', #208079, #149397, #13703 ) ;
#254471=DIRECTION ( 'NONE',  ( 1.000000000000000000, -0.000000000000000000, -0.000000000000000000 ) ) ;
#254476=CONICAL_SURFACE ( 'NONE', #409, 4.049999999999998934, 0.7853981633974604915 ) ;
#254498=DIRECTION ( 'NONE',  ( 0.000000000000000000, 0.1568667991644863147, -0.9876197685951252359 ) ) ;
#254504=ADVANCED_FACE ( 'NONE', ( #47604 ), #127168, .F. ) ;
#254557=VECTOR ( 'NONE', #232766, 1000.000000000000000 ) ;
#254565=LINE ( 'NONE', #75964, #165127 ) ;
#254567=DIRECTION ( 'NONE',  ( -1.000000000000000000, 7.304098846218135653E-16, -4.607487905232624742E-31 ) ) ;
#254570=DIRECTION ( 'NONE',  ( -3.469446951953605354E-14, -0.9999176327611372095, -0.01283462868039623485 ) ) ;
#254608=CIRCLE ( 'NONE', #142196, 0.1000000000000028644 ) ;
#254611=CARTESIAN_POINT ( 'NONE',  ( -23.25000000000000000, -1.164121893241208960, -41.41484808557160591 ) ) ;
#254624=ORIENTED_EDGE ( 'NONE', *, *, #247089, .F. ) ;
#254646=ADVANCED_FACE ( 'NONE', ( #17483 ), #106867, .F. ) ;
#254659=DIRECTION ( 'NONE',  ( 1.000000000000000000, 0.000000000000000000, 0.000000000000000000 ) ) ;
#254673=CARTESIAN_POINT ( 'NONE',  ( 23.24999999999999289, 6.450000000000001066, -21.15000000000000213 ) ) ;
#254685=ORIENTED_EDGE ( 'NONE', *, *, #54576, .F. ) ;
#254705=LINE ( 'NONE', #173987, #65674 ) ;
#254713=LINE ( 'NONE', #134791, #104436 ) ;
#254727=ORIENTED_EDGE ( 'NONE', *, *, #107950, .T. ) ;
#254745=AXIS2_PLACEMENT_3D ( 'NONE', #48486, #125473, #65481 ) ;
#254750=CARTESIAN_POINT ( 'NONE',  ( -21.14999999999999858, 11.75000000000000000, -6.783865662978153743 ) ) ;
#254758=AXIS2_PLACEMENT_3D ( 'NONE', #53901, #235114, #16088 ) ;
#254821=DIRECTION ( 'NONE',  ( -0.000000000000000000, -0.000000000000000000, 1.000000000000000000 ) ) ;
#254825=DIRECTION ( 'NONE',  ( 0.000000000000000000, 0.000000000000000000, -1.000000000000000000 ) ) ;
#254828=ADVANCED_FACE ( 'NONE', ( #129429 ), #251943, .T. ) ;
#254849=ORIENTED_EDGE ( 'NONE', *, *, #7214, .F. ) ;
#254869=ORIENTED_EDGE ( 'NONE', *, *, #41955, .F. ) ;
#254899=EDGE_LOOP ( 'NONE', ( #105627, #214585 ) ) ;
#254941=ORIENTED_EDGE ( 'NONE', *, *, #111360, .T. ) ;
#254987=DIRECTION ( 'NONE',  ( 0.000000000000000000, 0.1575844902526727098, 0.9875055080513754913 ) ) ;
#255002=LINE ( 'NONE', #37327, #164759 ) ;
#255016=AXIS2_PLACEMENT_3D ( 'NONE', #52246, #191813, #129245 ) ;
#255031=PLANE ( 'NONE',  #40095 ) ;
#255042=VERTEX_POINT ( 'NONE', #40650 ) ;
#255052=CARTESIAN_POINT ( 'NONE',  ( 20.95224633520496127, 8.900522166557230719, -8.493276447921262573 ) ) ;
#255058=EDGE_CURVE ( 'NONE', #238460, #52704, #99273, .T. ) ;
#255065=ORIENTED_EDGE ( 'NONE', *, *, #61792, .T. ) ;
#255077=B_SPLINE_CURVE_WITH_KNOTS ( 'NONE', 3,
 ( #45180, #3478, #24360, #163856, #124730, #243377, #144256 ),
 .UNSPECIFIED., .F., .F.,
 ( 4, 3, 4 ),
 ( 5.692061405548898279E-19, 3.357501770814694990E-05, 5.199112466349232217E-05 ),
 .UNSPECIFIED. ) ;
#255118=ORIENTED_EDGE ( 'NONE', *, *, #23992, .T. ) ;
#255135=ORIENTED_EDGE ( 'NONE', *, *, #104664, .T. ) ;
#255176=AXIS2_PLACEMENT_3D ( 'NONE', #211069, #92389, #171982 ) ;
#255185=CARTESIAN_POINT ( 'NONE',  ( 18.59999999999999432, -9.480686695278969012, -40.44111516875785384 ) ) ;
#255256=DIRECTION ( 'NONE',  ( 0.000000000000000000, 0.000000000000000000, 1.000000000000000000 ) ) ;
#255263=EDGE_LOOP ( 'NONE', ( #50761, #222330, #173172, #192891 ) ) ;
#255296=ADVANCED_FACE ( 'NONE', ( #93847 ), #110844, .F. ) ;
#255303=VERTEX_POINT ( 'NONE', #53446 ) ;
#255379=DIRECTION ( 'NONE',  ( 0.000000000000000000, -1.000000000000000000, 0.000000000000000000 ) ) ;
#255385=CARTESIAN_POINT ( 'NONE',  ( 19.75857864376268935, 11.65000000000000391, -24.75000000000000000 ) ) ;
#255403=CIRCLE ( 'NONE', #176369, 0.09999999999999892308 ) ;
#255429=TOROIDAL_SURFACE ( 'NONE', #130566, 0.6000000000000004219, 0.1000000000000000056 ) ;
#255445=ORIENTED_EDGE ( 'NONE', *, *, #29671, .F. ) ;
#255460=VERTEX_POINT ( 'NONE', #225326 ) ;
#255465=FACE_OUTER_BOUND ( 'NONE', #167564, .T. ) ;
#255475=DIRECTION ( 'NONE',  ( -1.000000000000000000, -0.000000000000000000, 0.000000000000000000 ) ) ;
#255496=CARTESIAN_POINT ( 'NONE',  ( 18.59999999999999432, 10.49142135623730887, -24.75000000000000000 ) ) ;
#255497=DIRECTION ( 'NONE',  ( 0.000000000000000000, 0.000000000000000000, -1.000000000000000000 ) ) ;
#255523=ADVANCED_FACE ( 'NONE', ( #239791 ), #106664, .T. ) ;
#255530=CARTESIAN_POINT ( 'NONE',  ( 21.14999999999999858, 11.75000000000000711, -0.1000000000000028644 ) ) ;
#255533=VERTEX_POINT ( 'NONE', #104095 ) ;
#255579=CARTESIAN_POINT ( 'NONE',  ( 21.05000000000000071, 0.000000000000000000, -33.50000000000000000 ) ) ;
#255581=AXIS2_PLACEMENT_3D ( 'NONE', #79606, #139575, #255648 ) ;
#255617=DIRECTION ( 'NONE',  ( 1.000000000000000000, 3.265361837132813093E-16, -0.000000000000000000 ) ) ;
#255648=DIRECTION ( 'NONE',  ( 0.000000000000000000, 0.000000000000000000, -1.000000000000000000 ) ) ;
#255669=DIRECTION ( 'NONE',  ( 0.000000000000000000, 0.000000000000000000, -1.000000000000000000 ) ) ;
#255671=ORIENTED_EDGE ( 'NONE', *, *, #109787, .T. ) ;
#255716=AXIS2_PLACEMENT_3D ( 'NONE', #69376, #90181, #169782 ) ;
#255776=CARTESIAN_POINT ( 'NONE',  ( 21.14999999999999503, -11.64999999999999147, 11.75000000000000000 ) ) ;
#255792=( BOUNDED_SURFACE ( )  B_SPLINE_SURFACE ( 3, 2, ( 
 ( #142591, #82599, #64369 ),
 ( #241714, #181743, #223416 ),
 ( #100868, #22694, #164751 ),
 ( #26535, #203862, #25254 ),
 ( #222117, #240433, #141330 ),
 ( #220857, #43525, #104731 ) ),
 .UNSPECIFIED., .F., .F., .F. ) 
 B_SPLINE_SURFACE_WITH_KNOTS ( ( 4, 2, 4 ),
 ( 3, 3 ),
 ( 1.570796326794897668, 2.356194490192346169, 3.141592653589794448 ),
 ( 0.000000000000000000, 1.000000000000000000 ),
 .UNSPECIFIED. ) 
 GEOMETRIC_REPRESENTATION_ITEM ( )  RATIONAL_B_SPLINE_SURFACE ( (
 ( 1.000000000000000000, 0.7071067811865536790, 1.000000000000000000),
 ( 1.000000000000000000, 0.6611148371784283384, 1.000000000000000000),
 ( 1.000000000000000000, 0.6092287576688637518, 1.000000000000000000),
 ( 1.000000000000000000, 0.5278258667065212073, 1.000000000000000000),
 ( 1.000000000000000000, 0.4993418825328512778, 1.000000000000000000),
 ( 1.000000000000000000, 0.4999999999999970024, 1.000000000000000000) ) ) 
 REPRESENTATION_ITEM ( '' )  SURFACE ( )  );
#255800=AXIS2_PLACEMENT_3D ( 'NONE', #150767, #186044, #67378 ) ;
#255811=CARTESIAN_POINT ( 'NONE',  ( -20.64999999999999858, 1.940186915887853303, -12.82911921105332631 ) ) ;
#255829=AXIS2_PLACEMENT_3D ( 'NONE', #13141, #92657, #245328 ) ;
#255862=ORIENTED_EDGE ( 'NONE', *, *, #194523, .F. ) ;
#255879=EDGE_LOOP ( 'NONE', ( #128299, #26414, #51662, #93430, #103918, #159172, #168190, #19601, #227304, #64958, #39423, #87127 ) ) ;
#255926=CARTESIAN_POINT ( 'NONE',  ( -18.59999999999999787, 9.350000000000001421, -21.15000000000000213 ) ) ;
#255937=DIRECTION ( 'NONE',  ( 0.000000000000000000, 0.000000000000000000, -1.000000000000000000 ) ) ;
#255949=AXIS2_PLACEMENT_3D ( 'NONE', #140499, #223885, #124812 ) ;
#255988=CIRCLE ( 'NONE', #72925, 0.09999999999999971412 ) ;
#255991=LINE ( 'NONE', #137368, #87866 ) ;
#255999=CYLINDRICAL_SURFACE ( 'NONE', #68048, 0.09999999999999939493 ) ;
#256007=CARTESIAN_POINT ( 'NONE',  ( -18.59999999999999787, 11.64999999999999680, -12.14999999999999680 ) ) ;
#256032=AXIS2_PLACEMENT_3D ( 'NONE', #114982, #194551, #175007 ) ;
#256053=DIRECTION ( 'NONE',  ( 0.000000000000000000, 0.000000000000000000, 1.000000000000000000 ) ) ;
#256064=DIRECTION ( 'NONE',  ( 0.000000000000000000, 0.000000000000000000, -1.000000000000000000 ) ) ;
#256082=ORIENTED_EDGE ( 'NONE', *, *, #131545, .T. ) ;
#256094=CARTESIAN_POINT ( 'NONE',  ( -22.57848426163147693, -0.004264329283117146777, 11.75005830689033282 ) ) ;
#256157=EDGE_CURVE ( 'NONE', #243786, #5738, #80224, .T. ) ;
#256178=DIRECTION ( 'NONE',  ( -1.000000000000000000, 0.000000000000000000, 0.000000000000000000 ) ) ;
#256183=AXIS2_PLACEMENT_3D ( 'NONE', #250340, #69161, #194250 ) ;
#256219=ORIENTED_EDGE ( 'NONE', *, *, #89948, .F. ) ;
#256222=CARTESIAN_POINT ( 'NONE',  ( 21.14999999999999858, 6.540656951701244282, -0.09999999999999939493 ) ) ;
#256228=DIRECTION ( 'NONE',  ( 1.000000000000000000, -0.000000000000000000, -0.000000000000000000 ) ) ;
#256234=AXIS2_PLACEMENT_3D ( 'NONE', #149534, #226449, #165218 ) ;
#256239=AXIS2_PLACEMENT_3D ( 'NONE', #138317, #39275, #118796 ) ;
#256245=VERTEX_POINT ( 'NONE', #75499 ) ;
#256287=DIRECTION ( 'NONE',  ( 0.000000000000000000, 1.214306433183772287E-13, 1.000000000000000000 ) ) ;
#256307=CARTESIAN_POINT ( 'NONE',  ( 21.04999999999998650, 6.649999999999999467, -12.25000000000000000 ) ) ;
#256309=ADVANCED_FACE ( 'NONE', ( #214976 ), #112049, .T. ) ;
#256348=CARTESIAN_POINT ( 'NONE',  ( -18.43569575749026512, -9.519327731092442235, -6.972976376559330447 ) ) ;
#256381=VERTEX_POINT ( 'NONE', #14241 ) ;
#256415=EDGE_LOOP ( 'NONE', ( #78268, #158257, #160018, #190971 ) ) ;
#256445=CARTESIAN_POINT ( 'NONE',  ( -23.25000000000000000, 11.65000000000000036, 11.75000000000000000 ) ) ;
#256462=AXIS2_PLACEMENT_3D ( 'NONE', #174863, #155282, #215219 ) ;
#256465=FACE_OUTER_BOUND ( 'NONE', #35675, .T. ) ;
#256475=ADVANCED_FACE ( 'NONE', ( #181005, #78027 ), #177173, .T. ) ;
#256521=EDGE_CURVE ( 'NONE', #210246, #237621, #172273, .T. ) ;
#256525=CARTESIAN_POINT ( 'NONE',  ( -20.94999999999999929, 1.835341550224411922, -11.55515129256298046 ) ) ;
#256549=EDGE_CURVE ( 'NONE', #168114, #105990, #14217, .T. ) ;
#256550=CARTESIAN_POINT ( 'NONE',  ( -18.50000000000000000, 11.74999999999999645, -0.1000000000000028644 ) ) ;
#256552=DIRECTION ( 'NONE',  ( -2.915501640297154283E-16, 1.000000000000000000, 0.000000000000000000 ) ) ;
#256576=CARTESIAN_POINT ( 'NONE',  ( 20.94999999999999929, -9.000000000000000000, -23.60603087734755690 ) ) ;
#256605=VECTOR ( 'NONE', #61411, 1000.000000000000000 ) ;
#256614=DIRECTION ( 'NONE',  ( 0.000000000000000000, -1.000000000000000000, 0.000000000000000000 ) ) ;
#256624=VERTEX_POINT ( 'NONE', #89888 ) ;
#256663=VERTEX_POINT ( 'NONE', #191608 ) ;
#256685=CARTESIAN_POINT ( 'NONE',  ( 20.94999999999999929, 2.449293598294709866E-16, -31.50000000000000000 ) ) ;
#256700=DIRECTION ( 'NONE',  ( 1.000000000000000000, 7.304098846218133681E-16, -4.217023435051677501E-16 ) ) ;
#256703=CARTESIAN_POINT ( 'NONE',  ( -23.15000000000000213, -9.000000000000003553, -9.893969122652444881 ) ) ;
#256711=DIRECTION ( 'NONE',  ( 0.000000000000000000, -0.8660254037844383745, 0.5000000000000003331 ) ) ;
#256712=VECTOR ( 'NONE', #67134, 1000.000000000000000 ) ;
#256713=LINE ( 'NONE', #78114, #137009 ) ;
#256731=AXIS2_PLACEMENT_3D ( 'NONE', #251604, #131655, #112116 ) ;
#256736=DIRECTION ( 'NONE',  ( -3.469446951953635015E-14, 1.000000000000000000, 0.000000000000000000 ) ) ;
#256740=EDGE_LOOP ( 'NONE', ( #120094, #131175, #26807, #176536 ) ) ;
#256742=DIRECTION ( 'NONE',  ( 0.000000000000000000, 0.8660254037844352659, -0.5000000000000058842 ) ) ;
#256743=AXIS2_PLACEMENT_3D ( 'NONE', #62053, #219820, #196404 ) ;
#256778=FACE_OUTER_BOUND ( 'NONE', #228885, .T. ) ;
#256780=ORIENTED_EDGE ( 'NONE', *, *, #53486, .F. ) ;
#256788=ORIENTED_EDGE ( 'NONE', *, *, #222745, .F. ) ;
#256827=CARTESIAN_POINT ( 'NONE',  ( 23.15000000000000213, -9.000000000000000000, -23.60603087734755690 ) ) ;
#256833=EDGE_CURVE ( 'NONE', #56467, #243852, #163991, .T. ) ;
#256843=CARTESIAN_POINT ( 'NONE',  ( -23.15000000000000213, -11.75000000000000000, 3.469446951953614189E-15 ) ) ;
#256849=DIRECTION ( 'NONE',  ( 0.000000000000000000, 1.000000000000000000, -0.000000000000000000 ) ) ;
#256853=ORIENTED_EDGE ( 'NONE', *, *, #14460, .T. ) ;
#256857=CIRCLE ( 'NONE', #32077, 0.1000000000000028644 ) ;
#256879=EDGE_CURVE ( 'NONE', #127472, #222808, #93288, .T. ) ;
#256913=ADVANCED_FACE ( 'NONE', ( #144402 ), #164006, .F. ) ;
#256965=ORIENTED_EDGE ( 'NONE', *, *, #120353, .T. ) ;
#256966=DIRECTION ( 'NONE',  ( 1.000000000000000000, 0.000000000000000000, 0.000000000000000000 ) ) ;
#256984=PLANE ( 'NONE',  #34225 ) ;
#256996=DIRECTION ( 'NONE',  ( 0.000000000000000000, 0.000000000000000000, -1.000000000000000000 ) ) ;
#257000=PRODUCT_DEFINITION_FORMATION_WITH_SPECIFIED_SOURCE ( 'ANY', '', #203297, .NOT_KNOWN. ) ;
#257010=DIRECTION ( 'NONE',  ( 1.000000000000000000, -0.000000000000000000, -0.000000000000000000 ) ) ;
#257016=DIRECTION ( 'NONE',  ( 0.000000000000000000, 2.168404344971003346E-15, -1.000000000000000000 ) ) ;
#257020=DIRECTION ( 'NONE',  ( 0.000000000000000000, -1.000000000000000000, -0.000000000000000000 ) ) ;
#257029=ORIENTED_EDGE ( 'NONE', *, *, #60971, .T. ) ;
#257063=DIRECTION ( 'NONE',  ( 1.000000000000000000, 0.000000000000000000, 0.000000000000000000 ) ) ;
#257067=AXIS2_PLACEMENT_3D ( 'NONE', #159881, #221102, #42470 ) ;
#257091=EDGE_CURVE ( 'NONE', #239961, #5222, #47659, .T. ) ;
#257104=ADVANCED_FACE ( 'NONE', ( #92159 ), #155861, .F. ) ;
#257106=CARTESIAN_POINT ( 'NONE',  ( -23.15000000000000213, 11.75000000000000000, -21.34999999999999787 ) ) ;
#257113=FACE_OUTER_BOUND ( 'NONE', #245165, .T. ) ;
#257117=CARTESIAN_POINT ( 'NONE',  ( 21.03670563405601968, 10.62482368932824173, -12.32554688620915151 ) ) ;
#257143=CARTESIAN_POINT ( 'NONE',  ( -18.49513951962167013, -9.437725026677698636, -40.27807257502914240 ) ) ;
#257190=EDGE_LOOP ( 'NONE', ( #230264, #79666, #226278, #218184 ) ) ;
#257193=CIRCLE ( 'NONE', #90245, 11.80000000000000426 ) ;
#257201=EDGE_LOOP ( 'NONE', ( #147850, #178308, #36296, #63122 ) ) ;
#257213=DIRECTION ( 'NONE',  ( 0.000000000000000000, 0.000000000000000000, -1.000000000000000000 ) ) ;
#257221=FACE_OUTER_BOUND ( 'NONE', #79365, .T. ) ;
#257228=VERTEX_POINT ( 'NONE', #38615 ) ;
#257230=CARTESIAN_POINT ( 'NONE',  ( -1.820710678118657944, -9.929289321881341834, -24.75000000000000000 ) ) ;
#257235=CARTESIAN_POINT ( 'NONE',  ( 22.47071067811865319, 0.09909245470260570621, 7.720074744498046648 ) ) ;
#257293=EDGE_CURVE ( 'NONE', #52704, #109, #214101, .T. ) ;
#257351=VECTOR ( 'NONE', #206582, 1000.000000000000000 ) ;
#257354=CARTESIAN_POINT ( 'NONE',  ( -21.52071067811865746, 7.779289321881349473, -21.15000000000000213 ) ) ;
#257368=AXIS2_PLACEMENT_3D ( 'NONE', #134546, #135835, #2746 ) ;
#257380=ORIENTED_EDGE ( 'NONE', *, *, #223329, .F. ) ;
#257459=LINE ( 'NONE', #161001, #165405 ) ;
#257471=DIRECTION ( 'NONE',  ( -0.000000000000000000, 1.000000000000000000, -1.224646799147352961E-16 ) ) ;
#257473=DIRECTION ( 'NONE',  ( -1.000000000000000000, 0.000000000000000000, 0.000000000000000000 ) ) ;
#257492=EDGE_CURVE ( 'NONE', #47066, #39469, #106107, .T. ) ;
#257495=ORIENTED_EDGE ( 'NONE', *, *, #184169, .F. ) ;
#257502=SPHERICAL_SURFACE ( 'NONE', #144688, 0.1000000000000000056 ) ;
#257516=CIRCLE ( 'NONE', #78502, 12.87499999999999822 ) ;
#257538=VERTEX_POINT ( 'NONE', #54952 ) ;
#257546=DIRECTION ( 'NONE',  ( 0.000000000000000000, 3.469446951953635015E-14, 1.000000000000000000 ) ) ;
#257559=CARTESIAN_POINT ( 'NONE',  ( 21.30000000000002558, 0.000000000000000000, 0.000000000000000000 ) ) ;
#257570=DIRECTION ( 'NONE',  ( 0.000000000000000000, -1.000000000000000000, 3.469446951953614189E-14 ) ) ;
#257598=DIRECTION ( 'NONE',  ( 0.000000000000000000, 0.000000000000000000, 1.000000000000000000 ) ) ;
#257621=CARTESIAN_POINT ( 'NONE',  ( 20.95346350065193519, 8.887177249174493809, -8.511731947035384493 ) ) ;
#257636=DIRECTION ( 'NONE',  ( -1.000000000000000000, 0.000000000000000000, 0.000000000000000000 ) ) ;
#257641=DIRECTION ( 'NONE',  ( 0.000000000000000000, 0.4999999999999929501, 0.8660254037844427044 ) ) ;
#257681=ORIENTED_EDGE ( 'NONE', *, *, #39522, .T. ) ;
#257759=AXIS2_PLACEMENT_3D ( 'NONE', #187501, #88348, #85769 ) ;
#257764=EDGE_CURVE ( 'NONE', #44201, #49525, #201999, .T. ) ;
#257768=EDGE_CURVE ( 'NONE', #143460, #128093, #193803, .T. ) ;
#257779=EDGE_CURVE ( 'NONE', #161574, #253517, #93784, .T. ) ;
#257793=ADVANCED_FACE ( 'NONE', ( #38975 ), #234586, .F. ) ;
#257893=ORIENTED_EDGE ( 'NONE', *, *, #154338, .F. ) ;
#257908=DIRECTION ( 'NONE',  ( 0.000000000000000000, 0.000000000000000000, -1.000000000000000000 ) ) ;
#257920=CARTESIAN_POINT ( 'NONE',  ( -21.07928932188134041, 0.09889514565439468108, 6.328516656393293083 ) ) ;
#257937=ORIENTED_EDGE ( 'NONE', *, *, #106095, .T. ) ;
#257942=ORIENTED_EDGE ( 'NONE', *, *, #205044, .T. ) ;
#257947=ORIENTED_EDGE ( 'NONE', *, *, #12690, .T. ) ;
#257960=EDGE_LOOP ( 'NONE', ( #98467, #4075, #145702, #5121 ) ) ;
#257979=CIRCLE ( 'NONE', #183033, 3.900000000000000799 ) ;
#258009=CARTESIAN_POINT ( 'NONE',  ( 20.54374330479337374, 10.50501031422304798, -7.725683634888938833 ) ) ;
#258018=CARTESIAN_POINT ( 'NONE',  ( 21.05000000000000071, 6.540656951701244282, -0.09999999999999939493 ) ) ;
#258039=CARTESIAN_POINT ( 'NONE',  ( 21.05000000000000071, 11.65000000000000746, -26.48519422934605316 ) ) ;
#258046=CIRCLE ( 'NONE', #120743, 4.299999999999956302 ) ;
#258061=DIRECTION ( 'NONE',  ( 0.000000000000000000, 0.000000000000000000, -1.000000000000000000 ) ) ;
#258068=CARTESIAN_POINT ( 'NONE',  ( 18.49999999999999289, 10.41716543471636136, -24.84999999941982551 ) ) ;
#258084=VECTOR ( 'NONE', #34685, 1000.000000000000114 ) ;
#258087=AXIS2_PLACEMENT_3D ( 'NONE', #165403, #109255, #87124 ) ;
#258091=DIRECTION ( 'NONE',  ( -1.000000000000000000, -2.952720810173289112E-16, 0.000000000000000000 ) ) ;
#258096=DIRECTION ( 'NONE',  ( 0.000000000000000000, 0.000000000000000000, -1.000000000000000000 ) ) ;
#258097=DIRECTION ( 'NONE',  ( 1.000000000000000000, 0.000000000000000000, 0.000000000000000000 ) ) ;
ENDSEC;
END-ISO-10303-21;
